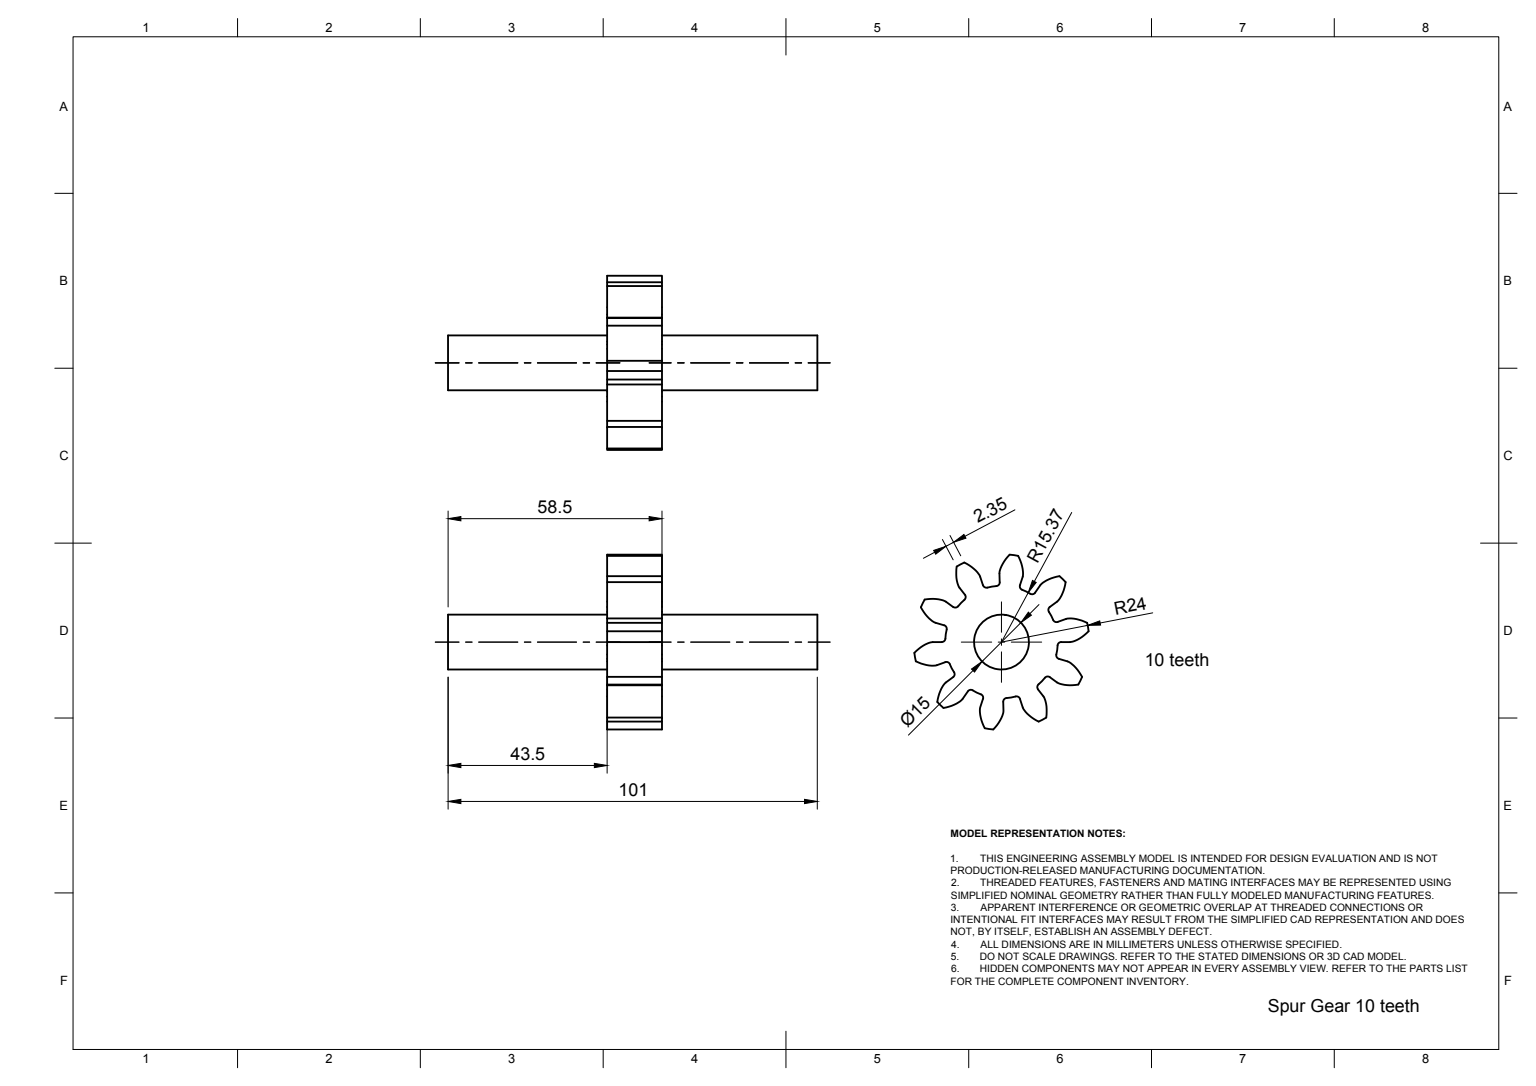
ISO-10303-21;
HEADER;
/* Generated by software containing ST-Developer
 * from STEP Tools, Inc. (www.steptools.com) 
 */

FILE_DESCRIPTION(
/* description */ (''),
/* implementation_level */ '2;1');

FILE_NAME(
/* name */ 'Spur Gear 10 teeth.step',
/* time_stamp */ '2026-10-05T21:54:13-07:00',
/* author */ (''),
/* organization */ (''),
/* preprocessor_version */ 'ST-DEVELOPER v20.2',
/* originating_system */ 'Autodesk Translation Framework v15.15.0.0',
/* authorisation */ '');

FILE_SCHEMA (('AUTOMOTIVE_DESIGN { 1 0 10303 214 3 1 1 }'));
ENDSEC;

DATA;
#10=MECHANICAL_DESIGN_GEOMETRIC_PRESENTATION_REPRESENTATION('',(#192),#43781);
#176=SHAPE_REPRESENTATION_RELATIONSHIP('SRR','None',#43814,#184);
#184=ADVANCED_BREP_SHAPE_REPRESENTATION('',(#236),#43774);
#192=STYLED_ITEM('',(#43862),#236);
#236=MANIFOLD_SOLID_BREP('Body1',#13052);
#281=FACE_BOUND('',#2275,.T.);
#282=FACE_BOUND('',#2277,.T.);
#571=B_SPLINE_CURVE_WITH_KNOTS('',5,(#32053,#32054,#32055,#32056,#32057,
#32058,#32059,#32060,#32061,#32062,#32063,#32064,#32065,#32066,#32067,#32068,
#32069,#32070,#32071,#32072,#32073,#32074,#32075,#32076,#32077,#32078,#32079,
#32080,#32081,#32082,#32083,#32084,#32085,#32086,#32087,#32088,#32089,#32090,
#32091,#32092,#32093,#32094,#32095,#32096,#32097,#32098,#32099,#32100,#32101,
#32102,#32103,#32104,#32105,#32106,#32107,#32108,#32109,#32110,#32111,#32112,
#32113,#32114,#32115,#32116,#32117,#32118,#32119,#32120,#32121,#32122,#32123,
#32124,#32125,#32126),.UNSPECIFIED.,.F.,.F.,(6,1,1,1,1,1,1,1,1,1,1,1,1,
1,1,1,1,1,1,1,1,1,1,1,1,1,1,1,1,1,1,1,1,1,1,1,1,1,1,1,1,1,1,1,1,1,1,1,1,
1,1,1,1,1,1,1,1,1,1,1,1,1,1,1,1,1,1,1,1,6),(0.,0.0142857142857143,0.0285714285714286,
0.0428571428571429,0.0571428571428571,0.0714285714285714,0.0857142857142857,
0.1,0.114285714285714,0.128571428571429,0.142857142857143,0.157142857142857,
0.171428571428571,0.185714285714286,0.2,0.214285714285714,0.228571428571429,
0.242857142857143,0.257142857142857,0.271428571428571,0.285714285714286,
0.3,0.314285714285714,0.328571428571429,0.342857142857143,0.357142857142857,
0.371428571428571,0.385714285714286,0.4,0.414285714285714,0.428571428571429,
0.442857142857143,0.457142857142857,0.471428571428572,0.485714285714286,
0.5,0.514285714285714,0.528571428571429,0.542857142857143,0.557142857142857,
0.571428571428571,0.585714285714286,0.6,0.614285714285714,0.628571428571428,
0.642857142857142,0.657142857142857,0.671428571428571,0.685714285714285,
0.699999999999999,0.714285714285714,0.728571428571428,0.742857142857142,
0.757142857142856,0.771428571428571,0.785714285714285,0.799999999999999,
0.814285714285713,0.828571428571428,0.842857142857142,0.857142857142856,
0.87142857142857,0.885714285714284,0.899999999999999,0.914285714285713,
0.928571428571427,0.942857142857141,0.957142857142856,0.97142857142857,
1.),.UNSPECIFIED.);
#572=B_SPLINE_CURVE_WITH_KNOTS('',5,(#32128,#32129,#32130,#32131,#32132,
#32133,#32134,#32135,#32136,#32137,#32138,#32139,#32140,#32141,#32142,#32143,
#32144,#32145,#32146,#32147,#32148,#32149,#32150,#32151,#32152,#32153,#32154,
#32155,#32156,#32157,#32158,#32159,#32160,#32161,#32162,#32163,#32164,#32165,
#32166,#32167,#32168,#32169,#32170,#32171,#32172,#32173,#32174,#32175,#32176,
#32177,#32178,#32179,#32180,#32181,#32182,#32183,#32184,#32185,#32186,#32187,
#32188,#32189,#32190,#32191,#32192,#32193,#32194,#32195,#32196,#32197,#32198,
#32199,#32200,#32201,#32202),.UNSPECIFIED.,.F.,.F.,(6,1,1,1,1,1,1,1,1,1,
1,1,1,1,1,1,1,1,1,1,1,1,1,1,1,1,1,1,1,1,1,1,1,1,1,1,1,1,1,1,1,1,1,1,1,1,
1,1,1,1,1,1,1,1,1,1,1,1,1,1,1,1,1,1,1,1,1,1,1,1,6),(-1.,-0.985714285714284,
-0.97142857142857,-0.957142857142856,-0.942857142857141,-0.928571428571427,
-0.914285714285713,-0.899999999999999,-0.885714285714284,-0.87142857142857,
-0.857142857142856,-0.842857142857142,-0.828571428571428,-0.814285714285713,
-0.799999999999999,-0.785714285714285,-0.771428571428571,-0.757142857142856,
-0.742857142857142,-0.728571428571428,-0.714285714285714,-0.699999999999999,
-0.685714285714285,-0.671428571428571,-0.657142857142857,-0.642857142857142,
-0.628571428571428,-0.614285714285714,-0.6,-0.585714285714286,-0.571428571428571,
-0.557142857142857,-0.542857142857143,-0.528571428571429,-0.514285714285714,
-0.5,-0.485714285714286,-0.471428571428572,-0.457142857142857,-0.442857142857143,
-0.428571428571429,-0.414285714285714,-0.4,-0.385714285714286,-0.371428571428571,
-0.357142857142857,-0.342857142857143,-0.328571428571429,-0.314285714285714,
-0.3,-0.285714285714286,-0.271428571428571,-0.257142857142857,-0.242857142857143,
-0.228571428571429,-0.214285714285714,-0.2,-0.185714285714286,-0.171428571428571,
-0.157142857142857,-0.142857142857143,-0.128571428571429,-0.114285714285714,
-0.1,-0.0857142857142857,-0.0714285714285714,-0.0571428571428571,-0.0428571428571429,
-0.0285714285714286,-0.0142857142857143,0.),.UNSPECIFIED.);
#573=B_SPLINE_CURVE_WITH_KNOTS('',5,(#32360,#32361,#32362,#32363,#32364,
#32365,#32366,#32367,#32368,#32369,#32370,#32371,#32372,#32373,#32374,#32375,
#32376,#32377,#32378,#32379,#32380,#32381,#32382,#32383,#32384,#32385,#32386,
#32387,#32388,#32389,#32390,#32391,#32392,#32393,#32394,#32395,#32396,#32397,
#32398,#32399,#32400,#32401,#32402,#32403,#32404,#32405,#32406,#32407,#32408,
#32409,#32410,#32411,#32412,#32413,#32414,#32415,#32416,#32417,#32418,#32419,
#32420,#32421,#32422,#32423,#32424,#32425,#32426,#32427,#32428,#32429,#32430,
#32431,#32432,#32433),.UNSPECIFIED.,.F.,.F.,(6,1,1,1,1,1,1,1,1,1,1,1,1,
1,1,1,1,1,1,1,1,1,1,1,1,1,1,1,1,1,1,1,1,1,1,1,1,1,1,1,1,1,1,1,1,1,1,1,1,
1,1,1,1,1,1,1,1,1,1,1,1,1,1,1,1,1,1,1,1,6),(0.,0.0142857142857143,0.0285714285714286,
0.0428571428571429,0.0571428571428571,0.0714285714285714,0.0857142857142857,
0.1,0.114285714285714,0.128571428571429,0.142857142857143,0.157142857142857,
0.171428571428571,0.185714285714286,0.2,0.214285714285714,0.228571428571429,
0.242857142857143,0.257142857142857,0.271428571428571,0.285714285714286,
0.3,0.314285714285714,0.328571428571429,0.342857142857143,0.357142857142857,
0.371428571428571,0.385714285714286,0.4,0.414285714285714,0.428571428571429,
0.442857142857143,0.457142857142857,0.471428571428572,0.485714285714286,
0.5,0.514285714285714,0.528571428571429,0.542857142857143,0.557142857142857,
0.571428571428571,0.585714285714286,0.6,0.614285714285714,0.628571428571428,
0.642857142857142,0.657142857142857,0.671428571428571,0.685714285714285,
0.699999999999999,0.714285714285714,0.728571428571428,0.742857142857142,
0.757142857142856,0.771428571428571,0.785714285714285,0.799999999999999,
0.814285714285713,0.828571428571428,0.842857142857142,0.857142857142856,
0.87142857142857,0.885714285714284,0.899999999999999,0.914285714285713,
0.928571428571427,0.942857142857141,0.957142857142856,0.97142857142857,
1.),.UNSPECIFIED.);
#574=B_SPLINE_CURVE_WITH_KNOTS('',5,(#32434,#32435,#32436,#32437,#32438,
#32439,#32440,#32441,#32442,#32443,#32444,#32445,#32446,#32447,#32448,#32449,
#32450,#32451,#32452,#32453,#32454,#32455,#32456,#32457,#32458,#32459,#32460,
#32461,#32462,#32463,#32464,#32465,#32466,#32467,#32468,#32469,#32470,#32471,
#32472,#32473,#32474,#32475,#32476,#32477,#32478,#32479,#32480,#32481,#32482,
#32483,#32484,#32485,#32486,#32487,#32488,#32489,#32490,#32491,#32492,#32493,
#32494,#32495,#32496,#32497,#32498,#32499,#32500,#32501,#32502,#32503,#32504,
#32505,#32506,#32507),.UNSPECIFIED.,.F.,.F.,(6,1,1,1,1,1,1,1,1,1,1,1,1,
1,1,1,1,1,1,1,1,1,1,1,1,1,1,1,1,1,1,1,1,1,1,1,1,1,1,1,1,1,1,1,1,1,1,1,1,
1,1,1,1,1,1,1,1,1,1,1,1,1,1,1,1,1,1,1,1,6),(0.,0.0142857142857143,0.0285714285714286,
0.0428571428571429,0.0571428571428571,0.0714285714285714,0.0857142857142857,
0.1,0.114285714285714,0.128571428571429,0.142857142857143,0.157142857142857,
0.171428571428571,0.185714285714286,0.2,0.214285714285714,0.228571428571429,
0.242857142857143,0.257142857142857,0.271428571428571,0.285714285714286,
0.3,0.314285714285714,0.328571428571429,0.342857142857143,0.357142857142857,
0.371428571428571,0.385714285714286,0.4,0.414285714285714,0.428571428571429,
0.442857142857143,0.457142857142857,0.471428571428572,0.485714285714286,
0.5,0.514285714285714,0.528571428571429,0.542857142857143,0.557142857142857,
0.571428571428571,0.585714285714286,0.6,0.614285714285714,0.628571428571428,
0.642857142857142,0.657142857142857,0.671428571428571,0.685714285714285,
0.699999999999999,0.714285714285714,0.728571428571428,0.742857142857142,
0.757142857142856,0.771428571428571,0.785714285714285,0.799999999999999,
0.814285714285713,0.828571428571428,0.842857142857142,0.857142857142856,
0.87142857142857,0.885714285714284,0.899999999999999,0.914285714285713,
0.928571428571427,0.942857142857141,0.957142857142856,0.97142857142857,
1.),.UNSPECIFIED.);
#575=B_SPLINE_CURVE_WITH_KNOTS('',5,(#32659,#32660,#32661,#32662,#32663,
#32664,#32665,#32666,#32667,#32668,#32669,#32670,#32671,#32672,#32673,#32674,
#32675,#32676,#32677,#32678,#32679,#32680,#32681,#32682,#32683,#32684,#32685,
#32686,#32687,#32688,#32689,#32690,#32691,#32692,#32693,#32694,#32695,#32696,
#32697,#32698,#32699,#32700,#32701,#32702,#32703,#32704,#32705,#32706,#32707,
#32708,#32709,#32710,#32711,#32712,#32713,#32714,#32715,#32716,#32717,#32718,
#32719,#32720,#32721,#32722,#32723,#32724,#32725,#32726,#32727,#32728,#32729,
#32730,#32731,#32732),.UNSPECIFIED.,.F.,.F.,(6,1,1,1,1,1,1,1,1,1,1,1,1,
1,1,1,1,1,1,1,1,1,1,1,1,1,1,1,1,1,1,1,1,1,1,1,1,1,1,1,1,1,1,1,1,1,1,1,1,
1,1,1,1,1,1,1,1,1,1,1,1,1,1,1,1,1,1,1,1,6),(0.,0.0142857142857143,0.0285714285714286,
0.0428571428571429,0.0571428571428571,0.0714285714285714,0.0857142857142857,
0.1,0.114285714285714,0.128571428571429,0.142857142857143,0.157142857142857,
0.171428571428571,0.185714285714286,0.2,0.214285714285714,0.228571428571429,
0.242857142857143,0.257142857142857,0.271428571428571,0.285714285714286,
0.3,0.314285714285714,0.328571428571429,0.342857142857143,0.357142857142857,
0.371428571428571,0.385714285714286,0.4,0.414285714285714,0.428571428571429,
0.442857142857143,0.457142857142857,0.471428571428572,0.485714285714286,
0.5,0.514285714285714,0.528571428571429,0.542857142857143,0.557142857142857,
0.571428571428571,0.585714285714286,0.6,0.614285714285714,0.628571428571428,
0.642857142857142,0.657142857142857,0.671428571428571,0.685714285714285,
0.699999999999999,0.714285714285714,0.728571428571428,0.742857142857142,
0.757142857142856,0.771428571428571,0.785714285714285,0.799999999999999,
0.814285714285713,0.828571428571428,0.842857142857142,0.857142857142856,
0.87142857142857,0.885714285714284,0.899999999999999,0.914285714285713,
0.928571428571427,0.942857142857141,0.957142857142856,0.97142857142857,
1.),.UNSPECIFIED.);
#576=B_SPLINE_CURVE_WITH_KNOTS('',5,(#32734,#32735,#32736,#32737,#32738,
#32739,#32740,#32741,#32742,#32743,#32744,#32745,#32746,#32747,#32748,#32749,
#32750,#32751,#32752,#32753,#32754,#32755,#32756,#32757,#32758,#32759,#32760,
#32761,#32762,#32763,#32764,#32765,#32766,#32767,#32768,#32769,#32770,#32771,
#32772,#32773,#32774,#32775,#32776,#32777,#32778,#32779,#32780,#32781,#32782,
#32783,#32784,#32785,#32786,#32787,#32788,#32789,#32790,#32791,#32792,#32793,
#32794,#32795,#32796,#32797,#32798,#32799,#32800,#32801,#32802,#32803,#32804,
#32805,#32806,#32807,#32808),.UNSPECIFIED.,.F.,.F.,(6,1,1,1,1,1,1,1,1,1,
1,1,1,1,1,1,1,1,1,1,1,1,1,1,1,1,1,1,1,1,1,1,1,1,1,1,1,1,1,1,1,1,1,1,1,1,
1,1,1,1,1,1,1,1,1,1,1,1,1,1,1,1,1,1,1,1,1,1,1,1,6),(-1.,-0.985714285714284,
-0.97142857142857,-0.957142857142856,-0.942857142857141,-0.928571428571427,
-0.914285714285713,-0.899999999999999,-0.885714285714284,-0.87142857142857,
-0.857142857142856,-0.842857142857142,-0.828571428571428,-0.814285714285713,
-0.799999999999999,-0.785714285714285,-0.771428571428571,-0.757142857142856,
-0.742857142857142,-0.728571428571428,-0.714285714285714,-0.699999999999999,
-0.685714285714285,-0.671428571428571,-0.657142857142857,-0.642857142857142,
-0.628571428571428,-0.614285714285714,-0.6,-0.585714285714286,-0.571428571428571,
-0.557142857142857,-0.542857142857143,-0.528571428571429,-0.514285714285714,
-0.5,-0.485714285714286,-0.471428571428572,-0.457142857142857,-0.442857142857143,
-0.428571428571429,-0.414285714285714,-0.4,-0.385714285714286,-0.371428571428571,
-0.357142857142857,-0.342857142857143,-0.328571428571429,-0.314285714285714,
-0.3,-0.285714285714286,-0.271428571428571,-0.257142857142857,-0.242857142857143,
-0.228571428571429,-0.214285714285714,-0.2,-0.185714285714286,-0.171428571428571,
-0.157142857142857,-0.142857142857143,-0.128571428571429,-0.114285714285714,
-0.1,-0.0857142857142857,-0.0714285714285714,-0.0571428571428571,-0.0428571428571429,
-0.0285714285714286,-0.0142857142857143,0.),.UNSPECIFIED.);
#577=B_SPLINE_CURVE_WITH_KNOTS('',5,(#32966,#32967,#32968,#32969,#32970,
#32971,#32972,#32973,#32974,#32975,#32976,#32977,#32978,#32979,#32980,#32981,
#32982,#32983,#32984,#32985,#32986,#32987,#32988,#32989,#32990,#32991,#32992,
#32993,#32994,#32995,#32996,#32997,#32998,#32999,#33000,#33001,#33002,#33003,
#33004,#33005,#33006,#33007,#33008,#33009,#33010,#33011,#33012,#33013,#33014,
#33015,#33016,#33017,#33018,#33019,#33020,#33021,#33022,#33023,#33024,#33025,
#33026,#33027,#33028,#33029,#33030,#33031,#33032,#33033,#33034,#33035,#33036,
#33037,#33038,#33039),.UNSPECIFIED.,.F.,.F.,(6,1,1,1,1,1,1,1,1,1,1,1,1,
1,1,1,1,1,1,1,1,1,1,1,1,1,1,1,1,1,1,1,1,1,1,1,1,1,1,1,1,1,1,1,1,1,1,1,1,
1,1,1,1,1,1,1,1,1,1,1,1,1,1,1,1,1,1,1,1,6),(0.,0.0142857142857143,0.0285714285714286,
0.0428571428571429,0.0571428571428571,0.0714285714285714,0.0857142857142857,
0.1,0.114285714285714,0.128571428571429,0.142857142857143,0.157142857142857,
0.171428571428571,0.185714285714286,0.2,0.214285714285714,0.228571428571429,
0.242857142857143,0.257142857142857,0.271428571428571,0.285714285714286,
0.3,0.314285714285714,0.328571428571429,0.342857142857143,0.357142857142857,
0.371428571428571,0.385714285714286,0.4,0.414285714285714,0.428571428571429,
0.442857142857143,0.457142857142857,0.471428571428572,0.485714285714286,
0.5,0.514285714285714,0.528571428571429,0.542857142857143,0.557142857142857,
0.571428571428571,0.585714285714286,0.6,0.614285714285714,0.628571428571428,
0.642857142857142,0.657142857142857,0.671428571428571,0.685714285714285,
0.699999999999999,0.714285714285714,0.728571428571428,0.742857142857142,
0.757142857142856,0.771428571428571,0.785714285714285,0.799999999999999,
0.814285714285713,0.828571428571428,0.842857142857142,0.857142857142856,
0.87142857142857,0.885714285714284,0.899999999999999,0.914285714285713,
0.928571428571427,0.942857142857141,0.957142857142856,0.97142857142857,
1.),.UNSPECIFIED.);
#578=B_SPLINE_CURVE_WITH_KNOTS('',5,(#33040,#33041,#33042,#33043,#33044,
#33045,#33046,#33047,#33048,#33049,#33050,#33051,#33052,#33053,#33054,#33055,
#33056,#33057,#33058,#33059,#33060,#33061,#33062,#33063,#33064,#33065,#33066,
#33067,#33068,#33069,#33070,#33071,#33072,#33073,#33074,#33075,#33076,#33077,
#33078,#33079,#33080,#33081,#33082,#33083,#33084,#33085,#33086,#33087,#33088,
#33089,#33090,#33091,#33092,#33093,#33094,#33095,#33096,#33097,#33098,#33099,
#33100,#33101,#33102,#33103,#33104,#33105,#33106,#33107,#33108,#33109,#33110,
#33111,#33112,#33113),.UNSPECIFIED.,.F.,.F.,(6,1,1,1,1,1,1,1,1,1,1,1,1,
1,1,1,1,1,1,1,1,1,1,1,1,1,1,1,1,1,1,1,1,1,1,1,1,1,1,1,1,1,1,1,1,1,1,1,1,
1,1,1,1,1,1,1,1,1,1,1,1,1,1,1,1,1,1,1,1,6),(0.,0.0142857142857143,0.0285714285714286,
0.0428571428571429,0.0571428571428571,0.0714285714285714,0.0857142857142857,
0.1,0.114285714285714,0.128571428571429,0.142857142857143,0.157142857142857,
0.171428571428571,0.185714285714286,0.2,0.214285714285714,0.228571428571429,
0.242857142857143,0.257142857142857,0.271428571428571,0.285714285714286,
0.3,0.314285714285714,0.328571428571429,0.342857142857143,0.357142857142857,
0.371428571428571,0.385714285714286,0.4,0.414285714285714,0.428571428571429,
0.442857142857143,0.457142857142857,0.471428571428572,0.485714285714286,
0.5,0.514285714285714,0.528571428571429,0.542857142857143,0.557142857142857,
0.571428571428571,0.585714285714286,0.6,0.614285714285714,0.628571428571428,
0.642857142857142,0.657142857142857,0.671428571428571,0.685714285714285,
0.699999999999999,0.714285714285714,0.728571428571428,0.742857142857142,
0.757142857142856,0.771428571428571,0.785714285714285,0.799999999999999,
0.814285714285713,0.828571428571428,0.842857142857142,0.857142857142856,
0.87142857142857,0.885714285714284,0.899999999999999,0.914285714285713,
0.928571428571427,0.942857142857141,0.957142857142856,0.97142857142857,
1.),.UNSPECIFIED.);
#579=B_SPLINE_CURVE_WITH_KNOTS('',5,(#33265,#33266,#33267,#33268,#33269,
#33270,#33271,#33272,#33273,#33274,#33275,#33276,#33277,#33278,#33279,#33280,
#33281,#33282,#33283,#33284,#33285,#33286,#33287,#33288,#33289,#33290,#33291,
#33292,#33293,#33294,#33295,#33296,#33297,#33298,#33299,#33300,#33301,#33302,
#33303,#33304,#33305,#33306,#33307,#33308,#33309,#33310,#33311,#33312,#33313,
#33314,#33315,#33316,#33317,#33318,#33319,#33320,#33321,#33322,#33323,#33324,
#33325,#33326,#33327,#33328,#33329,#33330,#33331,#33332,#33333,#33334,#33335,
#33336,#33337,#33338),.UNSPECIFIED.,.F.,.F.,(6,1,1,1,1,1,1,1,1,1,1,1,1,
1,1,1,1,1,1,1,1,1,1,1,1,1,1,1,1,1,1,1,1,1,1,1,1,1,1,1,1,1,1,1,1,1,1,1,1,
1,1,1,1,1,1,1,1,1,1,1,1,1,1,1,1,1,1,1,1,6),(0.,0.0142857142857143,0.0285714285714286,
0.0428571428571429,0.0571428571428571,0.0714285714285714,0.0857142857142857,
0.1,0.114285714285714,0.128571428571429,0.142857142857143,0.157142857142857,
0.171428571428571,0.185714285714286,0.2,0.214285714285714,0.228571428571429,
0.242857142857143,0.257142857142857,0.271428571428571,0.285714285714286,
0.3,0.314285714285714,0.328571428571429,0.342857142857143,0.357142857142857,
0.371428571428571,0.385714285714286,0.4,0.414285714285714,0.428571428571429,
0.442857142857143,0.457142857142857,0.471428571428572,0.485714285714286,
0.5,0.514285714285714,0.528571428571429,0.542857142857143,0.557142857142857,
0.571428571428571,0.585714285714286,0.6,0.614285714285714,0.628571428571428,
0.642857142857142,0.657142857142857,0.671428571428571,0.685714285714285,
0.699999999999999,0.714285714285714,0.728571428571428,0.742857142857142,
0.757142857142856,0.771428571428571,0.785714285714285,0.799999999999999,
0.814285714285713,0.828571428571428,0.842857142857142,0.857142857142856,
0.87142857142857,0.885714285714284,0.899999999999999,0.914285714285713,
0.928571428571427,0.942857142857141,0.957142857142856,0.97142857142857,
1.),.UNSPECIFIED.);
#580=B_SPLINE_CURVE_WITH_KNOTS('',5,(#33340,#33341,#33342,#33343,#33344,
#33345,#33346,#33347,#33348,#33349,#33350,#33351,#33352,#33353,#33354,#33355,
#33356,#33357,#33358,#33359,#33360,#33361,#33362,#33363,#33364,#33365,#33366,
#33367,#33368,#33369,#33370,#33371,#33372,#33373,#33374,#33375,#33376,#33377,
#33378,#33379,#33380,#33381,#33382,#33383,#33384,#33385,#33386,#33387,#33388,
#33389,#33390,#33391,#33392,#33393,#33394,#33395,#33396,#33397,#33398,#33399,
#33400,#33401,#33402,#33403,#33404,#33405,#33406,#33407,#33408,#33409,#33410,
#33411,#33412,#33413,#33414),.UNSPECIFIED.,.F.,.F.,(6,1,1,1,1,1,1,1,1,1,
1,1,1,1,1,1,1,1,1,1,1,1,1,1,1,1,1,1,1,1,1,1,1,1,1,1,1,1,1,1,1,1,1,1,1,1,
1,1,1,1,1,1,1,1,1,1,1,1,1,1,1,1,1,1,1,1,1,1,1,1,6),(-1.,-0.985714285714284,
-0.97142857142857,-0.957142857142856,-0.942857142857141,-0.928571428571427,
-0.914285714285713,-0.899999999999999,-0.885714285714284,-0.87142857142857,
-0.857142857142856,-0.842857142857142,-0.828571428571428,-0.814285714285713,
-0.799999999999999,-0.785714285714285,-0.771428571428571,-0.757142857142856,
-0.742857142857142,-0.728571428571428,-0.714285714285714,-0.699999999999999,
-0.685714285714285,-0.671428571428571,-0.657142857142857,-0.642857142857142,
-0.628571428571428,-0.614285714285714,-0.6,-0.585714285714286,-0.571428571428571,
-0.557142857142857,-0.542857142857143,-0.528571428571429,-0.514285714285714,
-0.5,-0.485714285714286,-0.471428571428572,-0.457142857142857,-0.442857142857143,
-0.428571428571429,-0.414285714285714,-0.4,-0.385714285714286,-0.371428571428571,
-0.357142857142857,-0.342857142857143,-0.328571428571429,-0.314285714285714,
-0.3,-0.285714285714286,-0.271428571428571,-0.257142857142857,-0.242857142857143,
-0.228571428571429,-0.214285714285714,-0.2,-0.185714285714286,-0.171428571428571,
-0.157142857142857,-0.142857142857143,-0.128571428571429,-0.114285714285714,
-0.1,-0.0857142857142857,-0.0714285714285714,-0.0571428571428571,-0.0428571428571429,
-0.0285714285714286,-0.0142857142857143,0.),.UNSPECIFIED.);
#581=B_SPLINE_CURVE_WITH_KNOTS('',5,(#33572,#33573,#33574,#33575,#33576,
#33577,#33578,#33579,#33580,#33581,#33582,#33583,#33584,#33585,#33586,#33587,
#33588,#33589,#33590,#33591,#33592,#33593,#33594,#33595,#33596,#33597,#33598,
#33599,#33600,#33601,#33602,#33603,#33604,#33605,#33606,#33607,#33608,#33609,
#33610,#33611,#33612,#33613,#33614,#33615,#33616,#33617,#33618,#33619,#33620,
#33621,#33622,#33623,#33624,#33625,#33626,#33627,#33628,#33629,#33630,#33631,
#33632,#33633,#33634,#33635,#33636,#33637,#33638,#33639,#33640,#33641,#33642,
#33643,#33644,#33645),.UNSPECIFIED.,.F.,.F.,(6,1,1,1,1,1,1,1,1,1,1,1,1,
1,1,1,1,1,1,1,1,1,1,1,1,1,1,1,1,1,1,1,1,1,1,1,1,1,1,1,1,1,1,1,1,1,1,1,1,
1,1,1,1,1,1,1,1,1,1,1,1,1,1,1,1,1,1,1,1,6),(0.,0.0142857142857143,0.0285714285714286,
0.0428571428571429,0.0571428571428571,0.0714285714285714,0.0857142857142857,
0.1,0.114285714285714,0.128571428571429,0.142857142857143,0.157142857142857,
0.171428571428571,0.185714285714286,0.2,0.214285714285714,0.228571428571429,
0.242857142857143,0.257142857142857,0.271428571428571,0.285714285714286,
0.3,0.314285714285714,0.328571428571429,0.342857142857143,0.357142857142857,
0.371428571428571,0.385714285714286,0.4,0.414285714285714,0.428571428571429,
0.442857142857143,0.457142857142857,0.471428571428572,0.485714285714286,
0.5,0.514285714285714,0.528571428571429,0.542857142857143,0.557142857142857,
0.571428571428571,0.585714285714286,0.6,0.614285714285714,0.628571428571428,
0.642857142857142,0.657142857142857,0.671428571428571,0.685714285714285,
0.699999999999999,0.714285714285714,0.728571428571428,0.742857142857142,
0.757142857142856,0.771428571428571,0.785714285714285,0.799999999999999,
0.814285714285713,0.828571428571428,0.842857142857142,0.857142857142856,
0.87142857142857,0.885714285714284,0.899999999999999,0.914285714285713,
0.928571428571427,0.942857142857141,0.957142857142856,0.97142857142857,
1.),.UNSPECIFIED.);
#582=B_SPLINE_CURVE_WITH_KNOTS('',5,(#33646,#33647,#33648,#33649,#33650,
#33651,#33652,#33653,#33654,#33655,#33656,#33657,#33658,#33659,#33660,#33661,
#33662,#33663,#33664,#33665,#33666,#33667,#33668,#33669,#33670,#33671,#33672,
#33673,#33674,#33675,#33676,#33677,#33678,#33679,#33680,#33681,#33682,#33683,
#33684,#33685,#33686,#33687,#33688,#33689,#33690,#33691,#33692,#33693,#33694,
#33695,#33696,#33697,#33698,#33699,#33700,#33701,#33702,#33703,#33704,#33705,
#33706,#33707,#33708,#33709,#33710,#33711,#33712,#33713,#33714,#33715,#33716,
#33717,#33718,#33719),.UNSPECIFIED.,.F.,.F.,(6,1,1,1,1,1,1,1,1,1,1,1,1,
1,1,1,1,1,1,1,1,1,1,1,1,1,1,1,1,1,1,1,1,1,1,1,1,1,1,1,1,1,1,1,1,1,1,1,1,
1,1,1,1,1,1,1,1,1,1,1,1,1,1,1,1,1,1,1,1,6),(0.,0.0142857142857143,0.0285714285714286,
0.0428571428571429,0.0571428571428571,0.0714285714285714,0.0857142857142857,
0.1,0.114285714285714,0.128571428571429,0.142857142857143,0.157142857142857,
0.171428571428571,0.185714285714286,0.2,0.214285714285714,0.228571428571429,
0.242857142857143,0.257142857142857,0.271428571428571,0.285714285714286,
0.3,0.314285714285714,0.328571428571429,0.342857142857143,0.357142857142857,
0.371428571428571,0.385714285714286,0.4,0.414285714285714,0.428571428571429,
0.442857142857143,0.457142857142857,0.471428571428572,0.485714285714286,
0.5,0.514285714285714,0.528571428571429,0.542857142857143,0.557142857142857,
0.571428571428571,0.585714285714286,0.6,0.614285714285714,0.628571428571428,
0.642857142857142,0.657142857142857,0.671428571428571,0.685714285714285,
0.699999999999999,0.714285714285714,0.728571428571428,0.742857142857142,
0.757142857142856,0.771428571428571,0.785714285714285,0.799999999999999,
0.814285714285713,0.828571428571428,0.842857142857142,0.857142857142856,
0.87142857142857,0.885714285714284,0.899999999999999,0.914285714285713,
0.928571428571427,0.942857142857141,0.957142857142856,0.97142857142857,
1.),.UNSPECIFIED.);
#583=B_SPLINE_CURVE_WITH_KNOTS('',5,(#33871,#33872,#33873,#33874,#33875,
#33876,#33877,#33878,#33879,#33880,#33881,#33882,#33883,#33884,#33885,#33886,
#33887,#33888,#33889,#33890,#33891,#33892,#33893,#33894,#33895,#33896,#33897,
#33898,#33899,#33900,#33901,#33902,#33903,#33904,#33905,#33906,#33907,#33908,
#33909,#33910,#33911,#33912,#33913,#33914,#33915,#33916,#33917,#33918,#33919,
#33920,#33921,#33922,#33923,#33924,#33925,#33926,#33927,#33928,#33929,#33930,
#33931,#33932,#33933,#33934,#33935,#33936,#33937,#33938,#33939,#33940,#33941,
#33942,#33943,#33944),.UNSPECIFIED.,.F.,.F.,(6,1,1,1,1,1,1,1,1,1,1,1,1,
1,1,1,1,1,1,1,1,1,1,1,1,1,1,1,1,1,1,1,1,1,1,1,1,1,1,1,1,1,1,1,1,1,1,1,1,
1,1,1,1,1,1,1,1,1,1,1,1,1,1,1,1,1,1,1,1,6),(0.,0.0142857142857143,0.0285714285714286,
0.0428571428571429,0.0571428571428571,0.0714285714285714,0.0857142857142857,
0.1,0.114285714285714,0.128571428571429,0.142857142857143,0.157142857142857,
0.171428571428571,0.185714285714286,0.2,0.214285714285714,0.228571428571429,
0.242857142857143,0.257142857142857,0.271428571428571,0.285714285714286,
0.3,0.314285714285714,0.328571428571429,0.342857142857143,0.357142857142857,
0.371428571428571,0.385714285714286,0.4,0.414285714285714,0.428571428571429,
0.442857142857143,0.457142857142857,0.471428571428572,0.485714285714286,
0.5,0.514285714285714,0.528571428571429,0.542857142857143,0.557142857142857,
0.571428571428571,0.585714285714286,0.6,0.614285714285714,0.628571428571428,
0.642857142857142,0.657142857142857,0.671428571428571,0.685714285714285,
0.699999999999999,0.714285714285714,0.728571428571428,0.742857142857142,
0.757142857142856,0.771428571428571,0.785714285714285,0.799999999999999,
0.814285714285713,0.828571428571428,0.842857142857142,0.857142857142856,
0.87142857142857,0.885714285714284,0.899999999999999,0.914285714285713,
0.928571428571427,0.942857142857141,0.957142857142856,0.97142857142857,
1.),.UNSPECIFIED.);
#584=B_SPLINE_CURVE_WITH_KNOTS('',5,(#33946,#33947,#33948,#33949,#33950,
#33951,#33952,#33953,#33954,#33955,#33956,#33957,#33958,#33959,#33960,#33961,
#33962,#33963,#33964,#33965,#33966,#33967,#33968,#33969,#33970,#33971,#33972,
#33973,#33974,#33975,#33976,#33977,#33978,#33979,#33980,#33981,#33982,#33983,
#33984,#33985,#33986,#33987,#33988,#33989,#33990,#33991,#33992,#33993,#33994,
#33995,#33996,#33997,#33998,#33999,#34000,#34001,#34002,#34003,#34004,#34005,
#34006,#34007,#34008,#34009,#34010,#34011,#34012,#34013,#34014,#34015,#34016,
#34017,#34018,#34019,#34020),.UNSPECIFIED.,.F.,.F.,(6,1,1,1,1,1,1,1,1,1,
1,1,1,1,1,1,1,1,1,1,1,1,1,1,1,1,1,1,1,1,1,1,1,1,1,1,1,1,1,1,1,1,1,1,1,1,
1,1,1,1,1,1,1,1,1,1,1,1,1,1,1,1,1,1,1,1,1,1,1,1,6),(-1.,-0.985714285714284,
-0.97142857142857,-0.957142857142856,-0.942857142857141,-0.928571428571427,
-0.914285714285713,-0.899999999999999,-0.885714285714284,-0.87142857142857,
-0.857142857142856,-0.842857142857142,-0.828571428571428,-0.814285714285713,
-0.799999999999999,-0.785714285714285,-0.771428571428571,-0.757142857142856,
-0.742857142857142,-0.728571428571428,-0.714285714285714,-0.699999999999999,
-0.685714285714285,-0.671428571428571,-0.657142857142857,-0.642857142857142,
-0.628571428571428,-0.614285714285714,-0.6,-0.585714285714286,-0.571428571428571,
-0.557142857142857,-0.542857142857143,-0.528571428571429,-0.514285714285714,
-0.5,-0.485714285714286,-0.471428571428572,-0.457142857142857,-0.442857142857143,
-0.428571428571429,-0.414285714285714,-0.4,-0.385714285714286,-0.371428571428571,
-0.357142857142857,-0.342857142857143,-0.328571428571429,-0.314285714285714,
-0.3,-0.285714285714286,-0.271428571428571,-0.257142857142857,-0.242857142857143,
-0.228571428571429,-0.214285714285714,-0.2,-0.185714285714286,-0.171428571428571,
-0.157142857142857,-0.142857142857143,-0.128571428571429,-0.114285714285714,
-0.1,-0.0857142857142857,-0.0714285714285714,-0.0571428571428571,-0.0428571428571429,
-0.0285714285714286,-0.0142857142857143,0.),.UNSPECIFIED.);
#585=B_SPLINE_CURVE_WITH_KNOTS('',5,(#34178,#34179,#34180,#34181,#34182,
#34183,#34184,#34185,#34186,#34187,#34188,#34189,#34190,#34191,#34192,#34193,
#34194,#34195,#34196,#34197,#34198,#34199,#34200,#34201,#34202,#34203,#34204,
#34205,#34206,#34207,#34208,#34209,#34210,#34211,#34212,#34213,#34214,#34215,
#34216,#34217,#34218,#34219,#34220,#34221,#34222,#34223,#34224,#34225,#34226,
#34227,#34228,#34229,#34230,#34231,#34232,#34233,#34234,#34235,#34236,#34237,
#34238,#34239,#34240,#34241,#34242,#34243,#34244,#34245,#34246,#34247,#34248,
#34249,#34250,#34251),.UNSPECIFIED.,.F.,.F.,(6,1,1,1,1,1,1,1,1,1,1,1,1,
1,1,1,1,1,1,1,1,1,1,1,1,1,1,1,1,1,1,1,1,1,1,1,1,1,1,1,1,1,1,1,1,1,1,1,1,
1,1,1,1,1,1,1,1,1,1,1,1,1,1,1,1,1,1,1,1,6),(0.,0.0142857142857143,0.0285714285714286,
0.0428571428571429,0.0571428571428571,0.0714285714285714,0.0857142857142857,
0.1,0.114285714285714,0.128571428571429,0.142857142857143,0.157142857142857,
0.171428571428571,0.185714285714286,0.2,0.214285714285714,0.228571428571429,
0.242857142857143,0.257142857142857,0.271428571428571,0.285714285714286,
0.3,0.314285714285714,0.328571428571429,0.342857142857143,0.357142857142857,
0.371428571428571,0.385714285714286,0.4,0.414285714285714,0.428571428571429,
0.442857142857143,0.457142857142857,0.471428571428572,0.485714285714286,
0.5,0.514285714285714,0.528571428571429,0.542857142857143,0.557142857142857,
0.571428571428571,0.585714285714286,0.6,0.614285714285714,0.628571428571428,
0.642857142857142,0.657142857142857,0.671428571428571,0.685714285714285,
0.699999999999999,0.714285714285714,0.728571428571428,0.742857142857142,
0.757142857142856,0.771428571428571,0.785714285714285,0.799999999999999,
0.814285714285713,0.828571428571428,0.842857142857142,0.857142857142856,
0.87142857142857,0.885714285714284,0.899999999999999,0.914285714285713,
0.928571428571427,0.942857142857141,0.957142857142856,0.97142857142857,
1.),.UNSPECIFIED.);
#586=B_SPLINE_CURVE_WITH_KNOTS('',5,(#34252,#34253,#34254,#34255,#34256,
#34257,#34258,#34259,#34260,#34261,#34262,#34263,#34264,#34265,#34266,#34267,
#34268,#34269,#34270,#34271,#34272,#34273,#34274,#34275,#34276,#34277,#34278,
#34279,#34280,#34281,#34282,#34283,#34284,#34285,#34286,#34287,#34288,#34289,
#34290,#34291,#34292,#34293,#34294,#34295,#34296,#34297,#34298,#34299,#34300,
#34301,#34302,#34303,#34304,#34305,#34306,#34307,#34308,#34309,#34310,#34311,
#34312,#34313,#34314,#34315,#34316,#34317,#34318,#34319,#34320,#34321,#34322,
#34323,#34324,#34325),.UNSPECIFIED.,.F.,.F.,(6,1,1,1,1,1,1,1,1,1,1,1,1,
1,1,1,1,1,1,1,1,1,1,1,1,1,1,1,1,1,1,1,1,1,1,1,1,1,1,1,1,1,1,1,1,1,1,1,1,
1,1,1,1,1,1,1,1,1,1,1,1,1,1,1,1,1,1,1,1,6),(0.,0.0142857142857143,0.0285714285714286,
0.0428571428571429,0.0571428571428571,0.0714285714285714,0.0857142857142857,
0.1,0.114285714285714,0.128571428571429,0.142857142857143,0.157142857142857,
0.171428571428571,0.185714285714286,0.2,0.214285714285714,0.228571428571429,
0.242857142857143,0.257142857142857,0.271428571428571,0.285714285714286,
0.3,0.314285714285714,0.328571428571429,0.342857142857143,0.357142857142857,
0.371428571428571,0.385714285714286,0.4,0.414285714285714,0.428571428571429,
0.442857142857143,0.457142857142857,0.471428571428572,0.485714285714286,
0.5,0.514285714285714,0.528571428571429,0.542857142857143,0.557142857142857,
0.571428571428571,0.585714285714286,0.6,0.614285714285714,0.628571428571428,
0.642857142857142,0.657142857142857,0.671428571428571,0.685714285714285,
0.699999999999999,0.714285714285714,0.728571428571428,0.742857142857142,
0.757142857142856,0.771428571428571,0.785714285714285,0.799999999999999,
0.814285714285713,0.828571428571428,0.842857142857142,0.857142857142856,
0.87142857142857,0.885714285714284,0.899999999999999,0.914285714285713,
0.928571428571427,0.942857142857141,0.957142857142856,0.97142857142857,
1.),.UNSPECIFIED.);
#587=B_SPLINE_CURVE_WITH_KNOTS('',5,(#34477,#34478,#34479,#34480,#34481,
#34482,#34483,#34484,#34485,#34486,#34487,#34488,#34489,#34490,#34491,#34492,
#34493,#34494,#34495,#34496,#34497,#34498,#34499,#34500,#34501,#34502,#34503,
#34504,#34505,#34506,#34507,#34508,#34509,#34510,#34511,#34512,#34513,#34514,
#34515,#34516,#34517,#34518,#34519,#34520,#34521,#34522,#34523,#34524,#34525,
#34526,#34527,#34528,#34529,#34530,#34531,#34532,#34533,#34534,#34535,#34536,
#34537,#34538,#34539,#34540,#34541,#34542,#34543,#34544,#34545,#34546,#34547,
#34548,#34549,#34550),.UNSPECIFIED.,.F.,.F.,(6,1,1,1,1,1,1,1,1,1,1,1,1,
1,1,1,1,1,1,1,1,1,1,1,1,1,1,1,1,1,1,1,1,1,1,1,1,1,1,1,1,1,1,1,1,1,1,1,1,
1,1,1,1,1,1,1,1,1,1,1,1,1,1,1,1,1,1,1,1,6),(0.,0.0142857142857143,0.0285714285714286,
0.0428571428571429,0.0571428571428571,0.0714285714285714,0.0857142857142857,
0.1,0.114285714285714,0.128571428571429,0.142857142857143,0.157142857142857,
0.171428571428571,0.185714285714286,0.2,0.214285714285714,0.228571428571429,
0.242857142857143,0.257142857142857,0.271428571428571,0.285714285714286,
0.3,0.314285714285714,0.328571428571429,0.342857142857143,0.357142857142857,
0.371428571428571,0.385714285714286,0.4,0.414285714285714,0.428571428571429,
0.442857142857143,0.457142857142857,0.471428571428572,0.485714285714286,
0.5,0.514285714285714,0.528571428571429,0.542857142857143,0.557142857142857,
0.571428571428571,0.585714285714286,0.6,0.614285714285714,0.628571428571428,
0.642857142857142,0.657142857142857,0.671428571428571,0.685714285714285,
0.699999999999999,0.714285714285714,0.728571428571428,0.742857142857142,
0.757142857142856,0.771428571428571,0.785714285714285,0.799999999999999,
0.814285714285713,0.828571428571428,0.842857142857142,0.857142857142856,
0.87142857142857,0.885714285714284,0.899999999999999,0.914285714285713,
0.928571428571427,0.942857142857141,0.957142857142856,0.97142857142857,
1.),.UNSPECIFIED.);
#588=B_SPLINE_CURVE_WITH_KNOTS('',5,(#34552,#34553,#34554,#34555,#34556,
#34557,#34558,#34559,#34560,#34561,#34562,#34563,#34564,#34565,#34566,#34567,
#34568,#34569,#34570,#34571,#34572,#34573,#34574,#34575,#34576,#34577,#34578,
#34579,#34580,#34581,#34582,#34583,#34584,#34585,#34586,#34587,#34588,#34589,
#34590,#34591,#34592,#34593,#34594,#34595,#34596,#34597,#34598,#34599,#34600,
#34601,#34602,#34603,#34604,#34605,#34606,#34607,#34608,#34609,#34610,#34611,
#34612,#34613,#34614,#34615,#34616,#34617,#34618,#34619,#34620,#34621,#34622,
#34623,#34624,#34625,#34626),.UNSPECIFIED.,.F.,.F.,(6,1,1,1,1,1,1,1,1,1,
1,1,1,1,1,1,1,1,1,1,1,1,1,1,1,1,1,1,1,1,1,1,1,1,1,1,1,1,1,1,1,1,1,1,1,1,
1,1,1,1,1,1,1,1,1,1,1,1,1,1,1,1,1,1,1,1,1,1,1,1,6),(-1.,-0.985714285714284,
-0.97142857142857,-0.957142857142856,-0.942857142857141,-0.928571428571427,
-0.914285714285713,-0.899999999999999,-0.885714285714284,-0.87142857142857,
-0.857142857142856,-0.842857142857142,-0.828571428571428,-0.814285714285713,
-0.799999999999999,-0.785714285714285,-0.771428571428571,-0.757142857142856,
-0.742857142857142,-0.728571428571428,-0.714285714285714,-0.699999999999999,
-0.685714285714285,-0.671428571428571,-0.657142857142857,-0.642857142857142,
-0.628571428571428,-0.614285714285714,-0.6,-0.585714285714286,-0.571428571428571,
-0.557142857142857,-0.542857142857143,-0.528571428571429,-0.514285714285714,
-0.5,-0.485714285714286,-0.471428571428572,-0.457142857142857,-0.442857142857143,
-0.428571428571429,-0.414285714285714,-0.4,-0.385714285714286,-0.371428571428571,
-0.357142857142857,-0.342857142857143,-0.328571428571429,-0.314285714285714,
-0.3,-0.285714285714286,-0.271428571428571,-0.257142857142857,-0.242857142857143,
-0.228571428571429,-0.214285714285714,-0.2,-0.185714285714286,-0.171428571428571,
-0.157142857142857,-0.142857142857143,-0.128571428571429,-0.114285714285714,
-0.1,-0.0857142857142857,-0.0714285714285714,-0.0571428571428571,-0.0428571428571429,
-0.0285714285714286,-0.0142857142857143,0.),.UNSPECIFIED.);
#589=B_SPLINE_CURVE_WITH_KNOTS('',5,(#34784,#34785,#34786,#34787,#34788,
#34789,#34790,#34791,#34792,#34793,#34794,#34795,#34796,#34797,#34798,#34799,
#34800,#34801,#34802,#34803,#34804,#34805,#34806,#34807,#34808,#34809,#34810,
#34811,#34812,#34813,#34814,#34815,#34816,#34817,#34818,#34819,#34820,#34821,
#34822,#34823,#34824,#34825,#34826,#34827,#34828,#34829,#34830,#34831,#34832,
#34833,#34834,#34835,#34836,#34837,#34838,#34839,#34840,#34841,#34842,#34843,
#34844,#34845,#34846,#34847,#34848,#34849,#34850,#34851,#34852,#34853,#34854,
#34855,#34856,#34857),.UNSPECIFIED.,.F.,.F.,(6,1,1,1,1,1,1,1,1,1,1,1,1,
1,1,1,1,1,1,1,1,1,1,1,1,1,1,1,1,1,1,1,1,1,1,1,1,1,1,1,1,1,1,1,1,1,1,1,1,
1,1,1,1,1,1,1,1,1,1,1,1,1,1,1,1,1,1,1,1,6),(0.,0.0142857142857143,0.0285714285714286,
0.0428571428571429,0.0571428571428571,0.0714285714285714,0.0857142857142857,
0.1,0.114285714285714,0.128571428571429,0.142857142857143,0.157142857142857,
0.171428571428571,0.185714285714286,0.2,0.214285714285714,0.228571428571429,
0.242857142857143,0.257142857142857,0.271428571428571,0.285714285714286,
0.3,0.314285714285714,0.328571428571429,0.342857142857143,0.357142857142857,
0.371428571428571,0.385714285714286,0.4,0.414285714285714,0.428571428571429,
0.442857142857143,0.457142857142857,0.471428571428572,0.485714285714286,
0.5,0.514285714285714,0.528571428571429,0.542857142857143,0.557142857142857,
0.571428571428571,0.585714285714286,0.6,0.614285714285714,0.628571428571428,
0.642857142857142,0.657142857142857,0.671428571428571,0.685714285714285,
0.699999999999999,0.714285714285714,0.728571428571428,0.742857142857142,
0.757142857142856,0.771428571428571,0.785714285714285,0.799999999999999,
0.814285714285713,0.828571428571428,0.842857142857142,0.857142857142856,
0.87142857142857,0.885714285714284,0.899999999999999,0.914285714285713,
0.928571428571427,0.942857142857141,0.957142857142856,0.97142857142857,
1.),.UNSPECIFIED.);
#590=B_SPLINE_CURVE_WITH_KNOTS('',5,(#34858,#34859,#34860,#34861,#34862,
#34863,#34864,#34865,#34866,#34867,#34868,#34869,#34870,#34871,#34872,#34873,
#34874,#34875,#34876,#34877,#34878,#34879,#34880,#34881,#34882,#34883,#34884,
#34885,#34886,#34887,#34888,#34889,#34890,#34891,#34892,#34893,#34894,#34895,
#34896,#34897,#34898,#34899,#34900,#34901,#34902,#34903,#34904,#34905,#34906,
#34907,#34908,#34909,#34910,#34911,#34912,#34913,#34914,#34915,#34916,#34917,
#34918,#34919,#34920,#34921,#34922,#34923,#34924,#34925,#34926,#34927,#34928,
#34929,#34930,#34931),.UNSPECIFIED.,.F.,.F.,(6,1,1,1,1,1,1,1,1,1,1,1,1,
1,1,1,1,1,1,1,1,1,1,1,1,1,1,1,1,1,1,1,1,1,1,1,1,1,1,1,1,1,1,1,1,1,1,1,1,
1,1,1,1,1,1,1,1,1,1,1,1,1,1,1,1,1,1,1,1,6),(0.,0.0142857142857143,0.0285714285714286,
0.0428571428571429,0.0571428571428571,0.0714285714285714,0.0857142857142857,
0.1,0.114285714285714,0.128571428571429,0.142857142857143,0.157142857142857,
0.171428571428571,0.185714285714286,0.2,0.214285714285714,0.228571428571429,
0.242857142857143,0.257142857142857,0.271428571428571,0.285714285714286,
0.3,0.314285714285714,0.328571428571429,0.342857142857143,0.357142857142857,
0.371428571428571,0.385714285714286,0.4,0.414285714285714,0.428571428571429,
0.442857142857143,0.457142857142857,0.471428571428572,0.485714285714286,
0.5,0.514285714285714,0.528571428571429,0.542857142857143,0.557142857142857,
0.571428571428571,0.585714285714286,0.6,0.614285714285714,0.628571428571428,
0.642857142857142,0.657142857142857,0.671428571428571,0.685714285714285,
0.699999999999999,0.714285714285714,0.728571428571428,0.742857142857142,
0.757142857142856,0.771428571428571,0.785714285714285,0.799999999999999,
0.814285714285713,0.828571428571428,0.842857142857142,0.857142857142856,
0.87142857142857,0.885714285714284,0.899999999999999,0.914285714285713,
0.928571428571427,0.942857142857141,0.957142857142856,0.97142857142857,
1.),.UNSPECIFIED.);
#591=B_SPLINE_CURVE_WITH_KNOTS('',5,(#35083,#35084,#35085,#35086,#35087,
#35088,#35089,#35090,#35091,#35092,#35093,#35094,#35095,#35096,#35097,#35098,
#35099,#35100,#35101,#35102,#35103,#35104,#35105,#35106,#35107,#35108,#35109,
#35110,#35111,#35112,#35113,#35114,#35115,#35116,#35117,#35118,#35119,#35120,
#35121,#35122,#35123,#35124,#35125,#35126,#35127,#35128,#35129,#35130,#35131,
#35132,#35133,#35134,#35135,#35136,#35137,#35138,#35139,#35140,#35141,#35142,
#35143,#35144,#35145,#35146,#35147,#35148,#35149,#35150,#35151,#35152,#35153,
#35154,#35155,#35156),.UNSPECIFIED.,.F.,.F.,(6,1,1,1,1,1,1,1,1,1,1,1,1,
1,1,1,1,1,1,1,1,1,1,1,1,1,1,1,1,1,1,1,1,1,1,1,1,1,1,1,1,1,1,1,1,1,1,1,1,
1,1,1,1,1,1,1,1,1,1,1,1,1,1,1,1,1,1,1,1,6),(0.,0.0142857142857143,0.0285714285714286,
0.0428571428571429,0.0571428571428571,0.0714285714285714,0.0857142857142857,
0.1,0.114285714285714,0.128571428571429,0.142857142857143,0.157142857142857,
0.171428571428571,0.185714285714286,0.2,0.214285714285714,0.228571428571429,
0.242857142857143,0.257142857142857,0.271428571428571,0.285714285714286,
0.3,0.314285714285714,0.328571428571429,0.342857142857143,0.357142857142857,
0.371428571428571,0.385714285714286,0.4,0.414285714285714,0.428571428571429,
0.442857142857143,0.457142857142857,0.471428571428572,0.485714285714286,
0.5,0.514285714285714,0.528571428571429,0.542857142857143,0.557142857142857,
0.571428571428571,0.585714285714286,0.6,0.614285714285714,0.628571428571428,
0.642857142857142,0.657142857142857,0.671428571428571,0.685714285714285,
0.699999999999999,0.714285714285714,0.728571428571428,0.742857142857142,
0.757142857142856,0.771428571428571,0.785714285714285,0.799999999999999,
0.814285714285713,0.828571428571428,0.842857142857142,0.857142857142856,
0.87142857142857,0.885714285714284,0.899999999999999,0.914285714285713,
0.928571428571427,0.942857142857141,0.957142857142856,0.97142857142857,
1.),.UNSPECIFIED.);
#592=B_SPLINE_CURVE_WITH_KNOTS('',5,(#35158,#35159,#35160,#35161,#35162,
#35163,#35164,#35165,#35166,#35167,#35168,#35169,#35170,#35171,#35172,#35173,
#35174,#35175,#35176,#35177,#35178,#35179,#35180,#35181,#35182,#35183,#35184,
#35185,#35186,#35187,#35188,#35189,#35190,#35191,#35192,#35193,#35194,#35195,
#35196,#35197,#35198,#35199,#35200,#35201,#35202,#35203,#35204,#35205,#35206,
#35207,#35208,#35209,#35210,#35211,#35212,#35213,#35214,#35215,#35216,#35217,
#35218,#35219,#35220,#35221,#35222,#35223,#35224,#35225,#35226,#35227,#35228,
#35229,#35230,#35231,#35232),.UNSPECIFIED.,.F.,.F.,(6,1,1,1,1,1,1,1,1,1,
1,1,1,1,1,1,1,1,1,1,1,1,1,1,1,1,1,1,1,1,1,1,1,1,1,1,1,1,1,1,1,1,1,1,1,1,
1,1,1,1,1,1,1,1,1,1,1,1,1,1,1,1,1,1,1,1,1,1,1,1,6),(-1.,-0.985714285714284,
-0.97142857142857,-0.957142857142856,-0.942857142857141,-0.928571428571427,
-0.914285714285713,-0.899999999999999,-0.885714285714284,-0.87142857142857,
-0.857142857142856,-0.842857142857142,-0.828571428571428,-0.814285714285713,
-0.799999999999999,-0.785714285714285,-0.771428571428571,-0.757142857142856,
-0.742857142857142,-0.728571428571428,-0.714285714285714,-0.699999999999999,
-0.685714285714285,-0.671428571428571,-0.657142857142857,-0.642857142857142,
-0.628571428571428,-0.614285714285714,-0.6,-0.585714285714286,-0.571428571428571,
-0.557142857142857,-0.542857142857143,-0.528571428571429,-0.514285714285714,
-0.5,-0.485714285714286,-0.471428571428572,-0.457142857142857,-0.442857142857143,
-0.428571428571429,-0.414285714285714,-0.4,-0.385714285714286,-0.371428571428571,
-0.357142857142857,-0.342857142857143,-0.328571428571429,-0.314285714285714,
-0.3,-0.285714285714286,-0.271428571428571,-0.257142857142857,-0.242857142857143,
-0.228571428571429,-0.214285714285714,-0.2,-0.185714285714286,-0.171428571428571,
-0.157142857142857,-0.142857142857143,-0.128571428571429,-0.114285714285714,
-0.1,-0.0857142857142857,-0.0714285714285714,-0.0571428571428571,-0.0428571428571429,
-0.0285714285714286,-0.0142857142857143,0.),.UNSPECIFIED.);
#593=B_SPLINE_CURVE_WITH_KNOTS('',5,(#35390,#35391,#35392,#35393,#35394,
#35395,#35396,#35397,#35398,#35399,#35400,#35401,#35402,#35403,#35404,#35405,
#35406,#35407,#35408,#35409,#35410,#35411,#35412,#35413,#35414,#35415,#35416,
#35417,#35418,#35419,#35420,#35421,#35422,#35423,#35424,#35425,#35426,#35427,
#35428,#35429,#35430,#35431,#35432,#35433,#35434,#35435,#35436,#35437,#35438,
#35439,#35440,#35441,#35442,#35443,#35444,#35445,#35446,#35447,#35448,#35449,
#35450,#35451,#35452,#35453,#35454,#35455,#35456,#35457,#35458,#35459,#35460,
#35461,#35462,#35463),.UNSPECIFIED.,.F.,.F.,(6,1,1,1,1,1,1,1,1,1,1,1,1,
1,1,1,1,1,1,1,1,1,1,1,1,1,1,1,1,1,1,1,1,1,1,1,1,1,1,1,1,1,1,1,1,1,1,1,1,
1,1,1,1,1,1,1,1,1,1,1,1,1,1,1,1,1,1,1,1,6),(0.,0.0142857142857143,0.0285714285714286,
0.0428571428571429,0.0571428571428571,0.0714285714285714,0.0857142857142857,
0.1,0.114285714285714,0.128571428571429,0.142857142857143,0.157142857142857,
0.171428571428571,0.185714285714286,0.2,0.214285714285714,0.228571428571429,
0.242857142857143,0.257142857142857,0.271428571428571,0.285714285714286,
0.3,0.314285714285714,0.328571428571429,0.342857142857143,0.357142857142857,
0.371428571428571,0.385714285714286,0.4,0.414285714285714,0.428571428571429,
0.442857142857143,0.457142857142857,0.471428571428572,0.485714285714286,
0.5,0.514285714285714,0.528571428571429,0.542857142857143,0.557142857142857,
0.571428571428571,0.585714285714286,0.6,0.614285714285714,0.628571428571428,
0.642857142857142,0.657142857142857,0.671428571428571,0.685714285714285,
0.699999999999999,0.714285714285714,0.728571428571428,0.742857142857142,
0.757142857142856,0.771428571428571,0.785714285714285,0.799999999999999,
0.814285714285713,0.828571428571428,0.842857142857142,0.857142857142856,
0.87142857142857,0.885714285714284,0.899999999999999,0.914285714285713,
0.928571428571427,0.942857142857141,0.957142857142856,0.97142857142857,
1.),.UNSPECIFIED.);
#594=B_SPLINE_CURVE_WITH_KNOTS('',5,(#35464,#35465,#35466,#35467,#35468,
#35469,#35470,#35471,#35472,#35473,#35474,#35475,#35476,#35477,#35478,#35479,
#35480,#35481,#35482,#35483,#35484,#35485,#35486,#35487,#35488,#35489,#35490,
#35491,#35492,#35493,#35494,#35495,#35496,#35497,#35498,#35499,#35500,#35501,
#35502,#35503,#35504,#35505,#35506,#35507,#35508,#35509,#35510,#35511,#35512,
#35513,#35514,#35515,#35516,#35517,#35518,#35519,#35520,#35521,#35522,#35523,
#35524,#35525,#35526,#35527,#35528,#35529,#35530,#35531,#35532,#35533,#35534,
#35535,#35536,#35537),.UNSPECIFIED.,.F.,.F.,(6,1,1,1,1,1,1,1,1,1,1,1,1,
1,1,1,1,1,1,1,1,1,1,1,1,1,1,1,1,1,1,1,1,1,1,1,1,1,1,1,1,1,1,1,1,1,1,1,1,
1,1,1,1,1,1,1,1,1,1,1,1,1,1,1,1,1,1,1,1,6),(0.,0.0142857142857143,0.0285714285714286,
0.0428571428571429,0.0571428571428571,0.0714285714285714,0.0857142857142857,
0.1,0.114285714285714,0.128571428571429,0.142857142857143,0.157142857142857,
0.171428571428571,0.185714285714286,0.2,0.214285714285714,0.228571428571429,
0.242857142857143,0.257142857142857,0.271428571428571,0.285714285714286,
0.3,0.314285714285714,0.328571428571429,0.342857142857143,0.357142857142857,
0.371428571428571,0.385714285714286,0.4,0.414285714285714,0.428571428571429,
0.442857142857143,0.457142857142857,0.471428571428572,0.485714285714286,
0.5,0.514285714285714,0.528571428571429,0.542857142857143,0.557142857142857,
0.571428571428571,0.585714285714286,0.6,0.614285714285714,0.628571428571428,
0.642857142857142,0.657142857142857,0.671428571428571,0.685714285714285,
0.699999999999999,0.714285714285714,0.728571428571428,0.742857142857142,
0.757142857142856,0.771428571428571,0.785714285714285,0.799999999999999,
0.814285714285713,0.828571428571428,0.842857142857142,0.857142857142856,
0.87142857142857,0.885714285714284,0.899999999999999,0.914285714285713,
0.928571428571427,0.942857142857141,0.957142857142856,0.97142857142857,
1.),.UNSPECIFIED.);
#595=B_SPLINE_CURVE_WITH_KNOTS('',5,(#35689,#35690,#35691,#35692,#35693,
#35694,#35695,#35696,#35697,#35698,#35699,#35700,#35701,#35702,#35703,#35704,
#35705,#35706,#35707,#35708,#35709,#35710,#35711,#35712,#35713,#35714,#35715,
#35716,#35717,#35718,#35719,#35720,#35721,#35722,#35723,#35724,#35725,#35726,
#35727,#35728,#35729,#35730,#35731,#35732,#35733,#35734,#35735,#35736,#35737,
#35738,#35739,#35740,#35741,#35742,#35743,#35744,#35745,#35746,#35747,#35748,
#35749,#35750,#35751,#35752,#35753,#35754,#35755,#35756,#35757,#35758,#35759,
#35760,#35761,#35762),.UNSPECIFIED.,.F.,.F.,(6,1,1,1,1,1,1,1,1,1,1,1,1,
1,1,1,1,1,1,1,1,1,1,1,1,1,1,1,1,1,1,1,1,1,1,1,1,1,1,1,1,1,1,1,1,1,1,1,1,
1,1,1,1,1,1,1,1,1,1,1,1,1,1,1,1,1,1,1,1,6),(0.,0.0142857142857143,0.0285714285714286,
0.0428571428571429,0.0571428571428571,0.0714285714285714,0.0857142857142857,
0.1,0.114285714285714,0.128571428571429,0.142857142857143,0.157142857142857,
0.171428571428571,0.185714285714286,0.2,0.214285714285714,0.228571428571429,
0.242857142857143,0.257142857142857,0.271428571428571,0.285714285714286,
0.3,0.314285714285714,0.328571428571429,0.342857142857143,0.357142857142857,
0.371428571428571,0.385714285714286,0.4,0.414285714285714,0.428571428571429,
0.442857142857143,0.457142857142857,0.471428571428572,0.485714285714286,
0.5,0.514285714285714,0.528571428571429,0.542857142857143,0.557142857142857,
0.571428571428571,0.585714285714286,0.6,0.614285714285714,0.628571428571428,
0.642857142857142,0.657142857142857,0.671428571428571,0.685714285714285,
0.699999999999999,0.714285714285714,0.728571428571428,0.742857142857142,
0.757142857142856,0.771428571428571,0.785714285714285,0.799999999999999,
0.814285714285713,0.828571428571428,0.842857142857142,0.857142857142856,
0.87142857142857,0.885714285714284,0.899999999999999,0.914285714285713,
0.928571428571427,0.942857142857141,0.957142857142856,0.97142857142857,
1.),.UNSPECIFIED.);
#596=B_SPLINE_CURVE_WITH_KNOTS('',5,(#35764,#35765,#35766,#35767,#35768,
#35769,#35770,#35771,#35772,#35773,#35774,#35775,#35776,#35777,#35778,#35779,
#35780,#35781,#35782,#35783,#35784,#35785,#35786,#35787,#35788,#35789,#35790,
#35791,#35792,#35793,#35794,#35795,#35796,#35797,#35798,#35799,#35800,#35801,
#35802,#35803,#35804,#35805,#35806,#35807,#35808,#35809,#35810,#35811,#35812,
#35813,#35814,#35815,#35816,#35817,#35818,#35819,#35820,#35821,#35822,#35823,
#35824,#35825,#35826,#35827,#35828,#35829,#35830,#35831,#35832,#35833,#35834,
#35835,#35836,#35837,#35838),.UNSPECIFIED.,.F.,.F.,(6,1,1,1,1,1,1,1,1,1,
1,1,1,1,1,1,1,1,1,1,1,1,1,1,1,1,1,1,1,1,1,1,1,1,1,1,1,1,1,1,1,1,1,1,1,1,
1,1,1,1,1,1,1,1,1,1,1,1,1,1,1,1,1,1,1,1,1,1,1,1,6),(-1.,-0.985714285714284,
-0.97142857142857,-0.957142857142856,-0.942857142857141,-0.928571428571427,
-0.914285714285713,-0.899999999999999,-0.885714285714284,-0.87142857142857,
-0.857142857142856,-0.842857142857142,-0.828571428571428,-0.814285714285713,
-0.799999999999999,-0.785714285714285,-0.771428571428571,-0.757142857142856,
-0.742857142857142,-0.728571428571428,-0.714285714285714,-0.699999999999999,
-0.685714285714285,-0.671428571428571,-0.657142857142857,-0.642857142857142,
-0.628571428571428,-0.614285714285714,-0.6,-0.585714285714286,-0.571428571428571,
-0.557142857142857,-0.542857142857143,-0.528571428571429,-0.514285714285714,
-0.5,-0.485714285714286,-0.471428571428572,-0.457142857142857,-0.442857142857143,
-0.428571428571429,-0.414285714285714,-0.4,-0.385714285714286,-0.371428571428571,
-0.357142857142857,-0.342857142857143,-0.328571428571429,-0.314285714285714,
-0.3,-0.285714285714286,-0.271428571428571,-0.257142857142857,-0.242857142857143,
-0.228571428571429,-0.214285714285714,-0.2,-0.185714285714286,-0.171428571428571,
-0.157142857142857,-0.142857142857143,-0.128571428571429,-0.114285714285714,
-0.1,-0.0857142857142857,-0.0714285714285714,-0.0571428571428571,-0.0428571428571429,
-0.0285714285714286,-0.0142857142857143,0.),.UNSPECIFIED.);
#597=B_SPLINE_CURVE_WITH_KNOTS('',5,(#35996,#35997,#35998,#35999,#36000,
#36001,#36002,#36003,#36004,#36005,#36006,#36007,#36008,#36009,#36010,#36011,
#36012,#36013,#36014,#36015,#36016,#36017,#36018,#36019,#36020,#36021,#36022,
#36023,#36024,#36025,#36026,#36027,#36028,#36029,#36030,#36031,#36032,#36033,
#36034,#36035,#36036,#36037,#36038,#36039,#36040,#36041,#36042,#36043,#36044,
#36045,#36046,#36047,#36048,#36049,#36050,#36051,#36052,#36053,#36054,#36055,
#36056,#36057,#36058,#36059,#36060,#36061,#36062,#36063,#36064,#36065,#36066,
#36067,#36068,#36069),.UNSPECIFIED.,.F.,.F.,(6,1,1,1,1,1,1,1,1,1,1,1,1,
1,1,1,1,1,1,1,1,1,1,1,1,1,1,1,1,1,1,1,1,1,1,1,1,1,1,1,1,1,1,1,1,1,1,1,1,
1,1,1,1,1,1,1,1,1,1,1,1,1,1,1,1,1,1,1,1,6),(0.,0.0142857142857143,0.0285714285714286,
0.0428571428571429,0.0571428571428571,0.0714285714285714,0.0857142857142857,
0.1,0.114285714285714,0.128571428571429,0.142857142857143,0.157142857142857,
0.171428571428571,0.185714285714286,0.2,0.214285714285714,0.228571428571429,
0.242857142857143,0.257142857142857,0.271428571428571,0.285714285714286,
0.3,0.314285714285714,0.328571428571429,0.342857142857143,0.357142857142857,
0.371428571428571,0.385714285714286,0.4,0.414285714285714,0.428571428571429,
0.442857142857143,0.457142857142857,0.471428571428572,0.485714285714286,
0.5,0.514285714285714,0.528571428571429,0.542857142857143,0.557142857142857,
0.571428571428571,0.585714285714286,0.6,0.614285714285714,0.628571428571428,
0.642857142857142,0.657142857142857,0.671428571428571,0.685714285714285,
0.699999999999999,0.714285714285714,0.728571428571428,0.742857142857142,
0.757142857142856,0.771428571428571,0.785714285714285,0.799999999999999,
0.814285714285713,0.828571428571428,0.842857142857142,0.857142857142856,
0.87142857142857,0.885714285714284,0.899999999999999,0.914285714285713,
0.928571428571427,0.942857142857141,0.957142857142856,0.97142857142857,
1.),.UNSPECIFIED.);
#598=B_SPLINE_CURVE_WITH_KNOTS('',5,(#36070,#36071,#36072,#36073,#36074,
#36075,#36076,#36077,#36078,#36079,#36080,#36081,#36082,#36083,#36084,#36085,
#36086,#36087,#36088,#36089,#36090,#36091,#36092,#36093,#36094,#36095,#36096,
#36097,#36098,#36099,#36100,#36101,#36102,#36103,#36104,#36105,#36106,#36107,
#36108,#36109,#36110,#36111,#36112,#36113,#36114,#36115,#36116,#36117,#36118,
#36119,#36120,#36121,#36122,#36123,#36124,#36125,#36126,#36127,#36128,#36129,
#36130,#36131,#36132,#36133,#36134,#36135,#36136,#36137,#36138,#36139,#36140,
#36141,#36142,#36143),.UNSPECIFIED.,.F.,.F.,(6,1,1,1,1,1,1,1,1,1,1,1,1,
1,1,1,1,1,1,1,1,1,1,1,1,1,1,1,1,1,1,1,1,1,1,1,1,1,1,1,1,1,1,1,1,1,1,1,1,
1,1,1,1,1,1,1,1,1,1,1,1,1,1,1,1,1,1,1,1,6),(0.,0.0142857142857143,0.0285714285714286,
0.0428571428571429,0.0571428571428571,0.0714285714285714,0.0857142857142857,
0.1,0.114285714285714,0.128571428571429,0.142857142857143,0.157142857142857,
0.171428571428571,0.185714285714286,0.2,0.214285714285714,0.228571428571429,
0.242857142857143,0.257142857142857,0.271428571428571,0.285714285714286,
0.3,0.314285714285714,0.328571428571429,0.342857142857143,0.357142857142857,
0.371428571428571,0.385714285714286,0.4,0.414285714285714,0.428571428571429,
0.442857142857143,0.457142857142857,0.471428571428572,0.485714285714286,
0.5,0.514285714285714,0.528571428571429,0.542857142857143,0.557142857142857,
0.571428571428571,0.585714285714286,0.6,0.614285714285714,0.628571428571428,
0.642857142857142,0.657142857142857,0.671428571428571,0.685714285714285,
0.699999999999999,0.714285714285714,0.728571428571428,0.742857142857142,
0.757142857142856,0.771428571428571,0.785714285714285,0.799999999999999,
0.814285714285713,0.828571428571428,0.842857142857142,0.857142857142856,
0.87142857142857,0.885714285714284,0.899999999999999,0.914285714285713,
0.928571428571427,0.942857142857141,0.957142857142856,0.97142857142857,
1.),.UNSPECIFIED.);
#599=B_SPLINE_CURVE_WITH_KNOTS('',5,(#36295,#36296,#36297,#36298,#36299,
#36300,#36301,#36302,#36303,#36304,#36305,#36306,#36307,#36308,#36309,#36310,
#36311,#36312,#36313,#36314,#36315,#36316,#36317,#36318,#36319,#36320,#36321,
#36322,#36323,#36324,#36325,#36326,#36327,#36328,#36329,#36330,#36331,#36332,
#36333,#36334,#36335,#36336,#36337,#36338,#36339,#36340,#36341,#36342,#36343,
#36344,#36345,#36346,#36347,#36348,#36349,#36350,#36351,#36352,#36353,#36354,
#36355,#36356,#36357,#36358,#36359,#36360,#36361,#36362,#36363,#36364,#36365,
#36366,#36367,#36368),.UNSPECIFIED.,.F.,.F.,(6,1,1,1,1,1,1,1,1,1,1,1,1,
1,1,1,1,1,1,1,1,1,1,1,1,1,1,1,1,1,1,1,1,1,1,1,1,1,1,1,1,1,1,1,1,1,1,1,1,
1,1,1,1,1,1,1,1,1,1,1,1,1,1,1,1,1,1,1,1,6),(0.,0.0142857142857143,0.0285714285714286,
0.0428571428571429,0.0571428571428571,0.0714285714285714,0.0857142857142857,
0.1,0.114285714285714,0.128571428571429,0.142857142857143,0.157142857142857,
0.171428571428571,0.185714285714286,0.2,0.214285714285714,0.228571428571429,
0.242857142857143,0.257142857142857,0.271428571428571,0.285714285714286,
0.3,0.314285714285714,0.328571428571429,0.342857142857143,0.357142857142857,
0.371428571428571,0.385714285714286,0.4,0.414285714285714,0.428571428571429,
0.442857142857143,0.457142857142857,0.471428571428572,0.485714285714286,
0.5,0.514285714285714,0.528571428571429,0.542857142857143,0.557142857142857,
0.571428571428571,0.585714285714286,0.6,0.614285714285714,0.628571428571428,
0.642857142857142,0.657142857142857,0.671428571428571,0.685714285714285,
0.699999999999999,0.714285714285714,0.728571428571428,0.742857142857142,
0.757142857142856,0.771428571428571,0.785714285714285,0.799999999999999,
0.814285714285713,0.828571428571428,0.842857142857142,0.857142857142856,
0.87142857142857,0.885714285714284,0.899999999999999,0.914285714285713,
0.928571428571427,0.942857142857141,0.957142857142856,0.97142857142857,
1.),.UNSPECIFIED.);
#600=B_SPLINE_CURVE_WITH_KNOTS('',5,(#36370,#36371,#36372,#36373,#36374,
#36375,#36376,#36377,#36378,#36379,#36380,#36381,#36382,#36383,#36384,#36385,
#36386,#36387,#36388,#36389,#36390,#36391,#36392,#36393,#36394,#36395,#36396,
#36397,#36398,#36399,#36400,#36401,#36402,#36403,#36404,#36405,#36406,#36407,
#36408,#36409,#36410,#36411,#36412,#36413,#36414,#36415,#36416,#36417,#36418,
#36419,#36420,#36421,#36422,#36423,#36424,#36425,#36426,#36427,#36428,#36429,
#36430,#36431,#36432,#36433,#36434,#36435,#36436,#36437,#36438,#36439,#36440,
#36441,#36442,#36443,#36444),.UNSPECIFIED.,.F.,.F.,(6,1,1,1,1,1,1,1,1,1,
1,1,1,1,1,1,1,1,1,1,1,1,1,1,1,1,1,1,1,1,1,1,1,1,1,1,1,1,1,1,1,1,1,1,1,1,
1,1,1,1,1,1,1,1,1,1,1,1,1,1,1,1,1,1,1,1,1,1,1,1,6),(-1.,-0.985714285714284,
-0.97142857142857,-0.957142857142856,-0.942857142857141,-0.928571428571427,
-0.914285714285713,-0.899999999999999,-0.885714285714284,-0.87142857142857,
-0.857142857142856,-0.842857142857142,-0.828571428571428,-0.814285714285713,
-0.799999999999999,-0.785714285714285,-0.771428571428571,-0.757142857142856,
-0.742857142857142,-0.728571428571428,-0.714285714285714,-0.699999999999999,
-0.685714285714285,-0.671428571428571,-0.657142857142857,-0.642857142857142,
-0.628571428571428,-0.614285714285714,-0.6,-0.585714285714286,-0.571428571428571,
-0.557142857142857,-0.542857142857143,-0.528571428571429,-0.514285714285714,
-0.5,-0.485714285714286,-0.471428571428572,-0.457142857142857,-0.442857142857143,
-0.428571428571429,-0.414285714285714,-0.4,-0.385714285714286,-0.371428571428571,
-0.357142857142857,-0.342857142857143,-0.328571428571429,-0.314285714285714,
-0.3,-0.285714285714286,-0.271428571428571,-0.257142857142857,-0.242857142857143,
-0.228571428571429,-0.214285714285714,-0.2,-0.185714285714286,-0.171428571428571,
-0.157142857142857,-0.142857142857143,-0.128571428571429,-0.114285714285714,
-0.1,-0.0857142857142857,-0.0714285714285714,-0.0571428571428571,-0.0428571428571429,
-0.0285714285714286,-0.0142857142857143,0.),.UNSPECIFIED.);
#601=B_SPLINE_CURVE_WITH_KNOTS('',5,(#36602,#36603,#36604,#36605,#36606,
#36607,#36608,#36609,#36610,#36611,#36612,#36613,#36614,#36615,#36616,#36617,
#36618,#36619,#36620,#36621,#36622,#36623,#36624,#36625,#36626,#36627,#36628,
#36629,#36630,#36631,#36632,#36633,#36634,#36635,#36636,#36637,#36638,#36639,
#36640,#36641,#36642,#36643,#36644,#36645,#36646,#36647,#36648,#36649,#36650,
#36651,#36652,#36653,#36654,#36655,#36656,#36657,#36658,#36659,#36660,#36661,
#36662,#36663,#36664,#36665,#36666,#36667,#36668,#36669,#36670,#36671,#36672,
#36673,#36674,#36675),.UNSPECIFIED.,.F.,.F.,(6,1,1,1,1,1,1,1,1,1,1,1,1,
1,1,1,1,1,1,1,1,1,1,1,1,1,1,1,1,1,1,1,1,1,1,1,1,1,1,1,1,1,1,1,1,1,1,1,1,
1,1,1,1,1,1,1,1,1,1,1,1,1,1,1,1,1,1,1,1,6),(0.,0.0142857142857143,0.0285714285714286,
0.0428571428571429,0.0571428571428571,0.0714285714285714,0.0857142857142857,
0.1,0.114285714285714,0.128571428571429,0.142857142857143,0.157142857142857,
0.171428571428571,0.185714285714286,0.2,0.214285714285714,0.228571428571429,
0.242857142857143,0.257142857142857,0.271428571428571,0.285714285714286,
0.3,0.314285714285714,0.328571428571429,0.342857142857143,0.357142857142857,
0.371428571428571,0.385714285714286,0.4,0.414285714285714,0.428571428571429,
0.442857142857143,0.457142857142857,0.471428571428572,0.485714285714286,
0.5,0.514285714285714,0.528571428571429,0.542857142857143,0.557142857142857,
0.571428571428571,0.585714285714286,0.6,0.614285714285714,0.628571428571428,
0.642857142857142,0.657142857142857,0.671428571428571,0.685714285714285,
0.699999999999999,0.714285714285714,0.728571428571428,0.742857142857142,
0.757142857142856,0.771428571428571,0.785714285714285,0.799999999999999,
0.814285714285713,0.828571428571428,0.842857142857142,0.857142857142856,
0.87142857142857,0.885714285714284,0.899999999999999,0.914285714285713,
0.928571428571427,0.942857142857141,0.957142857142856,0.97142857142857,
1.),.UNSPECIFIED.);
#602=B_SPLINE_CURVE_WITH_KNOTS('',5,(#36676,#36677,#36678,#36679,#36680,
#36681,#36682,#36683,#36684,#36685,#36686,#36687,#36688,#36689,#36690,#36691,
#36692,#36693,#36694,#36695,#36696,#36697,#36698,#36699,#36700,#36701,#36702,
#36703,#36704,#36705,#36706,#36707,#36708,#36709,#36710,#36711,#36712,#36713,
#36714,#36715,#36716,#36717,#36718,#36719,#36720,#36721,#36722,#36723,#36724,
#36725,#36726,#36727,#36728,#36729,#36730,#36731,#36732,#36733,#36734,#36735,
#36736,#36737,#36738,#36739,#36740,#36741,#36742,#36743,#36744,#36745,#36746,
#36747,#36748,#36749),.UNSPECIFIED.,.F.,.F.,(6,1,1,1,1,1,1,1,1,1,1,1,1,
1,1,1,1,1,1,1,1,1,1,1,1,1,1,1,1,1,1,1,1,1,1,1,1,1,1,1,1,1,1,1,1,1,1,1,1,
1,1,1,1,1,1,1,1,1,1,1,1,1,1,1,1,1,1,1,1,6),(0.,0.0142857142857143,0.0285714285714286,
0.0428571428571429,0.0571428571428571,0.0714285714285714,0.0857142857142857,
0.1,0.114285714285714,0.128571428571429,0.142857142857143,0.157142857142857,
0.171428571428571,0.185714285714286,0.2,0.214285714285714,0.228571428571429,
0.242857142857143,0.257142857142857,0.271428571428571,0.285714285714286,
0.3,0.314285714285714,0.328571428571429,0.342857142857143,0.357142857142857,
0.371428571428571,0.385714285714286,0.4,0.414285714285714,0.428571428571429,
0.442857142857143,0.457142857142857,0.471428571428572,0.485714285714286,
0.5,0.514285714285714,0.528571428571429,0.542857142857143,0.557142857142857,
0.571428571428571,0.585714285714286,0.6,0.614285714285714,0.628571428571428,
0.642857142857142,0.657142857142857,0.671428571428571,0.685714285714285,
0.699999999999999,0.714285714285714,0.728571428571428,0.742857142857142,
0.757142857142856,0.771428571428571,0.785714285714285,0.799999999999999,
0.814285714285713,0.828571428571428,0.842857142857142,0.857142857142856,
0.87142857142857,0.885714285714284,0.899999999999999,0.914285714285713,
0.928571428571427,0.942857142857141,0.957142857142856,0.97142857142857,
1.),.UNSPECIFIED.);
#603=B_SPLINE_CURVE_WITH_KNOTS('',5,(#36901,#36902,#36903,#36904,#36905,
#36906,#36907,#36908,#36909,#36910,#36911,#36912,#36913,#36914,#36915,#36916,
#36917,#36918,#36919,#36920,#36921,#36922,#36923,#36924,#36925,#36926,#36927,
#36928,#36929,#36930,#36931,#36932,#36933,#36934,#36935,#36936,#36937,#36938,
#36939,#36940,#36941,#36942,#36943,#36944,#36945,#36946,#36947,#36948,#36949,
#36950,#36951,#36952,#36953,#36954,#36955,#36956,#36957,#36958,#36959,#36960,
#36961,#36962,#36963,#36964,#36965,#36966,#36967,#36968,#36969,#36970,#36971,
#36972,#36973,#36974),.UNSPECIFIED.,.F.,.F.,(6,1,1,1,1,1,1,1,1,1,1,1,1,
1,1,1,1,1,1,1,1,1,1,1,1,1,1,1,1,1,1,1,1,1,1,1,1,1,1,1,1,1,1,1,1,1,1,1,1,
1,1,1,1,1,1,1,1,1,1,1,1,1,1,1,1,1,1,1,1,6),(0.,0.0142857142857143,0.0285714285714286,
0.0428571428571429,0.0571428571428571,0.0714285714285714,0.0857142857142857,
0.1,0.114285714285714,0.128571428571429,0.142857142857143,0.157142857142857,
0.171428571428571,0.185714285714286,0.2,0.214285714285714,0.228571428571429,
0.242857142857143,0.257142857142857,0.271428571428571,0.285714285714286,
0.3,0.314285714285714,0.328571428571429,0.342857142857143,0.357142857142857,
0.371428571428571,0.385714285714286,0.4,0.414285714285714,0.428571428571429,
0.442857142857143,0.457142857142857,0.471428571428572,0.485714285714286,
0.5,0.514285714285714,0.528571428571429,0.542857142857143,0.557142857142857,
0.571428571428571,0.585714285714286,0.6,0.614285714285714,0.628571428571428,
0.642857142857142,0.657142857142857,0.671428571428571,0.685714285714285,
0.699999999999999,0.714285714285714,0.728571428571428,0.742857142857142,
0.757142857142856,0.771428571428571,0.785714285714285,0.799999999999999,
0.814285714285713,0.828571428571428,0.842857142857142,0.857142857142856,
0.87142857142857,0.885714285714284,0.899999999999999,0.914285714285713,
0.928571428571427,0.942857142857141,0.957142857142856,0.97142857142857,
1.),.UNSPECIFIED.);
#604=B_SPLINE_CURVE_WITH_KNOTS('',5,(#36976,#36977,#36978,#36979,#36980,
#36981,#36982,#36983,#36984,#36985,#36986,#36987,#36988,#36989,#36990,#36991,
#36992,#36993,#36994,#36995,#36996,#36997,#36998,#36999,#37000,#37001,#37002,
#37003,#37004,#37005,#37006,#37007,#37008,#37009,#37010,#37011,#37012,#37013,
#37014,#37015,#37016,#37017,#37018,#37019,#37020,#37021,#37022,#37023,#37024,
#37025,#37026,#37027,#37028,#37029,#37030,#37031,#37032,#37033,#37034,#37035,
#37036,#37037,#37038,#37039,#37040,#37041,#37042,#37043,#37044,#37045,#37046,
#37047,#37048,#37049,#37050),.UNSPECIFIED.,.F.,.F.,(6,1,1,1,1,1,1,1,1,1,
1,1,1,1,1,1,1,1,1,1,1,1,1,1,1,1,1,1,1,1,1,1,1,1,1,1,1,1,1,1,1,1,1,1,1,1,
1,1,1,1,1,1,1,1,1,1,1,1,1,1,1,1,1,1,1,1,1,1,1,1,6),(-1.,-0.985714285714284,
-0.97142857142857,-0.957142857142856,-0.942857142857141,-0.928571428571427,
-0.914285714285713,-0.899999999999999,-0.885714285714284,-0.87142857142857,
-0.857142857142856,-0.842857142857142,-0.828571428571428,-0.814285714285713,
-0.799999999999999,-0.785714285714285,-0.771428571428571,-0.757142857142856,
-0.742857142857142,-0.728571428571428,-0.714285714285714,-0.699999999999999,
-0.685714285714285,-0.671428571428571,-0.657142857142857,-0.642857142857142,
-0.628571428571428,-0.614285714285714,-0.6,-0.585714285714286,-0.571428571428571,
-0.557142857142857,-0.542857142857143,-0.528571428571429,-0.514285714285714,
-0.5,-0.485714285714286,-0.471428571428572,-0.457142857142857,-0.442857142857143,
-0.428571428571429,-0.414285714285714,-0.4,-0.385714285714286,-0.371428571428571,
-0.357142857142857,-0.342857142857143,-0.328571428571429,-0.314285714285714,
-0.3,-0.285714285714286,-0.271428571428571,-0.257142857142857,-0.242857142857143,
-0.228571428571429,-0.214285714285714,-0.2,-0.185714285714286,-0.171428571428571,
-0.157142857142857,-0.142857142857143,-0.128571428571429,-0.114285714285714,
-0.1,-0.0857142857142857,-0.0714285714285714,-0.0571428571428571,-0.0428571428571429,
-0.0285714285714286,-0.0142857142857143,0.),.UNSPECIFIED.);
#605=B_SPLINE_CURVE_WITH_KNOTS('',5,(#37208,#37209,#37210,#37211,#37212,
#37213,#37214,#37215,#37216,#37217,#37218,#37219,#37220,#37221,#37222,#37223,
#37224,#37225,#37226,#37227,#37228,#37229,#37230,#37231,#37232,#37233,#37234,
#37235,#37236,#37237,#37238,#37239,#37240,#37241,#37242,#37243,#37244,#37245,
#37246,#37247,#37248,#37249,#37250,#37251,#37252,#37253,#37254,#37255,#37256,
#37257,#37258,#37259,#37260,#37261,#37262,#37263,#37264,#37265,#37266,#37267,
#37268,#37269,#37270,#37271,#37272,#37273,#37274,#37275,#37276,#37277,#37278,
#37279,#37280,#37281),.UNSPECIFIED.,.F.,.F.,(6,1,1,1,1,1,1,1,1,1,1,1,1,
1,1,1,1,1,1,1,1,1,1,1,1,1,1,1,1,1,1,1,1,1,1,1,1,1,1,1,1,1,1,1,1,1,1,1,1,
1,1,1,1,1,1,1,1,1,1,1,1,1,1,1,1,1,1,1,1,6),(0.,0.0142857142857143,0.0285714285714286,
0.0428571428571429,0.0571428571428571,0.0714285714285714,0.0857142857142857,
0.1,0.114285714285714,0.128571428571429,0.142857142857143,0.157142857142857,
0.171428571428571,0.185714285714286,0.2,0.214285714285714,0.228571428571429,
0.242857142857143,0.257142857142857,0.271428571428571,0.285714285714286,
0.3,0.314285714285714,0.328571428571429,0.342857142857143,0.357142857142857,
0.371428571428571,0.385714285714286,0.4,0.414285714285714,0.428571428571429,
0.442857142857143,0.457142857142857,0.471428571428572,0.485714285714286,
0.5,0.514285714285714,0.528571428571429,0.542857142857143,0.557142857142857,
0.571428571428571,0.585714285714286,0.6,0.614285714285714,0.628571428571428,
0.642857142857142,0.657142857142857,0.671428571428571,0.685714285714285,
0.699999999999999,0.714285714285714,0.728571428571428,0.742857142857142,
0.757142857142856,0.771428571428571,0.785714285714285,0.799999999999999,
0.814285714285713,0.828571428571428,0.842857142857142,0.857142857142856,
0.87142857142857,0.885714285714284,0.899999999999999,0.914285714285713,
0.928571428571427,0.942857142857141,0.957142857142856,0.97142857142857,
1.),.UNSPECIFIED.);
#606=B_SPLINE_CURVE_WITH_KNOTS('',5,(#37282,#37283,#37284,#37285,#37286,
#37287,#37288,#37289,#37290,#37291,#37292,#37293,#37294,#37295,#37296,#37297,
#37298,#37299,#37300,#37301,#37302,#37303,#37304,#37305,#37306,#37307,#37308,
#37309,#37310,#37311,#37312,#37313,#37314,#37315,#37316,#37317,#37318,#37319,
#37320,#37321,#37322,#37323,#37324,#37325,#37326,#37327,#37328,#37329,#37330,
#37331,#37332,#37333,#37334,#37335,#37336,#37337,#37338,#37339,#37340,#37341,
#37342,#37343,#37344,#37345,#37346,#37347,#37348,#37349,#37350,#37351,#37352,
#37353,#37354,#37355),.UNSPECIFIED.,.F.,.F.,(6,1,1,1,1,1,1,1,1,1,1,1,1,
1,1,1,1,1,1,1,1,1,1,1,1,1,1,1,1,1,1,1,1,1,1,1,1,1,1,1,1,1,1,1,1,1,1,1,1,
1,1,1,1,1,1,1,1,1,1,1,1,1,1,1,1,1,1,1,1,6),(0.,0.0142857142857143,0.0285714285714286,
0.0428571428571429,0.0571428571428571,0.0714285714285714,0.0857142857142857,
0.1,0.114285714285714,0.128571428571429,0.142857142857143,0.157142857142857,
0.171428571428571,0.185714285714286,0.2,0.214285714285714,0.228571428571429,
0.242857142857143,0.257142857142857,0.271428571428571,0.285714285714286,
0.3,0.314285714285714,0.328571428571429,0.342857142857143,0.357142857142857,
0.371428571428571,0.385714285714286,0.4,0.414285714285714,0.428571428571429,
0.442857142857143,0.457142857142857,0.471428571428572,0.485714285714286,
0.5,0.514285714285714,0.528571428571429,0.542857142857143,0.557142857142857,
0.571428571428571,0.585714285714286,0.6,0.614285714285714,0.628571428571428,
0.642857142857142,0.657142857142857,0.671428571428571,0.685714285714285,
0.699999999999999,0.714285714285714,0.728571428571428,0.742857142857142,
0.757142857142856,0.771428571428571,0.785714285714285,0.799999999999999,
0.814285714285713,0.828571428571428,0.842857142857142,0.857142857142856,
0.87142857142857,0.885714285714284,0.899999999999999,0.914285714285713,
0.928571428571427,0.942857142857141,0.957142857142856,0.97142857142857,
1.),.UNSPECIFIED.);
#607=B_SPLINE_CURVE_WITH_KNOTS('',5,(#37371,#37372,#37373,#37374,#37375,
#37376,#37377,#37378,#37379,#37380,#37381,#37382,#37383,#37384,#37385,#37386,
#37387,#37388,#37389,#37390,#37391,#37392,#37393,#37394,#37395,#37396,#37397,
#37398,#37399,#37400,#37401,#37402,#37403,#37404,#37405,#37406,#37407,#37408,
#37409,#37410,#37411,#37412,#37413,#37414,#37415,#37416,#37417,#37418,#37419,
#37420,#37421,#37422,#37423,#37424,#37425,#37426,#37427,#37428,#37429,#37430,
#37431,#37432,#37433,#37434,#37435,#37436,#37437,#37438,#37439,#37440,#37441,
#37442,#37443,#37444),.UNSPECIFIED.,.F.,.F.,(6,1,1,1,1,1,1,1,1,1,1,1,1,
1,1,1,1,1,1,1,1,1,1,1,1,1,1,1,1,1,1,1,1,1,1,1,1,1,1,1,1,1,1,1,1,1,1,1,1,
1,1,1,1,1,1,1,1,1,1,1,1,1,1,1,1,1,1,1,1,6),(0.,0.0142857142857143,0.0285714285714286,
0.0428571428571429,0.0571428571428571,0.0714285714285714,0.0857142857142857,
0.1,0.114285714285714,0.128571428571429,0.142857142857143,0.157142857142857,
0.171428571428571,0.185714285714286,0.2,0.214285714285714,0.228571428571429,
0.242857142857143,0.257142857142857,0.271428571428571,0.285714285714286,
0.3,0.314285714285714,0.328571428571429,0.342857142857143,0.357142857142857,
0.371428571428571,0.385714285714286,0.4,0.414285714285714,0.428571428571429,
0.442857142857143,0.457142857142857,0.471428571428572,0.485714285714286,
0.5,0.514285714285714,0.528571428571429,0.542857142857143,0.557142857142857,
0.571428571428571,0.585714285714286,0.6,0.614285714285714,0.628571428571428,
0.642857142857142,0.657142857142857,0.671428571428571,0.685714285714285,
0.699999999999999,0.714285714285714,0.728571428571428,0.742857142857142,
0.757142857142856,0.771428571428571,0.785714285714285,0.799999999999999,
0.814285714285713,0.828571428571428,0.842857142857142,0.857142857142856,
0.87142857142857,0.885714285714284,0.899999999999999,0.914285714285713,
0.928571428571427,0.942857142857141,0.957142857142856,0.97142857142857,
1.),.UNSPECIFIED.);
#608=B_SPLINE_CURVE_WITH_KNOTS('',5,(#37448,#37449,#37450,#37451,#37452,
#37453,#37454,#37455,#37456,#37457,#37458,#37459,#37460,#37461,#37462,#37463,
#37464,#37465,#37466,#37467,#37468,#37469,#37470,#37471,#37472,#37473,#37474,
#37475,#37476,#37477,#37478,#37479,#37480,#37481,#37482,#37483,#37484,#37485,
#37486,#37487,#37488,#37489,#37490,#37491,#37492,#37493,#37494,#37495,#37496,
#37497,#37498,#37499,#37500,#37501,#37502,#37503,#37504,#37505,#37506,#37507,
#37508,#37509,#37510,#37511,#37512,#37513,#37514,#37515,#37516,#37517,#37518,
#37519,#37520,#37521),.UNSPECIFIED.,.F.,.F.,(6,1,1,1,1,1,1,1,1,1,1,1,1,
1,1,1,1,1,1,1,1,1,1,1,1,1,1,1,1,1,1,1,1,1,1,1,1,1,1,1,1,1,1,1,1,1,1,1,1,
1,1,1,1,1,1,1,1,1,1,1,1,1,1,1,1,1,1,1,1,6),(0.,0.0142857142857143,0.0285714285714286,
0.0428571428571429,0.0571428571428571,0.0714285714285714,0.0857142857142857,
0.1,0.114285714285714,0.128571428571429,0.142857142857143,0.157142857142857,
0.171428571428571,0.185714285714286,0.2,0.214285714285714,0.228571428571429,
0.242857142857143,0.257142857142857,0.271428571428571,0.285714285714286,
0.3,0.314285714285714,0.328571428571429,0.342857142857143,0.357142857142857,
0.371428571428571,0.385714285714286,0.4,0.414285714285714,0.428571428571429,
0.442857142857143,0.457142857142857,0.471428571428572,0.485714285714286,
0.5,0.514285714285714,0.528571428571429,0.542857142857143,0.557142857142857,
0.571428571428571,0.585714285714286,0.6,0.614285714285714,0.628571428571428,
0.642857142857142,0.657142857142857,0.671428571428571,0.685714285714285,
0.699999999999999,0.714285714285714,0.728571428571428,0.742857142857142,
0.757142857142856,0.771428571428571,0.785714285714285,0.799999999999999,
0.814285714285713,0.828571428571428,0.842857142857142,0.857142857142856,
0.87142857142857,0.885714285714284,0.899999999999999,0.914285714285713,
0.928571428571427,0.942857142857141,0.957142857142856,0.97142857142857,
1.),.UNSPECIFIED.);
#609=B_SPLINE_CURVE_WITH_KNOTS('',5,(#37536,#37537,#37538,#37539,#37540,
#37541,#37542,#37543,#37544,#37545,#37546,#37547,#37548,#37549,#37550,#37551,
#37552,#37553,#37554,#37555,#37556,#37557,#37558,#37559,#37560,#37561,#37562,
#37563,#37564,#37565,#37566,#37567,#37568,#37569,#37570,#37571,#37572,#37573,
#37574,#37575,#37576,#37577,#37578,#37579,#37580,#37581,#37582,#37583,#37584,
#37585,#37586,#37587,#37588,#37589,#37590,#37591,#37592,#37593,#37594,#37595,
#37596,#37597,#37598,#37599,#37600,#37601,#37602,#37603,#37604,#37605,#37606,
#37607,#37608,#37609),.UNSPECIFIED.,.F.,.F.,(6,1,1,1,1,1,1,1,1,1,1,1,1,
1,1,1,1,1,1,1,1,1,1,1,1,1,1,1,1,1,1,1,1,1,1,1,1,1,1,1,1,1,1,1,1,1,1,1,1,
1,1,1,1,1,1,1,1,1,1,1,1,1,1,1,1,1,1,1,1,6),(0.,0.0142857142857143,0.0285714285714286,
0.0428571428571429,0.0571428571428571,0.0714285714285714,0.0857142857142857,
0.1,0.114285714285714,0.128571428571429,0.142857142857143,0.157142857142857,
0.171428571428571,0.185714285714286,0.2,0.214285714285714,0.228571428571429,
0.242857142857143,0.257142857142857,0.271428571428571,0.285714285714286,
0.3,0.314285714285714,0.328571428571429,0.342857142857143,0.357142857142857,
0.371428571428571,0.385714285714286,0.4,0.414285714285714,0.428571428571429,
0.442857142857143,0.457142857142857,0.471428571428572,0.485714285714286,
0.5,0.514285714285714,0.528571428571429,0.542857142857143,0.557142857142857,
0.571428571428571,0.585714285714286,0.6,0.614285714285714,0.628571428571428,
0.642857142857142,0.657142857142857,0.671428571428571,0.685714285714285,
0.699999999999999,0.714285714285714,0.728571428571428,0.742857142857142,
0.757142857142856,0.771428571428571,0.785714285714285,0.799999999999999,
0.814285714285713,0.828571428571428,0.842857142857142,0.857142857142856,
0.87142857142857,0.885714285714284,0.899999999999999,0.914285714285713,
0.928571428571427,0.942857142857141,0.957142857142856,0.97142857142857,
1.),.UNSPECIFIED.);
#610=B_SPLINE_CURVE_WITH_KNOTS('',5,(#37613,#37614,#37615,#37616,#37617,
#37618,#37619,#37620,#37621,#37622,#37623,#37624,#37625,#37626,#37627,#37628,
#37629,#37630,#37631,#37632,#37633,#37634,#37635,#37636,#37637,#37638,#37639,
#37640,#37641,#37642,#37643,#37644,#37645,#37646,#37647,#37648,#37649,#37650,
#37651,#37652,#37653,#37654,#37655,#37656,#37657,#37658,#37659,#37660,#37661,
#37662,#37663,#37664,#37665,#37666,#37667,#37668,#37669,#37670,#37671,#37672,
#37673,#37674,#37675,#37676,#37677,#37678,#37679,#37680,#37681,#37682,#37683,
#37684,#37685,#37686,#37687),.UNSPECIFIED.,.F.,.F.,(6,1,1,1,1,1,1,1,1,1,
1,1,1,1,1,1,1,1,1,1,1,1,1,1,1,1,1,1,1,1,1,1,1,1,1,1,1,1,1,1,1,1,1,1,1,1,
1,1,1,1,1,1,1,1,1,1,1,1,1,1,1,1,1,1,1,1,1,1,1,1,6),(-1.,-0.985714285714284,
-0.97142857142857,-0.957142857142856,-0.942857142857141,-0.928571428571427,
-0.914285714285713,-0.899999999999999,-0.885714285714284,-0.87142857142857,
-0.857142857142856,-0.842857142857142,-0.828571428571428,-0.814285714285713,
-0.799999999999999,-0.785714285714285,-0.771428571428571,-0.757142857142856,
-0.742857142857142,-0.728571428571428,-0.714285714285714,-0.699999999999999,
-0.685714285714285,-0.671428571428571,-0.657142857142857,-0.642857142857142,
-0.628571428571428,-0.614285714285714,-0.6,-0.585714285714286,-0.571428571428571,
-0.557142857142857,-0.542857142857143,-0.528571428571429,-0.514285714285714,
-0.5,-0.485714285714286,-0.471428571428572,-0.457142857142857,-0.442857142857143,
-0.428571428571429,-0.414285714285714,-0.4,-0.385714285714286,-0.371428571428571,
-0.357142857142857,-0.342857142857143,-0.328571428571429,-0.314285714285714,
-0.3,-0.285714285714286,-0.271428571428571,-0.257142857142857,-0.242857142857143,
-0.228571428571429,-0.214285714285714,-0.2,-0.185714285714286,-0.171428571428571,
-0.157142857142857,-0.142857142857143,-0.128571428571429,-0.114285714285714,
-0.1,-0.0857142857142857,-0.0714285714285714,-0.0571428571428571,-0.0428571428571429,
-0.0285714285714286,-0.0142857142857143,0.),.UNSPECIFIED.);
#987=B_SPLINE_SURFACE_WITH_KNOTS('',5,1,((#31902,#31903),(#31904,#31905),
(#31906,#31907),(#31908,#31909),(#31910,#31911),(#31912,#31913),(#31914,
#31915),(#31916,#31917),(#31918,#31919),(#31920,#31921),(#31922,#31923),
(#31924,#31925),(#31926,#31927),(#31928,#31929),(#31930,#31931),(#31932,
#31933),(#31934,#31935),(#31936,#31937),(#31938,#31939),(#31940,#31941),
(#31942,#31943),(#31944,#31945),(#31946,#31947),(#31948,#31949),(#31950,
#31951),(#31952,#31953),(#31954,#31955),(#31956,#31957),(#31958,#31959),
(#31960,#31961),(#31962,#31963),(#31964,#31965),(#31966,#31967),(#31968,
#31969),(#31970,#31971),(#31972,#31973),(#31974,#31975),(#31976,#31977),
(#31978,#31979),(#31980,#31981),(#31982,#31983),(#31984,#31985),(#31986,
#31987),(#31988,#31989),(#31990,#31991),(#31992,#31993),(#31994,#31995),
(#31996,#31997),(#31998,#31999),(#32000,#32001),(#32002,#32003),(#32004,
#32005),(#32006,#32007),(#32008,#32009),(#32010,#32011),(#32012,#32013),
(#32014,#32015),(#32016,#32017),(#32018,#32019),(#32020,#32021),(#32022,
#32023),(#32024,#32025),(#32026,#32027),(#32028,#32029),(#32030,#32031),
(#32032,#32033),(#32034,#32035),(#32036,#32037),(#32038,#32039),(#32040,
#32041),(#32042,#32043),(#32044,#32045),(#32046,#32047),(#32048,#32049),
(#32050,#32051)),.UNSPECIFIED.,.F.,.F.,.F.,(6,1,1,1,1,1,1,1,1,1,1,1,1,1,
1,1,1,1,1,1,1,1,1,1,1,1,1,1,1,1,1,1,1,1,1,1,1,1,1,1,1,1,1,1,1,1,1,1,1,1,
1,1,1,1,1,1,1,1,1,1,1,1,1,1,1,1,1,1,1,1,6),(2,2),(-1.,-0.985714285714284,
-0.97142857142857,-0.957142857142856,-0.942857142857141,-0.928571428571427,
-0.914285714285713,-0.899999999999999,-0.885714285714284,-0.87142857142857,
-0.857142857142856,-0.842857142857142,-0.828571428571428,-0.814285714285713,
-0.799999999999999,-0.785714285714285,-0.771428571428571,-0.757142857142856,
-0.742857142857142,-0.728571428571428,-0.714285714285714,-0.699999999999999,
-0.685714285714285,-0.671428571428571,-0.657142857142857,-0.642857142857142,
-0.628571428571428,-0.614285714285714,-0.6,-0.585714285714286,-0.571428571428571,
-0.557142857142857,-0.542857142857143,-0.528571428571429,-0.514285714285714,
-0.5,-0.485714285714286,-0.471428571428572,-0.457142857142857,-0.442857142857143,
-0.428571428571429,-0.414285714285714,-0.4,-0.385714285714286,-0.371428571428571,
-0.357142857142857,-0.342857142857143,-0.328571428571429,-0.314285714285714,
-0.3,-0.285714285714286,-0.271428571428571,-0.257142857142857,-0.242857142857143,
-0.228571428571429,-0.214285714285714,-0.2,-0.185714285714286,-0.171428571428571,
-0.157142857142857,-0.142857142857143,-0.128571428571429,-0.114285714285714,
-0.1,-0.0857142857142857,-0.0714285714285714,-0.0571428571428571,-0.0428571428571429,
-0.0285714285714286,-0.0142857142857143,0.),(0.,1.8),.UNSPECIFIED.);
#988=B_SPLINE_SURFACE_WITH_KNOTS('',5,1,((#32210,#32211),(#32212,#32213),
(#32214,#32215),(#32216,#32217),(#32218,#32219),(#32220,#32221),(#32222,
#32223),(#32224,#32225),(#32226,#32227),(#32228,#32229),(#32230,#32231),
(#32232,#32233),(#32234,#32235),(#32236,#32237),(#32238,#32239),(#32240,
#32241),(#32242,#32243),(#32244,#32245),(#32246,#32247),(#32248,#32249),
(#32250,#32251),(#32252,#32253),(#32254,#32255),(#32256,#32257),(#32258,
#32259),(#32260,#32261),(#32262,#32263),(#32264,#32265),(#32266,#32267),
(#32268,#32269),(#32270,#32271),(#32272,#32273),(#32274,#32275),(#32276,
#32277),(#32278,#32279),(#32280,#32281),(#32282,#32283),(#32284,#32285),
(#32286,#32287),(#32288,#32289),(#32290,#32291),(#32292,#32293),(#32294,
#32295),(#32296,#32297),(#32298,#32299),(#32300,#32301),(#32302,#32303),
(#32304,#32305),(#32306,#32307),(#32308,#32309),(#32310,#32311),(#32312,
#32313),(#32314,#32315),(#32316,#32317),(#32318,#32319),(#32320,#32321),
(#32322,#32323),(#32324,#32325),(#32326,#32327),(#32328,#32329),(#32330,
#32331),(#32332,#32333),(#32334,#32335),(#32336,#32337),(#32338,#32339),
(#32340,#32341),(#32342,#32343),(#32344,#32345),(#32346,#32347),(#32348,
#32349),(#32350,#32351),(#32352,#32353),(#32354,#32355),(#32356,#32357),
(#32358,#32359)),.UNSPECIFIED.,.F.,.F.,.F.,(6,1,1,1,1,1,1,1,1,1,1,1,1,1,
1,1,1,1,1,1,1,1,1,1,1,1,1,1,1,1,1,1,1,1,1,1,1,1,1,1,1,1,1,1,1,1,1,1,1,1,
1,1,1,1,1,1,1,1,1,1,1,1,1,1,1,1,1,1,1,1,6),(2,2),(0.,0.0142857142857143,
0.0285714285714286,0.0428571428571429,0.0571428571428571,0.0714285714285714,
0.0857142857142857,0.1,0.114285714285714,0.128571428571429,0.142857142857143,
0.157142857142857,0.171428571428571,0.185714285714286,0.2,0.214285714285714,
0.228571428571429,0.242857142857143,0.257142857142857,0.271428571428571,
0.285714285714286,0.3,0.314285714285714,0.328571428571429,0.342857142857143,
0.357142857142857,0.371428571428571,0.385714285714286,0.4,0.414285714285714,
0.428571428571429,0.442857142857143,0.457142857142857,0.471428571428572,
0.485714285714286,0.5,0.514285714285714,0.528571428571429,0.542857142857143,
0.557142857142857,0.571428571428571,0.585714285714286,0.6,0.614285714285714,
0.628571428571428,0.642857142857142,0.657142857142857,0.671428571428571,
0.685714285714285,0.699999999999999,0.714285714285714,0.728571428571428,
0.742857142857142,0.757142857142856,0.771428571428571,0.785714285714285,
0.799999999999999,0.814285714285713,0.828571428571428,0.842857142857142,
0.857142857142856,0.87142857142857,0.885714285714284,0.899999999999999,
0.914285714285713,0.928571428571427,0.942857142857141,0.957142857142856,
0.97142857142857,0.985714285714284,1.),(0.,1.8),.UNSPECIFIED.);
#989=B_SPLINE_SURFACE_WITH_KNOTS('',5,1,((#32508,#32509),(#32510,#32511),
(#32512,#32513),(#32514,#32515),(#32516,#32517),(#32518,#32519),(#32520,
#32521),(#32522,#32523),(#32524,#32525),(#32526,#32527),(#32528,#32529),
(#32530,#32531),(#32532,#32533),(#32534,#32535),(#32536,#32537),(#32538,
#32539),(#32540,#32541),(#32542,#32543),(#32544,#32545),(#32546,#32547),
(#32548,#32549),(#32550,#32551),(#32552,#32553),(#32554,#32555),(#32556,
#32557),(#32558,#32559),(#32560,#32561),(#32562,#32563),(#32564,#32565),
(#32566,#32567),(#32568,#32569),(#32570,#32571),(#32572,#32573),(#32574,
#32575),(#32576,#32577),(#32578,#32579),(#32580,#32581),(#32582,#32583),
(#32584,#32585),(#32586,#32587),(#32588,#32589),(#32590,#32591),(#32592,
#32593),(#32594,#32595),(#32596,#32597),(#32598,#32599),(#32600,#32601),
(#32602,#32603),(#32604,#32605),(#32606,#32607),(#32608,#32609),(#32610,
#32611),(#32612,#32613),(#32614,#32615),(#32616,#32617),(#32618,#32619),
(#32620,#32621),(#32622,#32623),(#32624,#32625),(#32626,#32627),(#32628,
#32629),(#32630,#32631),(#32632,#32633),(#32634,#32635),(#32636,#32637),
(#32638,#32639),(#32640,#32641),(#32642,#32643),(#32644,#32645),(#32646,
#32647),(#32648,#32649),(#32650,#32651),(#32652,#32653),(#32654,#32655),
(#32656,#32657)),.UNSPECIFIED.,.F.,.F.,.F.,(6,1,1,1,1,1,1,1,1,1,1,1,1,1,
1,1,1,1,1,1,1,1,1,1,1,1,1,1,1,1,1,1,1,1,1,1,1,1,1,1,1,1,1,1,1,1,1,1,1,1,
1,1,1,1,1,1,1,1,1,1,1,1,1,1,1,1,1,1,1,1,6),(2,2),(-1.,-0.985714285714284,
-0.97142857142857,-0.957142857142856,-0.942857142857141,-0.928571428571427,
-0.914285714285713,-0.899999999999999,-0.885714285714284,-0.87142857142857,
-0.857142857142856,-0.842857142857142,-0.828571428571428,-0.814285714285713,
-0.799999999999999,-0.785714285714285,-0.771428571428571,-0.757142857142856,
-0.742857142857142,-0.728571428571428,-0.714285714285714,-0.699999999999999,
-0.685714285714285,-0.671428571428571,-0.657142857142857,-0.642857142857142,
-0.628571428571428,-0.614285714285714,-0.6,-0.585714285714286,-0.571428571428571,
-0.557142857142857,-0.542857142857143,-0.528571428571429,-0.514285714285714,
-0.5,-0.485714285714286,-0.471428571428572,-0.457142857142857,-0.442857142857143,
-0.428571428571429,-0.414285714285714,-0.4,-0.385714285714286,-0.371428571428571,
-0.357142857142857,-0.342857142857143,-0.328571428571429,-0.314285714285714,
-0.3,-0.285714285714286,-0.271428571428571,-0.257142857142857,-0.242857142857143,
-0.228571428571429,-0.214285714285714,-0.2,-0.185714285714286,-0.171428571428571,
-0.157142857142857,-0.142857142857143,-0.128571428571429,-0.114285714285714,
-0.1,-0.0857142857142857,-0.0714285714285714,-0.0571428571428571,-0.0428571428571429,
-0.0285714285714286,-0.0142857142857143,0.),(0.,1.8),.UNSPECIFIED.);
#990=B_SPLINE_SURFACE_WITH_KNOTS('',5,1,((#32816,#32817),(#32818,#32819),
(#32820,#32821),(#32822,#32823),(#32824,#32825),(#32826,#32827),(#32828,
#32829),(#32830,#32831),(#32832,#32833),(#32834,#32835),(#32836,#32837),
(#32838,#32839),(#32840,#32841),(#32842,#32843),(#32844,#32845),(#32846,
#32847),(#32848,#32849),(#32850,#32851),(#32852,#32853),(#32854,#32855),
(#32856,#32857),(#32858,#32859),(#32860,#32861),(#32862,#32863),(#32864,
#32865),(#32866,#32867),(#32868,#32869),(#32870,#32871),(#32872,#32873),
(#32874,#32875),(#32876,#32877),(#32878,#32879),(#32880,#32881),(#32882,
#32883),(#32884,#32885),(#32886,#32887),(#32888,#32889),(#32890,#32891),
(#32892,#32893),(#32894,#32895),(#32896,#32897),(#32898,#32899),(#32900,
#32901),(#32902,#32903),(#32904,#32905),(#32906,#32907),(#32908,#32909),
(#32910,#32911),(#32912,#32913),(#32914,#32915),(#32916,#32917),(#32918,
#32919),(#32920,#32921),(#32922,#32923),(#32924,#32925),(#32926,#32927),
(#32928,#32929),(#32930,#32931),(#32932,#32933),(#32934,#32935),(#32936,
#32937),(#32938,#32939),(#32940,#32941),(#32942,#32943),(#32944,#32945),
(#32946,#32947),(#32948,#32949),(#32950,#32951),(#32952,#32953),(#32954,
#32955),(#32956,#32957),(#32958,#32959),(#32960,#32961),(#32962,#32963),
(#32964,#32965)),.UNSPECIFIED.,.F.,.F.,.F.,(6,1,1,1,1,1,1,1,1,1,1,1,1,1,
1,1,1,1,1,1,1,1,1,1,1,1,1,1,1,1,1,1,1,1,1,1,1,1,1,1,1,1,1,1,1,1,1,1,1,1,
1,1,1,1,1,1,1,1,1,1,1,1,1,1,1,1,1,1,1,1,6),(2,2),(0.,0.0142857142857143,
0.0285714285714286,0.0428571428571429,0.0571428571428571,0.0714285714285714,
0.0857142857142857,0.1,0.114285714285714,0.128571428571429,0.142857142857143,
0.157142857142857,0.171428571428571,0.185714285714286,0.2,0.214285714285714,
0.228571428571429,0.242857142857143,0.257142857142857,0.271428571428571,
0.285714285714286,0.3,0.314285714285714,0.328571428571429,0.342857142857143,
0.357142857142857,0.371428571428571,0.385714285714286,0.4,0.414285714285714,
0.428571428571429,0.442857142857143,0.457142857142857,0.471428571428572,
0.485714285714286,0.5,0.514285714285714,0.528571428571429,0.542857142857143,
0.557142857142857,0.571428571428571,0.585714285714286,0.6,0.614285714285714,
0.628571428571428,0.642857142857142,0.657142857142857,0.671428571428571,
0.685714285714285,0.699999999999999,0.714285714285714,0.728571428571428,
0.742857142857142,0.757142857142856,0.771428571428571,0.785714285714285,
0.799999999999999,0.814285714285713,0.828571428571428,0.842857142857142,
0.857142857142856,0.87142857142857,0.885714285714284,0.899999999999999,
0.914285714285713,0.928571428571427,0.942857142857141,0.957142857142856,
0.97142857142857,0.985714285714284,1.),(0.,1.8),.UNSPECIFIED.);
#991=B_SPLINE_SURFACE_WITH_KNOTS('',5,1,((#33114,#33115),(#33116,#33117),
(#33118,#33119),(#33120,#33121),(#33122,#33123),(#33124,#33125),(#33126,
#33127),(#33128,#33129),(#33130,#33131),(#33132,#33133),(#33134,#33135),
(#33136,#33137),(#33138,#33139),(#33140,#33141),(#33142,#33143),(#33144,
#33145),(#33146,#33147),(#33148,#33149),(#33150,#33151),(#33152,#33153),
(#33154,#33155),(#33156,#33157),(#33158,#33159),(#33160,#33161),(#33162,
#33163),(#33164,#33165),(#33166,#33167),(#33168,#33169),(#33170,#33171),
(#33172,#33173),(#33174,#33175),(#33176,#33177),(#33178,#33179),(#33180,
#33181),(#33182,#33183),(#33184,#33185),(#33186,#33187),(#33188,#33189),
(#33190,#33191),(#33192,#33193),(#33194,#33195),(#33196,#33197),(#33198,
#33199),(#33200,#33201),(#33202,#33203),(#33204,#33205),(#33206,#33207),
(#33208,#33209),(#33210,#33211),(#33212,#33213),(#33214,#33215),(#33216,
#33217),(#33218,#33219),(#33220,#33221),(#33222,#33223),(#33224,#33225),
(#33226,#33227),(#33228,#33229),(#33230,#33231),(#33232,#33233),(#33234,
#33235),(#33236,#33237),(#33238,#33239),(#33240,#33241),(#33242,#33243),
(#33244,#33245),(#33246,#33247),(#33248,#33249),(#33250,#33251),(#33252,
#33253),(#33254,#33255),(#33256,#33257),(#33258,#33259),(#33260,#33261),
(#33262,#33263)),.UNSPECIFIED.,.F.,.F.,.F.,(6,1,1,1,1,1,1,1,1,1,1,1,1,1,
1,1,1,1,1,1,1,1,1,1,1,1,1,1,1,1,1,1,1,1,1,1,1,1,1,1,1,1,1,1,1,1,1,1,1,1,
1,1,1,1,1,1,1,1,1,1,1,1,1,1,1,1,1,1,1,1,6),(2,2),(-1.,-0.985714285714284,
-0.97142857142857,-0.957142857142856,-0.942857142857141,-0.928571428571427,
-0.914285714285713,-0.899999999999999,-0.885714285714284,-0.87142857142857,
-0.857142857142856,-0.842857142857142,-0.828571428571428,-0.814285714285713,
-0.799999999999999,-0.785714285714285,-0.771428571428571,-0.757142857142856,
-0.742857142857142,-0.728571428571428,-0.714285714285714,-0.699999999999999,
-0.685714285714285,-0.671428571428571,-0.657142857142857,-0.642857142857142,
-0.628571428571428,-0.614285714285714,-0.6,-0.585714285714286,-0.571428571428571,
-0.557142857142857,-0.542857142857143,-0.528571428571429,-0.514285714285714,
-0.5,-0.485714285714286,-0.471428571428572,-0.457142857142857,-0.442857142857143,
-0.428571428571429,-0.414285714285714,-0.4,-0.385714285714286,-0.371428571428571,
-0.357142857142857,-0.342857142857143,-0.328571428571429,-0.314285714285714,
-0.3,-0.285714285714286,-0.271428571428571,-0.257142857142857,-0.242857142857143,
-0.228571428571429,-0.214285714285714,-0.2,-0.185714285714286,-0.171428571428571,
-0.157142857142857,-0.142857142857143,-0.128571428571429,-0.114285714285714,
-0.1,-0.0857142857142857,-0.0714285714285714,-0.0571428571428571,-0.0428571428571429,
-0.0285714285714286,-0.0142857142857143,0.),(0.,1.8),.UNSPECIFIED.);
#992=B_SPLINE_SURFACE_WITH_KNOTS('',5,1,((#33422,#33423),(#33424,#33425),
(#33426,#33427),(#33428,#33429),(#33430,#33431),(#33432,#33433),(#33434,
#33435),(#33436,#33437),(#33438,#33439),(#33440,#33441),(#33442,#33443),
(#33444,#33445),(#33446,#33447),(#33448,#33449),(#33450,#33451),(#33452,
#33453),(#33454,#33455),(#33456,#33457),(#33458,#33459),(#33460,#33461),
(#33462,#33463),(#33464,#33465),(#33466,#33467),(#33468,#33469),(#33470,
#33471),(#33472,#33473),(#33474,#33475),(#33476,#33477),(#33478,#33479),
(#33480,#33481),(#33482,#33483),(#33484,#33485),(#33486,#33487),(#33488,
#33489),(#33490,#33491),(#33492,#33493),(#33494,#33495),(#33496,#33497),
(#33498,#33499),(#33500,#33501),(#33502,#33503),(#33504,#33505),(#33506,
#33507),(#33508,#33509),(#33510,#33511),(#33512,#33513),(#33514,#33515),
(#33516,#33517),(#33518,#33519),(#33520,#33521),(#33522,#33523),(#33524,
#33525),(#33526,#33527),(#33528,#33529),(#33530,#33531),(#33532,#33533),
(#33534,#33535),(#33536,#33537),(#33538,#33539),(#33540,#33541),(#33542,
#33543),(#33544,#33545),(#33546,#33547),(#33548,#33549),(#33550,#33551),
(#33552,#33553),(#33554,#33555),(#33556,#33557),(#33558,#33559),(#33560,
#33561),(#33562,#33563),(#33564,#33565),(#33566,#33567),(#33568,#33569),
(#33570,#33571)),.UNSPECIFIED.,.F.,.F.,.F.,(6,1,1,1,1,1,1,1,1,1,1,1,1,1,
1,1,1,1,1,1,1,1,1,1,1,1,1,1,1,1,1,1,1,1,1,1,1,1,1,1,1,1,1,1,1,1,1,1,1,1,
1,1,1,1,1,1,1,1,1,1,1,1,1,1,1,1,1,1,1,1,6),(2,2),(0.,0.0142857142857143,
0.0285714285714286,0.0428571428571429,0.0571428571428571,0.0714285714285714,
0.0857142857142857,0.1,0.114285714285714,0.128571428571429,0.142857142857143,
0.157142857142857,0.171428571428571,0.185714285714286,0.2,0.214285714285714,
0.228571428571429,0.242857142857143,0.257142857142857,0.271428571428571,
0.285714285714286,0.3,0.314285714285714,0.328571428571429,0.342857142857143,
0.357142857142857,0.371428571428571,0.385714285714286,0.4,0.414285714285714,
0.428571428571429,0.442857142857143,0.457142857142857,0.471428571428572,
0.485714285714286,0.5,0.514285714285714,0.528571428571429,0.542857142857143,
0.557142857142857,0.571428571428571,0.585714285714286,0.6,0.614285714285714,
0.628571428571428,0.642857142857142,0.657142857142857,0.671428571428571,
0.685714285714285,0.699999999999999,0.714285714285714,0.728571428571428,
0.742857142857142,0.757142857142856,0.771428571428571,0.785714285714285,
0.799999999999999,0.814285714285713,0.828571428571428,0.842857142857142,
0.857142857142856,0.87142857142857,0.885714285714284,0.899999999999999,
0.914285714285713,0.928571428571427,0.942857142857141,0.957142857142856,
0.97142857142857,0.985714285714284,1.),(0.,1.8),.UNSPECIFIED.);
#993=B_SPLINE_SURFACE_WITH_KNOTS('',5,1,((#33720,#33721),(#33722,#33723),
(#33724,#33725),(#33726,#33727),(#33728,#33729),(#33730,#33731),(#33732,
#33733),(#33734,#33735),(#33736,#33737),(#33738,#33739),(#33740,#33741),
(#33742,#33743),(#33744,#33745),(#33746,#33747),(#33748,#33749),(#33750,
#33751),(#33752,#33753),(#33754,#33755),(#33756,#33757),(#33758,#33759),
(#33760,#33761),(#33762,#33763),(#33764,#33765),(#33766,#33767),(#33768,
#33769),(#33770,#33771),(#33772,#33773),(#33774,#33775),(#33776,#33777),
(#33778,#33779),(#33780,#33781),(#33782,#33783),(#33784,#33785),(#33786,
#33787),(#33788,#33789),(#33790,#33791),(#33792,#33793),(#33794,#33795),
(#33796,#33797),(#33798,#33799),(#33800,#33801),(#33802,#33803),(#33804,
#33805),(#33806,#33807),(#33808,#33809),(#33810,#33811),(#33812,#33813),
(#33814,#33815),(#33816,#33817),(#33818,#33819),(#33820,#33821),(#33822,
#33823),(#33824,#33825),(#33826,#33827),(#33828,#33829),(#33830,#33831),
(#33832,#33833),(#33834,#33835),(#33836,#33837),(#33838,#33839),(#33840,
#33841),(#33842,#33843),(#33844,#33845),(#33846,#33847),(#33848,#33849),
(#33850,#33851),(#33852,#33853),(#33854,#33855),(#33856,#33857),(#33858,
#33859),(#33860,#33861),(#33862,#33863),(#33864,#33865),(#33866,#33867),
(#33868,#33869)),.UNSPECIFIED.,.F.,.F.,.F.,(6,1,1,1,1,1,1,1,1,1,1,1,1,1,
1,1,1,1,1,1,1,1,1,1,1,1,1,1,1,1,1,1,1,1,1,1,1,1,1,1,1,1,1,1,1,1,1,1,1,1,
1,1,1,1,1,1,1,1,1,1,1,1,1,1,1,1,1,1,1,1,6),(2,2),(-1.,-0.985714285714284,
-0.97142857142857,-0.957142857142856,-0.942857142857141,-0.928571428571427,
-0.914285714285713,-0.899999999999999,-0.885714285714284,-0.87142857142857,
-0.857142857142856,-0.842857142857142,-0.828571428571428,-0.814285714285713,
-0.799999999999999,-0.785714285714285,-0.771428571428571,-0.757142857142856,
-0.742857142857142,-0.728571428571428,-0.714285714285714,-0.699999999999999,
-0.685714285714285,-0.671428571428571,-0.657142857142857,-0.642857142857142,
-0.628571428571428,-0.614285714285714,-0.6,-0.585714285714286,-0.571428571428571,
-0.557142857142857,-0.542857142857143,-0.528571428571429,-0.514285714285714,
-0.5,-0.485714285714286,-0.471428571428572,-0.457142857142857,-0.442857142857143,
-0.428571428571429,-0.414285714285714,-0.4,-0.385714285714286,-0.371428571428571,
-0.357142857142857,-0.342857142857143,-0.328571428571429,-0.314285714285714,
-0.3,-0.285714285714286,-0.271428571428571,-0.257142857142857,-0.242857142857143,
-0.228571428571429,-0.214285714285714,-0.2,-0.185714285714286,-0.171428571428571,
-0.157142857142857,-0.142857142857143,-0.128571428571429,-0.114285714285714,
-0.1,-0.0857142857142857,-0.0714285714285714,-0.0571428571428571,-0.0428571428571429,
-0.0285714285714286,-0.0142857142857143,0.),(0.,1.8),.UNSPECIFIED.);
#994=B_SPLINE_SURFACE_WITH_KNOTS('',5,1,((#34028,#34029),(#34030,#34031),
(#34032,#34033),(#34034,#34035),(#34036,#34037),(#34038,#34039),(#34040,
#34041),(#34042,#34043),(#34044,#34045),(#34046,#34047),(#34048,#34049),
(#34050,#34051),(#34052,#34053),(#34054,#34055),(#34056,#34057),(#34058,
#34059),(#34060,#34061),(#34062,#34063),(#34064,#34065),(#34066,#34067),
(#34068,#34069),(#34070,#34071),(#34072,#34073),(#34074,#34075),(#34076,
#34077),(#34078,#34079),(#34080,#34081),(#34082,#34083),(#34084,#34085),
(#34086,#34087),(#34088,#34089),(#34090,#34091),(#34092,#34093),(#34094,
#34095),(#34096,#34097),(#34098,#34099),(#34100,#34101),(#34102,#34103),
(#34104,#34105),(#34106,#34107),(#34108,#34109),(#34110,#34111),(#34112,
#34113),(#34114,#34115),(#34116,#34117),(#34118,#34119),(#34120,#34121),
(#34122,#34123),(#34124,#34125),(#34126,#34127),(#34128,#34129),(#34130,
#34131),(#34132,#34133),(#34134,#34135),(#34136,#34137),(#34138,#34139),
(#34140,#34141),(#34142,#34143),(#34144,#34145),(#34146,#34147),(#34148,
#34149),(#34150,#34151),(#34152,#34153),(#34154,#34155),(#34156,#34157),
(#34158,#34159),(#34160,#34161),(#34162,#34163),(#34164,#34165),(#34166,
#34167),(#34168,#34169),(#34170,#34171),(#34172,#34173),(#34174,#34175),
(#34176,#34177)),.UNSPECIFIED.,.F.,.F.,.F.,(6,1,1,1,1,1,1,1,1,1,1,1,1,1,
1,1,1,1,1,1,1,1,1,1,1,1,1,1,1,1,1,1,1,1,1,1,1,1,1,1,1,1,1,1,1,1,1,1,1,1,
1,1,1,1,1,1,1,1,1,1,1,1,1,1,1,1,1,1,1,1,6),(2,2),(0.,0.0142857142857143,
0.0285714285714286,0.0428571428571429,0.0571428571428571,0.0714285714285714,
0.0857142857142857,0.1,0.114285714285714,0.128571428571429,0.142857142857143,
0.157142857142857,0.171428571428571,0.185714285714286,0.2,0.214285714285714,
0.228571428571429,0.242857142857143,0.257142857142857,0.271428571428571,
0.285714285714286,0.3,0.314285714285714,0.328571428571429,0.342857142857143,
0.357142857142857,0.371428571428571,0.385714285714286,0.4,0.414285714285714,
0.428571428571429,0.442857142857143,0.457142857142857,0.471428571428572,
0.485714285714286,0.5,0.514285714285714,0.528571428571429,0.542857142857143,
0.557142857142857,0.571428571428571,0.585714285714286,0.6,0.614285714285714,
0.628571428571428,0.642857142857142,0.657142857142857,0.671428571428571,
0.685714285714285,0.699999999999999,0.714285714285714,0.728571428571428,
0.742857142857142,0.757142857142856,0.771428571428571,0.785714285714285,
0.799999999999999,0.814285714285713,0.828571428571428,0.842857142857142,
0.857142857142856,0.87142857142857,0.885714285714284,0.899999999999999,
0.914285714285713,0.928571428571427,0.942857142857141,0.957142857142856,
0.97142857142857,0.985714285714284,1.),(0.,1.8),.UNSPECIFIED.);
#995=B_SPLINE_SURFACE_WITH_KNOTS('',5,1,((#34326,#34327),(#34328,#34329),
(#34330,#34331),(#34332,#34333),(#34334,#34335),(#34336,#34337),(#34338,
#34339),(#34340,#34341),(#34342,#34343),(#34344,#34345),(#34346,#34347),
(#34348,#34349),(#34350,#34351),(#34352,#34353),(#34354,#34355),(#34356,
#34357),(#34358,#34359),(#34360,#34361),(#34362,#34363),(#34364,#34365),
(#34366,#34367),(#34368,#34369),(#34370,#34371),(#34372,#34373),(#34374,
#34375),(#34376,#34377),(#34378,#34379),(#34380,#34381),(#34382,#34383),
(#34384,#34385),(#34386,#34387),(#34388,#34389),(#34390,#34391),(#34392,
#34393),(#34394,#34395),(#34396,#34397),(#34398,#34399),(#34400,#34401),
(#34402,#34403),(#34404,#34405),(#34406,#34407),(#34408,#34409),(#34410,
#34411),(#34412,#34413),(#34414,#34415),(#34416,#34417),(#34418,#34419),
(#34420,#34421),(#34422,#34423),(#34424,#34425),(#34426,#34427),(#34428,
#34429),(#34430,#34431),(#34432,#34433),(#34434,#34435),(#34436,#34437),
(#34438,#34439),(#34440,#34441),(#34442,#34443),(#34444,#34445),(#34446,
#34447),(#34448,#34449),(#34450,#34451),(#34452,#34453),(#34454,#34455),
(#34456,#34457),(#34458,#34459),(#34460,#34461),(#34462,#34463),(#34464,
#34465),(#34466,#34467),(#34468,#34469),(#34470,#34471),(#34472,#34473),
(#34474,#34475)),.UNSPECIFIED.,.F.,.F.,.F.,(6,1,1,1,1,1,1,1,1,1,1,1,1,1,
1,1,1,1,1,1,1,1,1,1,1,1,1,1,1,1,1,1,1,1,1,1,1,1,1,1,1,1,1,1,1,1,1,1,1,1,
1,1,1,1,1,1,1,1,1,1,1,1,1,1,1,1,1,1,1,1,6),(2,2),(-1.,-0.985714285714284,
-0.97142857142857,-0.957142857142856,-0.942857142857141,-0.928571428571427,
-0.914285714285713,-0.899999999999999,-0.885714285714284,-0.87142857142857,
-0.857142857142856,-0.842857142857142,-0.828571428571428,-0.814285714285713,
-0.799999999999999,-0.785714285714285,-0.771428571428571,-0.757142857142856,
-0.742857142857142,-0.728571428571428,-0.714285714285714,-0.699999999999999,
-0.685714285714285,-0.671428571428571,-0.657142857142857,-0.642857142857142,
-0.628571428571428,-0.614285714285714,-0.6,-0.585714285714286,-0.571428571428571,
-0.557142857142857,-0.542857142857143,-0.528571428571429,-0.514285714285714,
-0.5,-0.485714285714286,-0.471428571428572,-0.457142857142857,-0.442857142857143,
-0.428571428571429,-0.414285714285714,-0.4,-0.385714285714286,-0.371428571428571,
-0.357142857142857,-0.342857142857143,-0.328571428571429,-0.314285714285714,
-0.3,-0.285714285714286,-0.271428571428571,-0.257142857142857,-0.242857142857143,
-0.228571428571429,-0.214285714285714,-0.2,-0.185714285714286,-0.171428571428571,
-0.157142857142857,-0.142857142857143,-0.128571428571429,-0.114285714285714,
-0.1,-0.0857142857142857,-0.0714285714285714,-0.0571428571428571,-0.0428571428571429,
-0.0285714285714286,-0.0142857142857143,0.),(0.,1.8),.UNSPECIFIED.);
#996=B_SPLINE_SURFACE_WITH_KNOTS('',5,1,((#34634,#34635),(#34636,#34637),
(#34638,#34639),(#34640,#34641),(#34642,#34643),(#34644,#34645),(#34646,
#34647),(#34648,#34649),(#34650,#34651),(#34652,#34653),(#34654,#34655),
(#34656,#34657),(#34658,#34659),(#34660,#34661),(#34662,#34663),(#34664,
#34665),(#34666,#34667),(#34668,#34669),(#34670,#34671),(#34672,#34673),
(#34674,#34675),(#34676,#34677),(#34678,#34679),(#34680,#34681),(#34682,
#34683),(#34684,#34685),(#34686,#34687),(#34688,#34689),(#34690,#34691),
(#34692,#34693),(#34694,#34695),(#34696,#34697),(#34698,#34699),(#34700,
#34701),(#34702,#34703),(#34704,#34705),(#34706,#34707),(#34708,#34709),
(#34710,#34711),(#34712,#34713),(#34714,#34715),(#34716,#34717),(#34718,
#34719),(#34720,#34721),(#34722,#34723),(#34724,#34725),(#34726,#34727),
(#34728,#34729),(#34730,#34731),(#34732,#34733),(#34734,#34735),(#34736,
#34737),(#34738,#34739),(#34740,#34741),(#34742,#34743),(#34744,#34745),
(#34746,#34747),(#34748,#34749),(#34750,#34751),(#34752,#34753),(#34754,
#34755),(#34756,#34757),(#34758,#34759),(#34760,#34761),(#34762,#34763),
(#34764,#34765),(#34766,#34767),(#34768,#34769),(#34770,#34771),(#34772,
#34773),(#34774,#34775),(#34776,#34777),(#34778,#34779),(#34780,#34781),
(#34782,#34783)),.UNSPECIFIED.,.F.,.F.,.F.,(6,1,1,1,1,1,1,1,1,1,1,1,1,1,
1,1,1,1,1,1,1,1,1,1,1,1,1,1,1,1,1,1,1,1,1,1,1,1,1,1,1,1,1,1,1,1,1,1,1,1,
1,1,1,1,1,1,1,1,1,1,1,1,1,1,1,1,1,1,1,1,6),(2,2),(0.,0.0142857142857143,
0.0285714285714286,0.0428571428571429,0.0571428571428571,0.0714285714285714,
0.0857142857142857,0.1,0.114285714285714,0.128571428571429,0.142857142857143,
0.157142857142857,0.171428571428571,0.185714285714286,0.2,0.214285714285714,
0.228571428571429,0.242857142857143,0.257142857142857,0.271428571428571,
0.285714285714286,0.3,0.314285714285714,0.328571428571429,0.342857142857143,
0.357142857142857,0.371428571428571,0.385714285714286,0.4,0.414285714285714,
0.428571428571429,0.442857142857143,0.457142857142857,0.471428571428572,
0.485714285714286,0.5,0.514285714285714,0.528571428571429,0.542857142857143,
0.557142857142857,0.571428571428571,0.585714285714286,0.6,0.614285714285714,
0.628571428571428,0.642857142857142,0.657142857142857,0.671428571428571,
0.685714285714285,0.699999999999999,0.714285714285714,0.728571428571428,
0.742857142857142,0.757142857142856,0.771428571428571,0.785714285714285,
0.799999999999999,0.814285714285713,0.828571428571428,0.842857142857142,
0.857142857142856,0.87142857142857,0.885714285714284,0.899999999999999,
0.914285714285713,0.928571428571427,0.942857142857141,0.957142857142856,
0.97142857142857,0.985714285714284,1.),(0.,1.8),.UNSPECIFIED.);
#997=B_SPLINE_SURFACE_WITH_KNOTS('',5,1,((#34932,#34933),(#34934,#34935),
(#34936,#34937),(#34938,#34939),(#34940,#34941),(#34942,#34943),(#34944,
#34945),(#34946,#34947),(#34948,#34949),(#34950,#34951),(#34952,#34953),
(#34954,#34955),(#34956,#34957),(#34958,#34959),(#34960,#34961),(#34962,
#34963),(#34964,#34965),(#34966,#34967),(#34968,#34969),(#34970,#34971),
(#34972,#34973),(#34974,#34975),(#34976,#34977),(#34978,#34979),(#34980,
#34981),(#34982,#34983),(#34984,#34985),(#34986,#34987),(#34988,#34989),
(#34990,#34991),(#34992,#34993),(#34994,#34995),(#34996,#34997),(#34998,
#34999),(#35000,#35001),(#35002,#35003),(#35004,#35005),(#35006,#35007),
(#35008,#35009),(#35010,#35011),(#35012,#35013),(#35014,#35015),(#35016,
#35017),(#35018,#35019),(#35020,#35021),(#35022,#35023),(#35024,#35025),
(#35026,#35027),(#35028,#35029),(#35030,#35031),(#35032,#35033),(#35034,
#35035),(#35036,#35037),(#35038,#35039),(#35040,#35041),(#35042,#35043),
(#35044,#35045),(#35046,#35047),(#35048,#35049),(#35050,#35051),(#35052,
#35053),(#35054,#35055),(#35056,#35057),(#35058,#35059),(#35060,#35061),
(#35062,#35063),(#35064,#35065),(#35066,#35067),(#35068,#35069),(#35070,
#35071),(#35072,#35073),(#35074,#35075),(#35076,#35077),(#35078,#35079),
(#35080,#35081)),.UNSPECIFIED.,.F.,.F.,.F.,(6,1,1,1,1,1,1,1,1,1,1,1,1,1,
1,1,1,1,1,1,1,1,1,1,1,1,1,1,1,1,1,1,1,1,1,1,1,1,1,1,1,1,1,1,1,1,1,1,1,1,
1,1,1,1,1,1,1,1,1,1,1,1,1,1,1,1,1,1,1,1,6),(2,2),(-1.,-0.985714285714284,
-0.97142857142857,-0.957142857142856,-0.942857142857141,-0.928571428571427,
-0.914285714285713,-0.899999999999999,-0.885714285714284,-0.87142857142857,
-0.857142857142856,-0.842857142857142,-0.828571428571428,-0.814285714285713,
-0.799999999999999,-0.785714285714285,-0.771428571428571,-0.757142857142856,
-0.742857142857142,-0.728571428571428,-0.714285714285714,-0.699999999999999,
-0.685714285714285,-0.671428571428571,-0.657142857142857,-0.642857142857142,
-0.628571428571428,-0.614285714285714,-0.6,-0.585714285714286,-0.571428571428571,
-0.557142857142857,-0.542857142857143,-0.528571428571429,-0.514285714285714,
-0.5,-0.485714285714286,-0.471428571428572,-0.457142857142857,-0.442857142857143,
-0.428571428571429,-0.414285714285714,-0.4,-0.385714285714286,-0.371428571428571,
-0.357142857142857,-0.342857142857143,-0.328571428571429,-0.314285714285714,
-0.3,-0.285714285714286,-0.271428571428571,-0.257142857142857,-0.242857142857143,
-0.228571428571429,-0.214285714285714,-0.2,-0.185714285714286,-0.171428571428571,
-0.157142857142857,-0.142857142857143,-0.128571428571429,-0.114285714285714,
-0.1,-0.0857142857142857,-0.0714285714285714,-0.0571428571428571,-0.0428571428571429,
-0.0285714285714286,-0.0142857142857143,0.),(0.,1.8),.UNSPECIFIED.);
#998=B_SPLINE_SURFACE_WITH_KNOTS('',5,1,((#35240,#35241),(#35242,#35243),
(#35244,#35245),(#35246,#35247),(#35248,#35249),(#35250,#35251),(#35252,
#35253),(#35254,#35255),(#35256,#35257),(#35258,#35259),(#35260,#35261),
(#35262,#35263),(#35264,#35265),(#35266,#35267),(#35268,#35269),(#35270,
#35271),(#35272,#35273),(#35274,#35275),(#35276,#35277),(#35278,#35279),
(#35280,#35281),(#35282,#35283),(#35284,#35285),(#35286,#35287),(#35288,
#35289),(#35290,#35291),(#35292,#35293),(#35294,#35295),(#35296,#35297),
(#35298,#35299),(#35300,#35301),(#35302,#35303),(#35304,#35305),(#35306,
#35307),(#35308,#35309),(#35310,#35311),(#35312,#35313),(#35314,#35315),
(#35316,#35317),(#35318,#35319),(#35320,#35321),(#35322,#35323),(#35324,
#35325),(#35326,#35327),(#35328,#35329),(#35330,#35331),(#35332,#35333),
(#35334,#35335),(#35336,#35337),(#35338,#35339),(#35340,#35341),(#35342,
#35343),(#35344,#35345),(#35346,#35347),(#35348,#35349),(#35350,#35351),
(#35352,#35353),(#35354,#35355),(#35356,#35357),(#35358,#35359),(#35360,
#35361),(#35362,#35363),(#35364,#35365),(#35366,#35367),(#35368,#35369),
(#35370,#35371),(#35372,#35373),(#35374,#35375),(#35376,#35377),(#35378,
#35379),(#35380,#35381),(#35382,#35383),(#35384,#35385),(#35386,#35387),
(#35388,#35389)),.UNSPECIFIED.,.F.,.F.,.F.,(6,1,1,1,1,1,1,1,1,1,1,1,1,1,
1,1,1,1,1,1,1,1,1,1,1,1,1,1,1,1,1,1,1,1,1,1,1,1,1,1,1,1,1,1,1,1,1,1,1,1,
1,1,1,1,1,1,1,1,1,1,1,1,1,1,1,1,1,1,1,1,6),(2,2),(0.,0.0142857142857143,
0.0285714285714286,0.0428571428571429,0.0571428571428571,0.0714285714285714,
0.0857142857142857,0.1,0.114285714285714,0.128571428571429,0.142857142857143,
0.157142857142857,0.171428571428571,0.185714285714286,0.2,0.214285714285714,
0.228571428571429,0.242857142857143,0.257142857142857,0.271428571428571,
0.285714285714286,0.3,0.314285714285714,0.328571428571429,0.342857142857143,
0.357142857142857,0.371428571428571,0.385714285714286,0.4,0.414285714285714,
0.428571428571429,0.442857142857143,0.457142857142857,0.471428571428572,
0.485714285714286,0.5,0.514285714285714,0.528571428571429,0.542857142857143,
0.557142857142857,0.571428571428571,0.585714285714286,0.6,0.614285714285714,
0.628571428571428,0.642857142857142,0.657142857142857,0.671428571428571,
0.685714285714285,0.699999999999999,0.714285714285714,0.728571428571428,
0.742857142857142,0.757142857142856,0.771428571428571,0.785714285714285,
0.799999999999999,0.814285714285713,0.828571428571428,0.842857142857142,
0.857142857142856,0.87142857142857,0.885714285714284,0.899999999999999,
0.914285714285713,0.928571428571427,0.942857142857141,0.957142857142856,
0.97142857142857,0.985714285714284,1.),(0.,1.8),.UNSPECIFIED.);
#999=B_SPLINE_SURFACE_WITH_KNOTS('',5,1,((#35538,#35539),(#35540,#35541),
(#35542,#35543),(#35544,#35545),(#35546,#35547),(#35548,#35549),(#35550,
#35551),(#35552,#35553),(#35554,#35555),(#35556,#35557),(#35558,#35559),
(#35560,#35561),(#35562,#35563),(#35564,#35565),(#35566,#35567),(#35568,
#35569),(#35570,#35571),(#35572,#35573),(#35574,#35575),(#35576,#35577),
(#35578,#35579),(#35580,#35581),(#35582,#35583),(#35584,#35585),(#35586,
#35587),(#35588,#35589),(#35590,#35591),(#35592,#35593),(#35594,#35595),
(#35596,#35597),(#35598,#35599),(#35600,#35601),(#35602,#35603),(#35604,
#35605),(#35606,#35607),(#35608,#35609),(#35610,#35611),(#35612,#35613),
(#35614,#35615),(#35616,#35617),(#35618,#35619),(#35620,#35621),(#35622,
#35623),(#35624,#35625),(#35626,#35627),(#35628,#35629),(#35630,#35631),
(#35632,#35633),(#35634,#35635),(#35636,#35637),(#35638,#35639),(#35640,
#35641),(#35642,#35643),(#35644,#35645),(#35646,#35647),(#35648,#35649),
(#35650,#35651),(#35652,#35653),(#35654,#35655),(#35656,#35657),(#35658,
#35659),(#35660,#35661),(#35662,#35663),(#35664,#35665),(#35666,#35667),
(#35668,#35669),(#35670,#35671),(#35672,#35673),(#35674,#35675),(#35676,
#35677),(#35678,#35679),(#35680,#35681),(#35682,#35683),(#35684,#35685),
(#35686,#35687)),.UNSPECIFIED.,.F.,.F.,.F.,(6,1,1,1,1,1,1,1,1,1,1,1,1,1,
1,1,1,1,1,1,1,1,1,1,1,1,1,1,1,1,1,1,1,1,1,1,1,1,1,1,1,1,1,1,1,1,1,1,1,1,
1,1,1,1,1,1,1,1,1,1,1,1,1,1,1,1,1,1,1,1,6),(2,2),(-1.,-0.985714285714284,
-0.97142857142857,-0.957142857142856,-0.942857142857141,-0.928571428571427,
-0.914285714285713,-0.899999999999999,-0.885714285714284,-0.87142857142857,
-0.857142857142856,-0.842857142857142,-0.828571428571428,-0.814285714285713,
-0.799999999999999,-0.785714285714285,-0.771428571428571,-0.757142857142856,
-0.742857142857142,-0.728571428571428,-0.714285714285714,-0.699999999999999,
-0.685714285714285,-0.671428571428571,-0.657142857142857,-0.642857142857142,
-0.628571428571428,-0.614285714285714,-0.6,-0.585714285714286,-0.571428571428571,
-0.557142857142857,-0.542857142857143,-0.528571428571429,-0.514285714285714,
-0.5,-0.485714285714286,-0.471428571428572,-0.457142857142857,-0.442857142857143,
-0.428571428571429,-0.414285714285714,-0.4,-0.385714285714286,-0.371428571428571,
-0.357142857142857,-0.342857142857143,-0.328571428571429,-0.314285714285714,
-0.3,-0.285714285714286,-0.271428571428571,-0.257142857142857,-0.242857142857143,
-0.228571428571429,-0.214285714285714,-0.2,-0.185714285714286,-0.171428571428571,
-0.157142857142857,-0.142857142857143,-0.128571428571429,-0.114285714285714,
-0.1,-0.0857142857142857,-0.0714285714285714,-0.0571428571428571,-0.0428571428571429,
-0.0285714285714286,-0.0142857142857143,0.),(0.,1.8),.UNSPECIFIED.);
#1000=B_SPLINE_SURFACE_WITH_KNOTS('',5,1,((#35846,#35847),(#35848,#35849),
(#35850,#35851),(#35852,#35853),(#35854,#35855),(#35856,#35857),(#35858,
#35859),(#35860,#35861),(#35862,#35863),(#35864,#35865),(#35866,#35867),
(#35868,#35869),(#35870,#35871),(#35872,#35873),(#35874,#35875),(#35876,
#35877),(#35878,#35879),(#35880,#35881),(#35882,#35883),(#35884,#35885),
(#35886,#35887),(#35888,#35889),(#35890,#35891),(#35892,#35893),(#35894,
#35895),(#35896,#35897),(#35898,#35899),(#35900,#35901),(#35902,#35903),
(#35904,#35905),(#35906,#35907),(#35908,#35909),(#35910,#35911),(#35912,
#35913),(#35914,#35915),(#35916,#35917),(#35918,#35919),(#35920,#35921),
(#35922,#35923),(#35924,#35925),(#35926,#35927),(#35928,#35929),(#35930,
#35931),(#35932,#35933),(#35934,#35935),(#35936,#35937),(#35938,#35939),
(#35940,#35941),(#35942,#35943),(#35944,#35945),(#35946,#35947),(#35948,
#35949),(#35950,#35951),(#35952,#35953),(#35954,#35955),(#35956,#35957),
(#35958,#35959),(#35960,#35961),(#35962,#35963),(#35964,#35965),(#35966,
#35967),(#35968,#35969),(#35970,#35971),(#35972,#35973),(#35974,#35975),
(#35976,#35977),(#35978,#35979),(#35980,#35981),(#35982,#35983),(#35984,
#35985),(#35986,#35987),(#35988,#35989),(#35990,#35991),(#35992,#35993),
(#35994,#35995)),.UNSPECIFIED.,.F.,.F.,.F.,(6,1,1,1,1,1,1,1,1,1,1,1,1,1,
1,1,1,1,1,1,1,1,1,1,1,1,1,1,1,1,1,1,1,1,1,1,1,1,1,1,1,1,1,1,1,1,1,1,1,1,
1,1,1,1,1,1,1,1,1,1,1,1,1,1,1,1,1,1,1,1,6),(2,2),(0.,0.0142857142857143,
0.0285714285714286,0.0428571428571429,0.0571428571428571,0.0714285714285714,
0.0857142857142857,0.1,0.114285714285714,0.128571428571429,0.142857142857143,
0.157142857142857,0.171428571428571,0.185714285714286,0.2,0.214285714285714,
0.228571428571429,0.242857142857143,0.257142857142857,0.271428571428571,
0.285714285714286,0.3,0.314285714285714,0.328571428571429,0.342857142857143,
0.357142857142857,0.371428571428571,0.385714285714286,0.4,0.414285714285714,
0.428571428571429,0.442857142857143,0.457142857142857,0.471428571428572,
0.485714285714286,0.5,0.514285714285714,0.528571428571429,0.542857142857143,
0.557142857142857,0.571428571428571,0.585714285714286,0.6,0.614285714285714,
0.628571428571428,0.642857142857142,0.657142857142857,0.671428571428571,
0.685714285714285,0.699999999999999,0.714285714285714,0.728571428571428,
0.742857142857142,0.757142857142856,0.771428571428571,0.785714285714285,
0.799999999999999,0.814285714285713,0.828571428571428,0.842857142857142,
0.857142857142856,0.87142857142857,0.885714285714284,0.899999999999999,
0.914285714285713,0.928571428571427,0.942857142857141,0.957142857142856,
0.97142857142857,0.985714285714284,1.),(0.,1.8),.UNSPECIFIED.);
#1001=B_SPLINE_SURFACE_WITH_KNOTS('',5,1,((#36144,#36145),(#36146,#36147),
(#36148,#36149),(#36150,#36151),(#36152,#36153),(#36154,#36155),(#36156,
#36157),(#36158,#36159),(#36160,#36161),(#36162,#36163),(#36164,#36165),
(#36166,#36167),(#36168,#36169),(#36170,#36171),(#36172,#36173),(#36174,
#36175),(#36176,#36177),(#36178,#36179),(#36180,#36181),(#36182,#36183),
(#36184,#36185),(#36186,#36187),(#36188,#36189),(#36190,#36191),(#36192,
#36193),(#36194,#36195),(#36196,#36197),(#36198,#36199),(#36200,#36201),
(#36202,#36203),(#36204,#36205),(#36206,#36207),(#36208,#36209),(#36210,
#36211),(#36212,#36213),(#36214,#36215),(#36216,#36217),(#36218,#36219),
(#36220,#36221),(#36222,#36223),(#36224,#36225),(#36226,#36227),(#36228,
#36229),(#36230,#36231),(#36232,#36233),(#36234,#36235),(#36236,#36237),
(#36238,#36239),(#36240,#36241),(#36242,#36243),(#36244,#36245),(#36246,
#36247),(#36248,#36249),(#36250,#36251),(#36252,#36253),(#36254,#36255),
(#36256,#36257),(#36258,#36259),(#36260,#36261),(#36262,#36263),(#36264,
#36265),(#36266,#36267),(#36268,#36269),(#36270,#36271),(#36272,#36273),
(#36274,#36275),(#36276,#36277),(#36278,#36279),(#36280,#36281),(#36282,
#36283),(#36284,#36285),(#36286,#36287),(#36288,#36289),(#36290,#36291),
(#36292,#36293)),.UNSPECIFIED.,.F.,.F.,.F.,(6,1,1,1,1,1,1,1,1,1,1,1,1,1,
1,1,1,1,1,1,1,1,1,1,1,1,1,1,1,1,1,1,1,1,1,1,1,1,1,1,1,1,1,1,1,1,1,1,1,1,
1,1,1,1,1,1,1,1,1,1,1,1,1,1,1,1,1,1,1,1,6),(2,2),(-1.,-0.985714285714284,
-0.97142857142857,-0.957142857142856,-0.942857142857141,-0.928571428571427,
-0.914285714285713,-0.899999999999999,-0.885714285714284,-0.87142857142857,
-0.857142857142856,-0.842857142857142,-0.828571428571428,-0.814285714285713,
-0.799999999999999,-0.785714285714285,-0.771428571428571,-0.757142857142856,
-0.742857142857142,-0.728571428571428,-0.714285714285714,-0.699999999999999,
-0.685714285714285,-0.671428571428571,-0.657142857142857,-0.642857142857142,
-0.628571428571428,-0.614285714285714,-0.6,-0.585714285714286,-0.571428571428571,
-0.557142857142857,-0.542857142857143,-0.528571428571429,-0.514285714285714,
-0.5,-0.485714285714286,-0.471428571428572,-0.457142857142857,-0.442857142857143,
-0.428571428571429,-0.414285714285714,-0.4,-0.385714285714286,-0.371428571428571,
-0.357142857142857,-0.342857142857143,-0.328571428571429,-0.314285714285714,
-0.3,-0.285714285714286,-0.271428571428571,-0.257142857142857,-0.242857142857143,
-0.228571428571429,-0.214285714285714,-0.2,-0.185714285714286,-0.171428571428571,
-0.157142857142857,-0.142857142857143,-0.128571428571429,-0.114285714285714,
-0.1,-0.0857142857142857,-0.0714285714285714,-0.0571428571428571,-0.0428571428571429,
-0.0285714285714286,-0.0142857142857143,0.),(0.,1.8),.UNSPECIFIED.);
#1002=B_SPLINE_SURFACE_WITH_KNOTS('',5,1,((#36452,#36453),(#36454,#36455),
(#36456,#36457),(#36458,#36459),(#36460,#36461),(#36462,#36463),(#36464,
#36465),(#36466,#36467),(#36468,#36469),(#36470,#36471),(#36472,#36473),
(#36474,#36475),(#36476,#36477),(#36478,#36479),(#36480,#36481),(#36482,
#36483),(#36484,#36485),(#36486,#36487),(#36488,#36489),(#36490,#36491),
(#36492,#36493),(#36494,#36495),(#36496,#36497),(#36498,#36499),(#36500,
#36501),(#36502,#36503),(#36504,#36505),(#36506,#36507),(#36508,#36509),
(#36510,#36511),(#36512,#36513),(#36514,#36515),(#36516,#36517),(#36518,
#36519),(#36520,#36521),(#36522,#36523),(#36524,#36525),(#36526,#36527),
(#36528,#36529),(#36530,#36531),(#36532,#36533),(#36534,#36535),(#36536,
#36537),(#36538,#36539),(#36540,#36541),(#36542,#36543),(#36544,#36545),
(#36546,#36547),(#36548,#36549),(#36550,#36551),(#36552,#36553),(#36554,
#36555),(#36556,#36557),(#36558,#36559),(#36560,#36561),(#36562,#36563),
(#36564,#36565),(#36566,#36567),(#36568,#36569),(#36570,#36571),(#36572,
#36573),(#36574,#36575),(#36576,#36577),(#36578,#36579),(#36580,#36581),
(#36582,#36583),(#36584,#36585),(#36586,#36587),(#36588,#36589),(#36590,
#36591),(#36592,#36593),(#36594,#36595),(#36596,#36597),(#36598,#36599),
(#36600,#36601)),.UNSPECIFIED.,.F.,.F.,.F.,(6,1,1,1,1,1,1,1,1,1,1,1,1,1,
1,1,1,1,1,1,1,1,1,1,1,1,1,1,1,1,1,1,1,1,1,1,1,1,1,1,1,1,1,1,1,1,1,1,1,1,
1,1,1,1,1,1,1,1,1,1,1,1,1,1,1,1,1,1,1,1,6),(2,2),(0.,0.0142857142857143,
0.0285714285714286,0.0428571428571429,0.0571428571428571,0.0714285714285714,
0.0857142857142857,0.1,0.114285714285714,0.128571428571429,0.142857142857143,
0.157142857142857,0.171428571428571,0.185714285714286,0.2,0.214285714285714,
0.228571428571429,0.242857142857143,0.257142857142857,0.271428571428571,
0.285714285714286,0.3,0.314285714285714,0.328571428571429,0.342857142857143,
0.357142857142857,0.371428571428571,0.385714285714286,0.4,0.414285714285714,
0.428571428571429,0.442857142857143,0.457142857142857,0.471428571428572,
0.485714285714286,0.5,0.514285714285714,0.528571428571429,0.542857142857143,
0.557142857142857,0.571428571428571,0.585714285714286,0.6,0.614285714285714,
0.628571428571428,0.642857142857142,0.657142857142857,0.671428571428571,
0.685714285714285,0.699999999999999,0.714285714285714,0.728571428571428,
0.742857142857142,0.757142857142856,0.771428571428571,0.785714285714285,
0.799999999999999,0.814285714285713,0.828571428571428,0.842857142857142,
0.857142857142856,0.87142857142857,0.885714285714284,0.899999999999999,
0.914285714285713,0.928571428571427,0.942857142857141,0.957142857142856,
0.97142857142857,0.985714285714284,1.),(0.,1.8),.UNSPECIFIED.);
#1003=B_SPLINE_SURFACE_WITH_KNOTS('',5,1,((#36750,#36751),(#36752,#36753),
(#36754,#36755),(#36756,#36757),(#36758,#36759),(#36760,#36761),(#36762,
#36763),(#36764,#36765),(#36766,#36767),(#36768,#36769),(#36770,#36771),
(#36772,#36773),(#36774,#36775),(#36776,#36777),(#36778,#36779),(#36780,
#36781),(#36782,#36783),(#36784,#36785),(#36786,#36787),(#36788,#36789),
(#36790,#36791),(#36792,#36793),(#36794,#36795),(#36796,#36797),(#36798,
#36799),(#36800,#36801),(#36802,#36803),(#36804,#36805),(#36806,#36807),
(#36808,#36809),(#36810,#36811),(#36812,#36813),(#36814,#36815),(#36816,
#36817),(#36818,#36819),(#36820,#36821),(#36822,#36823),(#36824,#36825),
(#36826,#36827),(#36828,#36829),(#36830,#36831),(#36832,#36833),(#36834,
#36835),(#36836,#36837),(#36838,#36839),(#36840,#36841),(#36842,#36843),
(#36844,#36845),(#36846,#36847),(#36848,#36849),(#36850,#36851),(#36852,
#36853),(#36854,#36855),(#36856,#36857),(#36858,#36859),(#36860,#36861),
(#36862,#36863),(#36864,#36865),(#36866,#36867),(#36868,#36869),(#36870,
#36871),(#36872,#36873),(#36874,#36875),(#36876,#36877),(#36878,#36879),
(#36880,#36881),(#36882,#36883),(#36884,#36885),(#36886,#36887),(#36888,
#36889),(#36890,#36891),(#36892,#36893),(#36894,#36895),(#36896,#36897),
(#36898,#36899)),.UNSPECIFIED.,.F.,.F.,.F.,(6,1,1,1,1,1,1,1,1,1,1,1,1,1,
1,1,1,1,1,1,1,1,1,1,1,1,1,1,1,1,1,1,1,1,1,1,1,1,1,1,1,1,1,1,1,1,1,1,1,1,
1,1,1,1,1,1,1,1,1,1,1,1,1,1,1,1,1,1,1,1,6),(2,2),(-1.,-0.985714285714284,
-0.97142857142857,-0.957142857142856,-0.942857142857141,-0.928571428571427,
-0.914285714285713,-0.899999999999999,-0.885714285714284,-0.87142857142857,
-0.857142857142856,-0.842857142857142,-0.828571428571428,-0.814285714285713,
-0.799999999999999,-0.785714285714285,-0.771428571428571,-0.757142857142856,
-0.742857142857142,-0.728571428571428,-0.714285714285714,-0.699999999999999,
-0.685714285714285,-0.671428571428571,-0.657142857142857,-0.642857142857142,
-0.628571428571428,-0.614285714285714,-0.6,-0.585714285714286,-0.571428571428571,
-0.557142857142857,-0.542857142857143,-0.528571428571429,-0.514285714285714,
-0.5,-0.485714285714286,-0.471428571428572,-0.457142857142857,-0.442857142857143,
-0.428571428571429,-0.414285714285714,-0.4,-0.385714285714286,-0.371428571428571,
-0.357142857142857,-0.342857142857143,-0.328571428571429,-0.314285714285714,
-0.3,-0.285714285714286,-0.271428571428571,-0.257142857142857,-0.242857142857143,
-0.228571428571429,-0.214285714285714,-0.2,-0.185714285714286,-0.171428571428571,
-0.157142857142857,-0.142857142857143,-0.128571428571429,-0.114285714285714,
-0.1,-0.0857142857142857,-0.0714285714285714,-0.0571428571428571,-0.0428571428571429,
-0.0285714285714286,-0.0142857142857143,0.),(0.,1.8),.UNSPECIFIED.);
#1004=B_SPLINE_SURFACE_WITH_KNOTS('',5,1,((#37058,#37059),(#37060,#37061),
(#37062,#37063),(#37064,#37065),(#37066,#37067),(#37068,#37069),(#37070,
#37071),(#37072,#37073),(#37074,#37075),(#37076,#37077),(#37078,#37079),
(#37080,#37081),(#37082,#37083),(#37084,#37085),(#37086,#37087),(#37088,
#37089),(#37090,#37091),(#37092,#37093),(#37094,#37095),(#37096,#37097),
(#37098,#37099),(#37100,#37101),(#37102,#37103),(#37104,#37105),(#37106,
#37107),(#37108,#37109),(#37110,#37111),(#37112,#37113),(#37114,#37115),
(#37116,#37117),(#37118,#37119),(#37120,#37121),(#37122,#37123),(#37124,
#37125),(#37126,#37127),(#37128,#37129),(#37130,#37131),(#37132,#37133),
(#37134,#37135),(#37136,#37137),(#37138,#37139),(#37140,#37141),(#37142,
#37143),(#37144,#37145),(#37146,#37147),(#37148,#37149),(#37150,#37151),
(#37152,#37153),(#37154,#37155),(#37156,#37157),(#37158,#37159),(#37160,
#37161),(#37162,#37163),(#37164,#37165),(#37166,#37167),(#37168,#37169),
(#37170,#37171),(#37172,#37173),(#37174,#37175),(#37176,#37177),(#37178,
#37179),(#37180,#37181),(#37182,#37183),(#37184,#37185),(#37186,#37187),
(#37188,#37189),(#37190,#37191),(#37192,#37193),(#37194,#37195),(#37196,
#37197),(#37198,#37199),(#37200,#37201),(#37202,#37203),(#37204,#37205),
(#37206,#37207)),.UNSPECIFIED.,.F.,.F.,.F.,(6,1,1,1,1,1,1,1,1,1,1,1,1,1,
1,1,1,1,1,1,1,1,1,1,1,1,1,1,1,1,1,1,1,1,1,1,1,1,1,1,1,1,1,1,1,1,1,1,1,1,
1,1,1,1,1,1,1,1,1,1,1,1,1,1,1,1,1,1,1,1,6),(2,2),(0.,0.0142857142857143,
0.0285714285714286,0.0428571428571429,0.0571428571428571,0.0714285714285714,
0.0857142857142857,0.1,0.114285714285714,0.128571428571429,0.142857142857143,
0.157142857142857,0.171428571428571,0.185714285714286,0.2,0.214285714285714,
0.228571428571429,0.242857142857143,0.257142857142857,0.271428571428571,
0.285714285714286,0.3,0.314285714285714,0.328571428571429,0.342857142857143,
0.357142857142857,0.371428571428571,0.385714285714286,0.4,0.414285714285714,
0.428571428571429,0.442857142857143,0.457142857142857,0.471428571428572,
0.485714285714286,0.5,0.514285714285714,0.528571428571429,0.542857142857143,
0.557142857142857,0.571428571428571,0.585714285714286,0.6,0.614285714285714,
0.628571428571428,0.642857142857142,0.657142857142857,0.671428571428571,
0.685714285714285,0.699999999999999,0.714285714285714,0.728571428571428,
0.742857142857142,0.757142857142856,0.771428571428571,0.785714285714285,
0.799999999999999,0.814285714285713,0.828571428571428,0.842857142857142,
0.857142857142856,0.87142857142857,0.885714285714284,0.899999999999999,
0.914285714285713,0.928571428571427,0.942857142857141,0.957142857142856,
0.97142857142857,0.985714285714284,1.),(0.,1.8),.UNSPECIFIED.);
#1005=B_SPLINE_SURFACE_WITH_KNOTS('',5,1,((#37720,#37721),(#37722,#37723),
(#37724,#37725),(#37726,#37727),(#37728,#37729),(#37730,#37731),(#37732,
#37733),(#37734,#37735),(#37736,#37737),(#37738,#37739),(#37740,#37741),
(#37742,#37743),(#37744,#37745),(#37746,#37747),(#37748,#37749),(#37750,
#37751),(#37752,#37753),(#37754,#37755),(#37756,#37757),(#37758,#37759),
(#37760,#37761),(#37762,#37763),(#37764,#37765),(#37766,#37767),(#37768,
#37769),(#37770,#37771),(#37772,#37773),(#37774,#37775),(#37776,#37777),
(#37778,#37779),(#37780,#37781),(#37782,#37783),(#37784,#37785),(#37786,
#37787),(#37788,#37789),(#37790,#37791),(#37792,#37793),(#37794,#37795),
(#37796,#37797),(#37798,#37799),(#37800,#37801),(#37802,#37803),(#37804,
#37805),(#37806,#37807),(#37808,#37809),(#37810,#37811),(#37812,#37813),
(#37814,#37815),(#37816,#37817),(#37818,#37819),(#37820,#37821),(#37822,
#37823),(#37824,#37825),(#37826,#37827),(#37828,#37829),(#37830,#37831),
(#37832,#37833),(#37834,#37835),(#37836,#37837),(#37838,#37839),(#37840,
#37841),(#37842,#37843),(#37844,#37845),(#37846,#37847),(#37848,#37849),
(#37850,#37851),(#37852,#37853),(#37854,#37855),(#37856,#37857),(#37858,
#37859),(#37860,#37861),(#37862,#37863),(#37864,#37865),(#37866,#37867),
(#37868,#37869)),.UNSPECIFIED.,.F.,.F.,.F.,(6,1,1,1,1,1,1,1,1,1,1,1,1,1,
1,1,1,1,1,1,1,1,1,1,1,1,1,1,1,1,1,1,1,1,1,1,1,1,1,1,1,1,1,1,1,1,1,1,1,1,
1,1,1,1,1,1,1,1,1,1,1,1,1,1,1,1,1,1,1,1,6),(2,2),(-1.,-0.985714285714284,
-0.97142857142857,-0.957142857142856,-0.942857142857141,-0.928571428571427,
-0.914285714285713,-0.899999999999999,-0.885714285714284,-0.87142857142857,
-0.857142857142856,-0.842857142857142,-0.828571428571428,-0.814285714285713,
-0.799999999999999,-0.785714285714285,-0.771428571428571,-0.757142857142856,
-0.742857142857142,-0.728571428571428,-0.714285714285714,-0.699999999999999,
-0.685714285714285,-0.671428571428571,-0.657142857142857,-0.642857142857142,
-0.628571428571428,-0.614285714285714,-0.6,-0.585714285714286,-0.571428571428571,
-0.557142857142857,-0.542857142857143,-0.528571428571429,-0.514285714285714,
-0.5,-0.485714285714286,-0.471428571428572,-0.457142857142857,-0.442857142857143,
-0.428571428571429,-0.414285714285714,-0.4,-0.385714285714286,-0.371428571428571,
-0.357142857142857,-0.342857142857143,-0.328571428571429,-0.314285714285714,
-0.3,-0.285714285714286,-0.271428571428571,-0.257142857142857,-0.242857142857143,
-0.228571428571429,-0.214285714285714,-0.2,-0.185714285714286,-0.171428571428571,
-0.157142857142857,-0.142857142857143,-0.128571428571429,-0.114285714285714,
-0.1,-0.0857142857142857,-0.0714285714285714,-0.0571428571428571,-0.0428571428571429,
-0.0285714285714286,-0.0142857142857143,0.),(0.,1.8),.UNSPECIFIED.);
#1006=B_SPLINE_SURFACE_WITH_KNOTS('',5,1,((#37873,#37874),(#37875,#37876),
(#37877,#37878),(#37879,#37880),(#37881,#37882),(#37883,#37884),(#37885,
#37886),(#37887,#37888),(#37889,#37890),(#37891,#37892),(#37893,#37894),
(#37895,#37896),(#37897,#37898),(#37899,#37900),(#37901,#37902),(#37903,
#37904),(#37905,#37906),(#37907,#37908),(#37909,#37910),(#37911,#37912),
(#37913,#37914),(#37915,#37916),(#37917,#37918),(#37919,#37920),(#37921,
#37922),(#37923,#37924),(#37925,#37926),(#37927,#37928),(#37929,#37930),
(#37931,#37932),(#37933,#37934),(#37935,#37936),(#37937,#37938),(#37939,
#37940),(#37941,#37942),(#37943,#37944),(#37945,#37946),(#37947,#37948),
(#37949,#37950),(#37951,#37952),(#37953,#37954),(#37955,#37956),(#37957,
#37958),(#37959,#37960),(#37961,#37962),(#37963,#37964),(#37965,#37966),
(#37967,#37968),(#37969,#37970),(#37971,#37972),(#37973,#37974),(#37975,
#37976),(#37977,#37978),(#37979,#37980),(#37981,#37982),(#37983,#37984),
(#37985,#37986),(#37987,#37988),(#37989,#37990),(#37991,#37992),(#37993,
#37994),(#37995,#37996),(#37997,#37998),(#37999,#38000),(#38001,#38002),
(#38003,#38004),(#38005,#38006),(#38007,#38008),(#38009,#38010),(#38011,
#38012),(#38013,#38014),(#38015,#38016),(#38017,#38018),(#38019,#38020),
(#38021,#38022)),.UNSPECIFIED.,.F.,.F.,.F.,(6,1,1,1,1,1,1,1,1,1,1,1,1,1,
1,1,1,1,1,1,1,1,1,1,1,1,1,1,1,1,1,1,1,1,1,1,1,1,1,1,1,1,1,1,1,1,1,1,1,1,
1,1,1,1,1,1,1,1,1,1,1,1,1,1,1,1,1,1,1,1,6),(2,2),(0.,0.0142857142857143,
0.0285714285714286,0.0428571428571429,0.0571428571428571,0.0714285714285714,
0.0857142857142857,0.1,0.114285714285714,0.128571428571429,0.142857142857143,
0.157142857142857,0.171428571428571,0.185714285714286,0.2,0.214285714285714,
0.228571428571429,0.242857142857143,0.257142857142857,0.271428571428571,
0.285714285714286,0.3,0.314285714285714,0.328571428571429,0.342857142857143,
0.357142857142857,0.371428571428571,0.385714285714286,0.4,0.414285714285714,
0.428571428571429,0.442857142857143,0.457142857142857,0.471428571428572,
0.485714285714286,0.5,0.514285714285714,0.528571428571429,0.542857142857143,
0.557142857142857,0.571428571428571,0.585714285714286,0.6,0.614285714285714,
0.628571428571428,0.642857142857142,0.657142857142857,0.671428571428571,
0.685714285714285,0.699999999999999,0.714285714285714,0.728571428571428,
0.742857142857142,0.757142857142856,0.771428571428571,0.785714285714285,
0.799999999999999,0.814285714285713,0.828571428571428,0.842857142857142,
0.857142857142856,0.87142857142857,0.885714285714284,0.899999999999999,
0.914285714285713,0.928571428571427,0.942857142857141,0.957142857142856,
0.97142857142857,0.985714285714284,1.),(0.,1.8),.UNSPECIFIED.);
#1051=PLANE('',#13483);
#1052=PLANE('',#13484);
#1053=PLANE('',#13488);
#1054=PLANE('',#13492);
#1055=PLANE('',#13496);
#1056=PLANE('',#13500);
#1057=PLANE('',#13504);
#1058=PLANE('',#13508);
#1059=PLANE('',#13512);
#1060=PLANE('',#13516);
#1061=PLANE('',#13520);
#1062=PLANE('',#13524);
#1063=PLANE('',#13528);
#1064=PLANE('',#13532);
#1065=PLANE('',#13536);
#1066=PLANE('',#13540);
#1067=PLANE('',#13544);
#1068=PLANE('',#13548);
#1069=PLANE('',#13552);
#1070=PLANE('',#13556);
#1071=PLANE('',#13584);
#1072=PLANE('',#13598);
#1073=PLANE('',#13622);
#1074=PLANE('',#13624);
#1453=FACE_OUTER_BOUND('',#2207,.T.);
#1454=FACE_OUTER_BOUND('',#2208,.T.);
#1455=FACE_OUTER_BOUND('',#2209,.T.);
#1456=FACE_OUTER_BOUND('',#2210,.T.);
#1457=FACE_OUTER_BOUND('',#2211,.T.);
#1458=FACE_OUTER_BOUND('',#2212,.T.);
#1459=FACE_OUTER_BOUND('',#2213,.T.);
#1460=FACE_OUTER_BOUND('',#2214,.T.);
#1461=FACE_OUTER_BOUND('',#2215,.T.);
#1462=FACE_OUTER_BOUND('',#2216,.T.);
#1463=FACE_OUTER_BOUND('',#2217,.T.);
#1464=FACE_OUTER_BOUND('',#2218,.T.);
#1465=FACE_OUTER_BOUND('',#2219,.T.);
#1466=FACE_OUTER_BOUND('',#2220,.T.);
#1467=FACE_OUTER_BOUND('',#2221,.T.);
#1468=FACE_OUTER_BOUND('',#2222,.T.);
#1469=FACE_OUTER_BOUND('',#2223,.T.);
#1470=FACE_OUTER_BOUND('',#2224,.T.);
#1471=FACE_OUTER_BOUND('',#2225,.T.);
#1472=FACE_OUTER_BOUND('',#2226,.T.);
#1473=FACE_OUTER_BOUND('',#2227,.T.);
#1474=FACE_OUTER_BOUND('',#2228,.T.);
#1475=FACE_OUTER_BOUND('',#2229,.T.);
#1476=FACE_OUTER_BOUND('',#2230,.T.);
#1477=FACE_OUTER_BOUND('',#2231,.T.);
#1478=FACE_OUTER_BOUND('',#2232,.T.);
#1479=FACE_OUTER_BOUND('',#2233,.T.);
#1480=FACE_OUTER_BOUND('',#2234,.T.);
#1481=FACE_OUTER_BOUND('',#2235,.T.);
#1482=FACE_OUTER_BOUND('',#2236,.T.);
#1483=FACE_OUTER_BOUND('',#2237,.T.);
#1484=FACE_OUTER_BOUND('',#2238,.T.);
#1485=FACE_OUTER_BOUND('',#2239,.T.);
#1486=FACE_OUTER_BOUND('',#2240,.T.);
#1487=FACE_OUTER_BOUND('',#2241,.T.);
#1488=FACE_OUTER_BOUND('',#2242,.T.);
#1489=FACE_OUTER_BOUND('',#2243,.T.);
#1490=FACE_OUTER_BOUND('',#2244,.T.);
#1491=FACE_OUTER_BOUND('',#2245,.T.);
#1492=FACE_OUTER_BOUND('',#2246,.T.);
#1493=FACE_OUTER_BOUND('',#2247,.T.);
#1494=FACE_OUTER_BOUND('',#2248,.T.);
#1495=FACE_OUTER_BOUND('',#2249,.T.);
#1496=FACE_OUTER_BOUND('',#2250,.T.);
#1497=FACE_OUTER_BOUND('',#2251,.T.);
#1498=FACE_OUTER_BOUND('',#2252,.T.);
#1499=FACE_OUTER_BOUND('',#2253,.T.);
#1500=FACE_OUTER_BOUND('',#2254,.T.);
#1501=FACE_OUTER_BOUND('',#2255,.T.);
#1502=FACE_OUTER_BOUND('',#2256,.T.);
#1503=FACE_OUTER_BOUND('',#2257,.T.);
#1504=FACE_OUTER_BOUND('',#2258,.T.);
#1505=FACE_OUTER_BOUND('',#2259,.T.);
#1506=FACE_OUTER_BOUND('',#2260,.T.);
#1507=FACE_OUTER_BOUND('',#2261,.T.);
#1508=FACE_OUTER_BOUND('',#2262,.T.);
#1509=FACE_OUTER_BOUND('',#2263,.T.);
#1510=FACE_OUTER_BOUND('',#2264,.T.);
#1511=FACE_OUTER_BOUND('',#2265,.T.);
#1512=FACE_OUTER_BOUND('',#2266,.T.);
#1513=FACE_OUTER_BOUND('',#2267,.T.);
#1514=FACE_OUTER_BOUND('',#2268,.T.);
#1515=FACE_OUTER_BOUND('',#2269,.T.);
#1516=FACE_OUTER_BOUND('',#2270,.T.);
#1517=FACE_OUTER_BOUND('',#2271,.T.);
#1518=FACE_OUTER_BOUND('',#2272,.T.);
#1519=FACE_OUTER_BOUND('',#2273,.T.);
#1520=FACE_OUTER_BOUND('',#2274,.T.);
#1521=FACE_OUTER_BOUND('',#2276,.T.);
#1522=FACE_OUTER_BOUND('',#2278,.T.);
#1523=FACE_OUTER_BOUND('',#2279,.T.);
#1524=FACE_OUTER_BOUND('',#2280,.T.);
#1525=FACE_OUTER_BOUND('',#2281,.T.);
#1526=FACE_OUTER_BOUND('',#2282,.T.);
#1527=FACE_OUTER_BOUND('',#2283,.T.);
#1528=FACE_OUTER_BOUND('',#2284,.T.);
#1529=FACE_OUTER_BOUND('',#2285,.T.);
#1530=FACE_OUTER_BOUND('',#2286,.T.);
#1531=FACE_OUTER_BOUND('',#2287,.T.);
#1532=FACE_OUTER_BOUND('',#2288,.T.);
#1533=FACE_OUTER_BOUND('',#2289,.T.);
#1534=FACE_OUTER_BOUND('',#2290,.T.);
#1535=FACE_OUTER_BOUND('',#2291,.T.);
#1536=FACE_OUTER_BOUND('',#2292,.T.);
#1537=FACE_OUTER_BOUND('',#2293,.T.);
#1538=FACE_OUTER_BOUND('',#2294,.T.);
#2207=EDGE_LOOP('',(#9143,#9144,#9145,#9146));
#2208=EDGE_LOOP('',(#9147,#9148,#9149,#9150));
#2209=EDGE_LOOP('',(#9151));
#2210=EDGE_LOOP('',(#9152));
#2211=EDGE_LOOP('',(#9153,#9154,#9155,#9156));
#2212=EDGE_LOOP('',(#9157,#9158,#9159,#9160));
#2213=EDGE_LOOP('',(#9161,#9162,#9163,#9164));
#2214=EDGE_LOOP('',(#9165,#9166,#9167,#9168));
#2215=EDGE_LOOP('',(#9169,#9170,#9171,#9172));
#2216=EDGE_LOOP('',(#9173,#9174,#9175,#9176));
#2217=EDGE_LOOP('',(#9177,#9178,#9179,#9180));
#2218=EDGE_LOOP('',(#9181,#9182,#9183,#9184));
#2219=EDGE_LOOP('',(#9185,#9186,#9187,#9188));
#2220=EDGE_LOOP('',(#9189,#9190,#9191,#9192));
#2221=EDGE_LOOP('',(#9193,#9194,#9195,#9196));
#2222=EDGE_LOOP('',(#9197,#9198,#9199,#9200));
#2223=EDGE_LOOP('',(#9201,#9202,#9203,#9204));
#2224=EDGE_LOOP('',(#9205,#9206,#9207,#9208));
#2225=EDGE_LOOP('',(#9209,#9210,#9211,#9212));
#2226=EDGE_LOOP('',(#9213,#9214,#9215,#9216));
#2227=EDGE_LOOP('',(#9217,#9218,#9219,#9220));
#2228=EDGE_LOOP('',(#9221,#9222,#9223,#9224));
#2229=EDGE_LOOP('',(#9225,#9226,#9227,#9228));
#2230=EDGE_LOOP('',(#9229,#9230,#9231,#9232));
#2231=EDGE_LOOP('',(#9233,#9234,#9235,#9236));
#2232=EDGE_LOOP('',(#9237,#9238,#9239,#9240));
#2233=EDGE_LOOP('',(#9241,#9242,#9243,#9244));
#2234=EDGE_LOOP('',(#9245,#9246,#9247,#9248));
#2235=EDGE_LOOP('',(#9249,#9250,#9251,#9252));
#2236=EDGE_LOOP('',(#9253,#9254,#9255,#9256));
#2237=EDGE_LOOP('',(#9257,#9258,#9259,#9260));
#2238=EDGE_LOOP('',(#9261,#9262,#9263,#9264));
#2239=EDGE_LOOP('',(#9265,#9266,#9267,#9268));
#2240=EDGE_LOOP('',(#9269,#9270,#9271,#9272));
#2241=EDGE_LOOP('',(#9273,#9274,#9275,#9276));
#2242=EDGE_LOOP('',(#9277,#9278,#9279,#9280));
#2243=EDGE_LOOP('',(#9281,#9282,#9283,#9284));
#2244=EDGE_LOOP('',(#9285,#9286,#9287,#9288));
#2245=EDGE_LOOP('',(#9289,#9290,#9291,#9292));
#2246=EDGE_LOOP('',(#9293,#9294,#9295,#9296));
#2247=EDGE_LOOP('',(#9297,#9298,#9299,#9300));
#2248=EDGE_LOOP('',(#9301,#9302,#9303,#9304));
#2249=EDGE_LOOP('',(#9305,#9306,#9307,#9308));
#2250=EDGE_LOOP('',(#9309,#9310,#9311,#9312));
#2251=EDGE_LOOP('',(#9313,#9314,#9315,#9316));
#2252=EDGE_LOOP('',(#9317,#9318,#9319,#9320));
#2253=EDGE_LOOP('',(#9321,#9322,#9323,#9324));
#2254=EDGE_LOOP('',(#9325,#9326,#9327,#9328));
#2255=EDGE_LOOP('',(#9329,#9330,#9331,#9332));
#2256=EDGE_LOOP('',(#9333,#9334,#9335,#9336));
#2257=EDGE_LOOP('',(#9337,#9338,#9339,#9340));
#2258=EDGE_LOOP('',(#9341,#9342,#9343,#9344));
#2259=EDGE_LOOP('',(#9345,#9346,#9347,#9348));
#2260=EDGE_LOOP('',(#9349,#9350,#9351,#9352));
#2261=EDGE_LOOP('',(#9353,#9354,#9355,#9356));
#2262=EDGE_LOOP('',(#9357,#9358,#9359,#9360));
#2263=EDGE_LOOP('',(#9361,#9362,#9363,#9364));
#2264=EDGE_LOOP('',(#9365,#9366,#9367,#9368));
#2265=EDGE_LOOP('',(#9369,#9370,#9371,#9372));
#2266=EDGE_LOOP('',(#9373,#9374,#9375,#9376));
#2267=EDGE_LOOP('',(#9377,#9378,#9379,#9380));
#2268=EDGE_LOOP('',(#9381,#9382,#9383,#9384));
#2269=EDGE_LOOP('',(#9385,#9386,#9387,#9388));
#2270=EDGE_LOOP('',(#9389,#9390,#9391,#9392));
#2271=EDGE_LOOP('',(#9393,#9394,#9395,#9396));
#2272=EDGE_LOOP('',(#9397,#9398,#9399,#9400));
#2273=EDGE_LOOP('',(#9401,#9402,#9403,#9404));
#2274=EDGE_LOOP('',(#9405,#9406,#9407,#9408,#9409,#9410,#9411,#9412,#9413,
#9414,#9415,#9416,#9417,#9418,#9419,#9420,#9421,#9422,#9423,#9424,#9425,
#9426,#9427,#9428,#9429,#9430,#9431,#9432,#9433,#9434,#9435,#9436,#9437,
#9438,#9439,#9440,#9441,#9442,#9443,#9444,#9445,#9446,#9447,#9448,#9449,
#9450,#9451,#9452,#9453,#9454,#9455,#9456,#9457,#9458,#9459,#9460,#9461,
#9462,#9463,#9464,#9465,#9466,#9467,#9468,#9469,#9470,#9471,#9472,#9473,
#9474,#9475,#9476,#9477,#9478,#9479,#9480,#9481,#9482,#9483,#9484));
#2275=EDGE_LOOP('',(#9485));
#2276=EDGE_LOOP('',(#9486,#9487,#9488,#9489,#9490,#9491,#9492,#9493,#9494,
#9495,#9496,#9497,#9498,#9499,#9500,#9501,#9502,#9503,#9504,#9505,#9506,
#9507,#9508,#9509,#9510,#9511,#9512,#9513,#9514,#9515,#9516,#9517,#9518,
#9519,#9520,#9521,#9522,#9523,#9524,#9525,#9526,#9527,#9528,#9529,#9530,
#9531,#9532,#9533,#9534,#9535,#9536,#9537,#9538,#9539,#9540,#9541,#9542,
#9543,#9544,#9545,#9546,#9547,#9548,#9549,#9550,#9551,#9552,#9553,#9554,
#9555,#9556,#9557,#9558,#9559,#9560,#9561,#9562,#9563,#9564,#9565));
#2277=EDGE_LOOP('',(#9566));
#2278=EDGE_LOOP('',(#9567,#9568,#9569,#9570));
#2279=EDGE_LOOP('',(#9571,#9572,#9573,#9574));
#2280=EDGE_LOOP('',(#9575,#9576,#9577,#9578));
#2281=EDGE_LOOP('',(#9579,#9580,#9581,#9582));
#2282=EDGE_LOOP('',(#9583,#9584,#9585,#9586));
#2283=EDGE_LOOP('',(#9587,#9588,#9589,#9590));
#2284=EDGE_LOOP('',(#9591,#9592,#9593,#9594));
#2285=EDGE_LOOP('',(#9595,#9596,#9597,#9598));
#2286=EDGE_LOOP('',(#9599,#9600,#9601,#9602));
#2287=EDGE_LOOP('',(#9603,#9604,#9605,#9606));
#2288=EDGE_LOOP('',(#9607,#9608,#9609,#9610));
#2289=EDGE_LOOP('',(#9611,#9612,#9613,#9614));
#2290=EDGE_LOOP('',(#9615,#9616,#9617,#9618));
#2291=EDGE_LOOP('',(#9619,#9620,#9621,#9622));
#2292=EDGE_LOOP('',(#9623,#9624,#9625,#9626));
#2293=EDGE_LOOP('',(#9627,#9628,#9629,#9630));
#2294=EDGE_LOOP('',(#9631,#9632,#9633,#9634));
#3245=LINE('',#31622,#3693);
#3246=LINE('',#31628,#3694);
#3247=LINE('',#31637,#3695);
#3248=LINE('',#31640,#3696);
#3249=LINE('',#31643,#3697);
#3250=LINE('',#31645,#3698);
#3251=LINE('',#31646,#3699);
#3252=LINE('',#31652,#3700);
#3253=LINE('',#31655,#3701);
#3254=LINE('',#31658,#3702);
#3255=LINE('',#31660,#3703);
#3256=LINE('',#31661,#3704);
#3257=LINE('',#31667,#3705);
#3258=LINE('',#31670,#3706);
#3259=LINE('',#31673,#3707);
#3260=LINE('',#31675,#3708);
#3261=LINE('',#31676,#3709);
#3262=LINE('',#31682,#3710);
#3263=LINE('',#31685,#3711);
#3264=LINE('',#31688,#3712);
#3265=LINE('',#31690,#3713);
#3266=LINE('',#31691,#3714);
#3267=LINE('',#31697,#3715);
#3268=LINE('',#31700,#3716);
#3269=LINE('',#31703,#3717);
#3270=LINE('',#31705,#3718);
#3271=LINE('',#31706,#3719);
#3272=LINE('',#31712,#3720);
#3273=LINE('',#31715,#3721);
#3274=LINE('',#31718,#3722);
#3275=LINE('',#31720,#3723);
#3276=LINE('',#31721,#3724);
#3277=LINE('',#31727,#3725);
#3278=LINE('',#31730,#3726);
#3279=LINE('',#31733,#3727);
#3280=LINE('',#31735,#3728);
#3281=LINE('',#31736,#3729);
#3282=LINE('',#31742,#3730);
#3283=LINE('',#31745,#3731);
#3284=LINE('',#31748,#3732);
#3285=LINE('',#31750,#3733);
#3286=LINE('',#31751,#3734);
#3287=LINE('',#31757,#3735);
#3288=LINE('',#31760,#3736);
#3289=LINE('',#31763,#3737);
#3290=LINE('',#31765,#3738);
#3291=LINE('',#31766,#3739);
#3292=LINE('',#31772,#3740);
#3293=LINE('',#31775,#3741);
#3294=LINE('',#31778,#3742);
#3295=LINE('',#31780,#3743);
#3296=LINE('',#31781,#3744);
#3297=LINE('',#31787,#3745);
#3298=LINE('',#31790,#3746);
#3299=LINE('',#31793,#3747);
#3300=LINE('',#31795,#3748);
#3301=LINE('',#31796,#3749);
#3302=LINE('',#31802,#3750);
#3303=LINE('',#31805,#3751);
#3304=LINE('',#31808,#3752);
#3305=LINE('',#31810,#3753);
#3306=LINE('',#31811,#3754);
#3307=LINE('',#31817,#3755);
#3308=LINE('',#31820,#3756);
#3309=LINE('',#31823,#3757);
#3310=LINE('',#31825,#3758);
#3311=LINE('',#31826,#3759);
#3312=LINE('',#31832,#3760);
#3313=LINE('',#31835,#3761);
#3314=LINE('',#31838,#3762);
#3315=LINE('',#31840,#3763);
#3316=LINE('',#31841,#3764);
#3317=LINE('',#31847,#3765);
#3318=LINE('',#31850,#3766);
#3319=LINE('',#31853,#3767);
#3320=LINE('',#31855,#3768);
#3321=LINE('',#31856,#3769);
#3322=LINE('',#31862,#3770);
#3323=LINE('',#31865,#3771);
#3324=LINE('',#31868,#3772);
#3325=LINE('',#31870,#3773);
#3326=LINE('',#31871,#3774);
#3327=LINE('',#31877,#3775);
#3328=LINE('',#31880,#3776);
#3329=LINE('',#31883,#3777);
#3330=LINE('',#31885,#3778);
#3331=LINE('',#31886,#3779);
#3332=LINE('',#31892,#3780);
#3333=LINE('',#31895,#3781);
#3334=LINE('',#31898,#3782);
#3335=LINE('',#31900,#3783);
#3336=LINE('',#31901,#3784);
#3337=LINE('',#32203,#3785);
#3338=LINE('',#32209,#3786);
#3339=LINE('',#32809,#3787);
#3340=LINE('',#32815,#3788);
#3341=LINE('',#33415,#3789);
#3342=LINE('',#33421,#3790);
#3343=LINE('',#34021,#3791);
#3344=LINE('',#34027,#3792);
#3345=LINE('',#34627,#3793);
#3346=LINE('',#34633,#3794);
#3347=LINE('',#35233,#3795);
#3348=LINE('',#35239,#3796);
#3349=LINE('',#35839,#3797);
#3350=LINE('',#35845,#3798);
#3351=LINE('',#36445,#3799);
#3352=LINE('',#36451,#3800);
#3353=LINE('',#37051,#3801);
#3354=LINE('',#37057,#3802);
#3355=LINE('',#37369,#3803);
#3356=LINE('',#37523,#3804);
#3357=LINE('',#37534,#3805);
#3358=LINE('',#37689,#3806);
#3359=LINE('',#37702,#3807);
#3360=LINE('',#37712,#3808);
#3361=LINE('',#37714,#3809);
#3362=LINE('',#37716,#3810);
#3363=LINE('',#37717,#3811);
#3364=LINE('',#37719,#3812);
#3365=LINE('',#37870,#3813);
#3366=LINE('',#37872,#3814);
#3693=VECTOR('',#15745,7.50000000000001);
#3694=VECTOR('',#15752,7.50000000000001);
#3695=VECTOR('',#15763,10.);
#3696=VECTOR('',#15766,10.);
#3697=VECTOR('',#15769,10.);
#3698=VECTOR('',#15770,10.);
#3699=VECTOR('',#15771,10.);
#3700=VECTOR('',#15776,10.);
#3701=VECTOR('',#15779,10.);
#3702=VECTOR('',#15782,10.);
#3703=VECTOR('',#15783,10.);
#3704=VECTOR('',#15784,10.);
#3705=VECTOR('',#15789,10.);
#3706=VECTOR('',#15792,10.);
#3707=VECTOR('',#15795,10.);
#3708=VECTOR('',#15796,10.);
#3709=VECTOR('',#15797,10.);
#3710=VECTOR('',#15802,10.);
#3711=VECTOR('',#15805,10.);
#3712=VECTOR('',#15808,10.);
#3713=VECTOR('',#15809,10.);
#3714=VECTOR('',#15810,10.);
#3715=VECTOR('',#15815,10.);
#3716=VECTOR('',#15818,10.);
#3717=VECTOR('',#15821,10.);
#3718=VECTOR('',#15822,10.);
#3719=VECTOR('',#15823,10.);
#3720=VECTOR('',#15828,10.);
#3721=VECTOR('',#15831,10.);
#3722=VECTOR('',#15834,10.);
#3723=VECTOR('',#15835,10.);
#3724=VECTOR('',#15836,10.);
#3725=VECTOR('',#15841,10.);
#3726=VECTOR('',#15844,10.);
#3727=VECTOR('',#15847,10.);
#3728=VECTOR('',#15848,10.);
#3729=VECTOR('',#15849,10.);
#3730=VECTOR('',#15854,10.);
#3731=VECTOR('',#15857,10.);
#3732=VECTOR('',#15860,10.);
#3733=VECTOR('',#15861,10.);
#3734=VECTOR('',#15862,10.);
#3735=VECTOR('',#15867,10.);
#3736=VECTOR('',#15870,10.);
#3737=VECTOR('',#15873,10.);
#3738=VECTOR('',#15874,10.);
#3739=VECTOR('',#15875,10.);
#3740=VECTOR('',#15880,10.);
#3741=VECTOR('',#15883,10.);
#3742=VECTOR('',#15886,10.);
#3743=VECTOR('',#15887,10.);
#3744=VECTOR('',#15888,10.);
#3745=VECTOR('',#15893,10.);
#3746=VECTOR('',#15896,10.);
#3747=VECTOR('',#15899,10.);
#3748=VECTOR('',#15900,10.);
#3749=VECTOR('',#15901,10.);
#3750=VECTOR('',#15906,10.);
#3751=VECTOR('',#15909,10.);
#3752=VECTOR('',#15912,10.);
#3753=VECTOR('',#15913,10.);
#3754=VECTOR('',#15914,10.);
#3755=VECTOR('',#15919,10.);
#3756=VECTOR('',#15922,10.);
#3757=VECTOR('',#15925,10.);
#3758=VECTOR('',#15926,10.);
#3759=VECTOR('',#15927,10.);
#3760=VECTOR('',#15932,10.);
#3761=VECTOR('',#15935,10.);
#3762=VECTOR('',#15938,10.);
#3763=VECTOR('',#15939,10.);
#3764=VECTOR('',#15940,10.);
#3765=VECTOR('',#15945,10.);
#3766=VECTOR('',#15948,10.);
#3767=VECTOR('',#15951,10.);
#3768=VECTOR('',#15952,10.);
#3769=VECTOR('',#15953,10.);
#3770=VECTOR('',#15958,10.);
#3771=VECTOR('',#15961,10.);
#3772=VECTOR('',#15964,10.);
#3773=VECTOR('',#15965,10.);
#3774=VECTOR('',#15966,10.);
#3775=VECTOR('',#15971,10.);
#3776=VECTOR('',#15974,10.);
#3777=VECTOR('',#15977,10.);
#3778=VECTOR('',#15978,10.);
#3779=VECTOR('',#15979,10.);
#3780=VECTOR('',#15984,10.);
#3781=VECTOR('',#15987,10.);
#3782=VECTOR('',#15990,10.);
#3783=VECTOR('',#15991,10.);
#3784=VECTOR('',#15992,10.);
#3785=VECTOR('',#15993,10.);
#3786=VECTOR('',#16000,10.);
#3787=VECTOR('',#16001,10.);
#3788=VECTOR('',#16008,10.);
#3789=VECTOR('',#16009,10.);
#3790=VECTOR('',#16016,10.);
#3791=VECTOR('',#16017,10.);
#3792=VECTOR('',#16024,10.);
#3793=VECTOR('',#16025,10.);
#3794=VECTOR('',#16032,10.);
#3795=VECTOR('',#16033,10.);
#3796=VECTOR('',#16040,10.);
#3797=VECTOR('',#16041,10.);
#3798=VECTOR('',#16048,10.);
#3799=VECTOR('',#16049,10.);
#3800=VECTOR('',#16056,10.);
#3801=VECTOR('',#16057,10.);
#3802=VECTOR('',#16064,10.);
#3803=VECTOR('',#16085,10.);
#3804=VECTOR('',#16088,10.);
#3805=VECTOR('',#16101,10.);
#3806=VECTOR('',#16104,10.);
#3807=VECTOR('',#16127,10.);
#3808=VECTOR('',#16146,10.);
#3809=VECTOR('',#16149,10.);
#3810=VECTOR('',#16152,10.);
#3811=VECTOR('',#16153,10.);
#3812=VECTOR('',#16156,10.);
#3813=VECTOR('',#16157,10.);
#3814=VECTOR('',#16160,10.);
#4063=CIRCLE('',#13478,7.5);
#4064=CIRCLE('',#13479,7.50000000000001);
#4065=CIRCLE('',#13481,7.50000000000001);
#4066=CIRCLE('',#13482,7.5);
#4067=CIRCLE('',#13486,1.);
#4068=CIRCLE('',#13487,1.);
#4069=CIRCLE('',#13490,1.);
#4070=CIRCLE('',#13491,1.);
#4071=CIRCLE('',#13494,1.);
#4072=CIRCLE('',#13495,1.);
#4073=CIRCLE('',#13498,1.);
#4074=CIRCLE('',#13499,1.);
#4075=CIRCLE('',#13502,1.);
#4076=CIRCLE('',#13503,1.);
#4077=CIRCLE('',#13506,1.);
#4078=CIRCLE('',#13507,1.);
#4079=CIRCLE('',#13510,1.);
#4080=CIRCLE('',#13511,1.);
#4081=CIRCLE('',#13514,1.);
#4082=CIRCLE('',#13515,1.);
#4083=CIRCLE('',#13518,1.);
#4084=CIRCLE('',#13519,1.);
#4085=CIRCLE('',#13522,1.);
#4086=CIRCLE('',#13523,1.);
#4087=CIRCLE('',#13526,1.);
#4088=CIRCLE('',#13527,1.);
#4089=CIRCLE('',#13530,1.);
#4090=CIRCLE('',#13531,1.);
#4091=CIRCLE('',#13534,1.);
#4092=CIRCLE('',#13535,1.);
#4093=CIRCLE('',#13538,1.);
#4094=CIRCLE('',#13539,1.);
#4095=CIRCLE('',#13542,1.);
#4096=CIRCLE('',#13543,1.);
#4097=CIRCLE('',#13546,1.);
#4098=CIRCLE('',#13547,1.);
#4099=CIRCLE('',#13550,1.);
#4100=CIRCLE('',#13551,1.);
#4101=CIRCLE('',#13554,1.);
#4102=CIRCLE('',#13555,1.);
#4103=CIRCLE('',#13558,23.9999999999999);
#4104=CIRCLE('',#13559,23.9999999999999);
#4105=CIRCLE('',#13561,23.9999999999999);
#4106=CIRCLE('',#13562,23.9999999999999);
#4107=CIRCLE('',#13564,23.9999999999999);
#4108=CIRCLE('',#13565,23.9999999999999);
#4109=CIRCLE('',#13567,23.9999999999999);
#4110=CIRCLE('',#13568,23.9999999999999);
#4111=CIRCLE('',#13570,23.9999999999999);
#4112=CIRCLE('',#13571,23.9999999999999);
#4113=CIRCLE('',#13573,23.9999999999999);
#4114=CIRCLE('',#13574,23.9999999999999);
#4115=CIRCLE('',#13576,23.9999999999999);
#4116=CIRCLE('',#13577,23.9999999999999);
#4117=CIRCLE('',#13579,23.9999999999999);
#4118=CIRCLE('',#13580,23.9999999999999);
#4119=CIRCLE('',#13582,23.9999999999999);
#4120=CIRCLE('',#13583,23.9999999999999);
#4121=CIRCLE('',#13585,15.372);
#4122=CIRCLE('',#13586,15.372);
#4123=CIRCLE('',#13587,15.372);
#4124=CIRCLE('',#13588,15.372);
#4125=CIRCLE('',#13589,15.372);
#4126=CIRCLE('',#13590,15.372);
#4127=CIRCLE('',#13591,15.372);
#4128=CIRCLE('',#13592,15.372);
#4129=CIRCLE('',#13593,1.);
#4130=CIRCLE('',#13594,23.9999999999999);
#4131=CIRCLE('',#13595,1.);
#4132=CIRCLE('',#13596,15.372);
#4133=CIRCLE('',#13597,15.372);
#4134=CIRCLE('',#13599,15.372);
#4135=CIRCLE('',#13600,1.);
#4136=CIRCLE('',#13601,23.9999999999999);
#4137=CIRCLE('',#13602,1.);
#4138=CIRCLE('',#13603,15.372);
#4139=CIRCLE('',#13604,15.372);
#4140=CIRCLE('',#13605,15.372);
#4141=CIRCLE('',#13606,15.372);
#4142=CIRCLE('',#13607,15.372);
#4143=CIRCLE('',#13608,15.372);
#4144=CIRCLE('',#13609,15.372);
#4145=CIRCLE('',#13610,15.372);
#4146=CIRCLE('',#13611,15.372);
#5243=VERTEX_POINT('',#31619);
#5244=VERTEX_POINT('',#31621);
#5245=VERTEX_POINT('',#31625);
#5246=VERTEX_POINT('',#31627);
#5247=VERTEX_POINT('',#31633);
#5248=VERTEX_POINT('',#31634);
#5249=VERTEX_POINT('',#31636);
#5250=VERTEX_POINT('',#31638);
#5251=VERTEX_POINT('',#31642);
#5252=VERTEX_POINT('',#31644);
#5253=VERTEX_POINT('',#31648);
#5254=VERTEX_POINT('',#31649);
#5255=VERTEX_POINT('',#31651);
#5256=VERTEX_POINT('',#31653);
#5257=VERTEX_POINT('',#31657);
#5258=VERTEX_POINT('',#31659);
#5259=VERTEX_POINT('',#31663);
#5260=VERTEX_POINT('',#31664);
#5261=VERTEX_POINT('',#31666);
#5262=VERTEX_POINT('',#31668);
#5263=VERTEX_POINT('',#31672);
#5264=VERTEX_POINT('',#31674);
#5265=VERTEX_POINT('',#31678);
#5266=VERTEX_POINT('',#31679);
#5267=VERTEX_POINT('',#31681);
#5268=VERTEX_POINT('',#31683);
#5269=VERTEX_POINT('',#31687);
#5270=VERTEX_POINT('',#31689);
#5271=VERTEX_POINT('',#31693);
#5272=VERTEX_POINT('',#31694);
#5273=VERTEX_POINT('',#31696);
#5274=VERTEX_POINT('',#31698);
#5275=VERTEX_POINT('',#31702);
#5276=VERTEX_POINT('',#31704);
#5277=VERTEX_POINT('',#31708);
#5278=VERTEX_POINT('',#31709);
#5279=VERTEX_POINT('',#31711);
#5280=VERTEX_POINT('',#31713);
#5281=VERTEX_POINT('',#31717);
#5282=VERTEX_POINT('',#31719);
#5283=VERTEX_POINT('',#31723);
#5284=VERTEX_POINT('',#31724);
#5285=VERTEX_POINT('',#31726);
#5286=VERTEX_POINT('',#31728);
#5287=VERTEX_POINT('',#31732);
#5288=VERTEX_POINT('',#31734);
#5289=VERTEX_POINT('',#31738);
#5290=VERTEX_POINT('',#31739);
#5291=VERTEX_POINT('',#31741);
#5292=VERTEX_POINT('',#31743);
#5293=VERTEX_POINT('',#31747);
#5294=VERTEX_POINT('',#31749);
#5295=VERTEX_POINT('',#31753);
#5296=VERTEX_POINT('',#31754);
#5297=VERTEX_POINT('',#31756);
#5298=VERTEX_POINT('',#31758);
#5299=VERTEX_POINT('',#31762);
#5300=VERTEX_POINT('',#31764);
#5301=VERTEX_POINT('',#31768);
#5302=VERTEX_POINT('',#31769);
#5303=VERTEX_POINT('',#31771);
#5304=VERTEX_POINT('',#31773);
#5305=VERTEX_POINT('',#31777);
#5306=VERTEX_POINT('',#31779);
#5307=VERTEX_POINT('',#31783);
#5308=VERTEX_POINT('',#31784);
#5309=VERTEX_POINT('',#31786);
#5310=VERTEX_POINT('',#31788);
#5311=VERTEX_POINT('',#31792);
#5312=VERTEX_POINT('',#31794);
#5313=VERTEX_POINT('',#31798);
#5314=VERTEX_POINT('',#31799);
#5315=VERTEX_POINT('',#31801);
#5316=VERTEX_POINT('',#31803);
#5317=VERTEX_POINT('',#31807);
#5318=VERTEX_POINT('',#31809);
#5319=VERTEX_POINT('',#31813);
#5320=VERTEX_POINT('',#31814);
#5321=VERTEX_POINT('',#31816);
#5322=VERTEX_POINT('',#31818);
#5323=VERTEX_POINT('',#31822);
#5324=VERTEX_POINT('',#31824);
#5325=VERTEX_POINT('',#31828);
#5326=VERTEX_POINT('',#31829);
#5327=VERTEX_POINT('',#31831);
#5328=VERTEX_POINT('',#31833);
#5329=VERTEX_POINT('',#31837);
#5330=VERTEX_POINT('',#31839);
#5331=VERTEX_POINT('',#31843);
#5332=VERTEX_POINT('',#31844);
#5333=VERTEX_POINT('',#31846);
#5334=VERTEX_POINT('',#31848);
#5335=VERTEX_POINT('',#31852);
#5336=VERTEX_POINT('',#31854);
#5337=VERTEX_POINT('',#31858);
#5338=VERTEX_POINT('',#31859);
#5339=VERTEX_POINT('',#31861);
#5340=VERTEX_POINT('',#31863);
#5341=VERTEX_POINT('',#31867);
#5342=VERTEX_POINT('',#31869);
#5343=VERTEX_POINT('',#31873);
#5344=VERTEX_POINT('',#31874);
#5345=VERTEX_POINT('',#31876);
#5346=VERTEX_POINT('',#31878);
#5347=VERTEX_POINT('',#31882);
#5348=VERTEX_POINT('',#31884);
#5349=VERTEX_POINT('',#31888);
#5350=VERTEX_POINT('',#31889);
#5351=VERTEX_POINT('',#31891);
#5352=VERTEX_POINT('',#31893);
#5353=VERTEX_POINT('',#31897);
#5354=VERTEX_POINT('',#31899);
#5355=VERTEX_POINT('',#32052);
#5356=VERTEX_POINT('',#32127);
#5357=VERTEX_POINT('',#32205);
#5358=VERTEX_POINT('',#32207);
#5359=VERTEX_POINT('',#32658);
#5360=VERTEX_POINT('',#32733);
#5361=VERTEX_POINT('',#32811);
#5362=VERTEX_POINT('',#32813);
#5363=VERTEX_POINT('',#33264);
#5364=VERTEX_POINT('',#33339);
#5365=VERTEX_POINT('',#33417);
#5366=VERTEX_POINT('',#33419);
#5367=VERTEX_POINT('',#33870);
#5368=VERTEX_POINT('',#33945);
#5369=VERTEX_POINT('',#34023);
#5370=VERTEX_POINT('',#34025);
#5371=VERTEX_POINT('',#34476);
#5372=VERTEX_POINT('',#34551);
#5373=VERTEX_POINT('',#34629);
#5374=VERTEX_POINT('',#34631);
#5375=VERTEX_POINT('',#35082);
#5376=VERTEX_POINT('',#35157);
#5377=VERTEX_POINT('',#35235);
#5378=VERTEX_POINT('',#35237);
#5379=VERTEX_POINT('',#35688);
#5380=VERTEX_POINT('',#35763);
#5381=VERTEX_POINT('',#35841);
#5382=VERTEX_POINT('',#35843);
#5383=VERTEX_POINT('',#36294);
#5384=VERTEX_POINT('',#36369);
#5385=VERTEX_POINT('',#36447);
#5386=VERTEX_POINT('',#36449);
#5387=VERTEX_POINT('',#36900);
#5388=VERTEX_POINT('',#36975);
#5389=VERTEX_POINT('',#37053);
#5390=VERTEX_POINT('',#37055);
#5391=VERTEX_POINT('',#37364);
#5392=VERTEX_POINT('',#37366);
#5393=VERTEX_POINT('',#37368);
#5394=VERTEX_POINT('',#37370);
#5395=VERTEX_POINT('',#37445);
#5396=VERTEX_POINT('',#37447);
#5397=VERTEX_POINT('',#37522);
#5398=VERTEX_POINT('',#37524);
#5399=VERTEX_POINT('',#37529);
#5400=VERTEX_POINT('',#37531);
#5401=VERTEX_POINT('',#37533);
#5402=VERTEX_POINT('',#37535);
#5403=VERTEX_POINT('',#37610);
#5404=VERTEX_POINT('',#37612);
#5405=VERTEX_POINT('',#37688);
#5406=VERTEX_POINT('',#37690);
#6733=EDGE_CURVE('',#5243,#5243,#4063,.T.);
#6734=EDGE_CURVE('',#5243,#5244,#3245,.T.);
#6735=EDGE_CURVE('',#5244,#5244,#4064,.F.);
#6736=EDGE_CURVE('',#5245,#5245,#4065,.T.);
#6737=EDGE_CURVE('',#5245,#5246,#3246,.T.);
#6738=EDGE_CURVE('',#5246,#5246,#4066,.T.);
#6739=EDGE_CURVE('',#5247,#5248,#4067,.T.);
#6740=EDGE_CURVE('',#5248,#5249,#3247,.T.);
#6741=EDGE_CURVE('',#5249,#5250,#4068,.T.);
#6742=EDGE_CURVE('',#5250,#5247,#3248,.T.);
#6743=EDGE_CURVE('',#5251,#5248,#3249,.T.);
#6744=EDGE_CURVE('',#5252,#5251,#3250,.T.);
#6745=EDGE_CURVE('',#5249,#5252,#3251,.T.);
#6746=EDGE_CURVE('',#5253,#5254,#4069,.T.);
#6747=EDGE_CURVE('',#5254,#5255,#3252,.T.);
#6748=EDGE_CURVE('',#5255,#5256,#4070,.T.);
#6749=EDGE_CURVE('',#5256,#5253,#3253,.T.);
#6750=EDGE_CURVE('',#5254,#5257,#3254,.T.);
#6751=EDGE_CURVE('',#5257,#5258,#3255,.T.);
#6752=EDGE_CURVE('',#5255,#5258,#3256,.T.);
#6753=EDGE_CURVE('',#5259,#5260,#4071,.T.);
#6754=EDGE_CURVE('',#5260,#5261,#3257,.T.);
#6755=EDGE_CURVE('',#5261,#5262,#4072,.T.);
#6756=EDGE_CURVE('',#5262,#5259,#3258,.T.);
#6757=EDGE_CURVE('',#5263,#5260,#3259,.T.);
#6758=EDGE_CURVE('',#5264,#5263,#3260,.T.);
#6759=EDGE_CURVE('',#5261,#5264,#3261,.T.);
#6760=EDGE_CURVE('',#5265,#5266,#4073,.T.);
#6761=EDGE_CURVE('',#5266,#5267,#3262,.T.);
#6762=EDGE_CURVE('',#5267,#5268,#4074,.T.);
#6763=EDGE_CURVE('',#5268,#5265,#3263,.T.);
#6764=EDGE_CURVE('',#5266,#5269,#3264,.T.);
#6765=EDGE_CURVE('',#5269,#5270,#3265,.T.);
#6766=EDGE_CURVE('',#5267,#5270,#3266,.T.);
#6767=EDGE_CURVE('',#5271,#5272,#4075,.T.);
#6768=EDGE_CURVE('',#5272,#5273,#3267,.T.);
#6769=EDGE_CURVE('',#5273,#5274,#4076,.T.);
#6770=EDGE_CURVE('',#5274,#5271,#3268,.T.);
#6771=EDGE_CURVE('',#5275,#5272,#3269,.T.);
#6772=EDGE_CURVE('',#5276,#5275,#3270,.T.);
#6773=EDGE_CURVE('',#5273,#5276,#3271,.T.);
#6774=EDGE_CURVE('',#5277,#5278,#4077,.T.);
#6775=EDGE_CURVE('',#5278,#5279,#3272,.T.);
#6776=EDGE_CURVE('',#5279,#5280,#4078,.T.);
#6777=EDGE_CURVE('',#5280,#5277,#3273,.T.);
#6778=EDGE_CURVE('',#5278,#5281,#3274,.T.);
#6779=EDGE_CURVE('',#5281,#5282,#3275,.T.);
#6780=EDGE_CURVE('',#5279,#5282,#3276,.T.);
#6781=EDGE_CURVE('',#5283,#5284,#4079,.T.);
#6782=EDGE_CURVE('',#5284,#5285,#3277,.T.);
#6783=EDGE_CURVE('',#5285,#5286,#4080,.T.);
#6784=EDGE_CURVE('',#5286,#5283,#3278,.T.);
#6785=EDGE_CURVE('',#5287,#5284,#3279,.T.);
#6786=EDGE_CURVE('',#5288,#5287,#3280,.T.);
#6787=EDGE_CURVE('',#5285,#5288,#3281,.T.);
#6788=EDGE_CURVE('',#5289,#5290,#4081,.T.);
#6789=EDGE_CURVE('',#5290,#5291,#3282,.T.);
#6790=EDGE_CURVE('',#5291,#5292,#4082,.T.);
#6791=EDGE_CURVE('',#5292,#5289,#3283,.T.);
#6792=EDGE_CURVE('',#5290,#5293,#3284,.T.);
#6793=EDGE_CURVE('',#5293,#5294,#3285,.T.);
#6794=EDGE_CURVE('',#5291,#5294,#3286,.T.);
#6795=EDGE_CURVE('',#5295,#5296,#4083,.T.);
#6796=EDGE_CURVE('',#5296,#5297,#3287,.T.);
#6797=EDGE_CURVE('',#5297,#5298,#4084,.T.);
#6798=EDGE_CURVE('',#5298,#5295,#3288,.T.);
#6799=EDGE_CURVE('',#5299,#5296,#3289,.T.);
#6800=EDGE_CURVE('',#5300,#5299,#3290,.T.);
#6801=EDGE_CURVE('',#5297,#5300,#3291,.T.);
#6802=EDGE_CURVE('',#5301,#5302,#4085,.T.);
#6803=EDGE_CURVE('',#5302,#5303,#3292,.T.);
#6804=EDGE_CURVE('',#5303,#5304,#4086,.T.);
#6805=EDGE_CURVE('',#5304,#5301,#3293,.T.);
#6806=EDGE_CURVE('',#5302,#5305,#3294,.T.);
#6807=EDGE_CURVE('',#5305,#5306,#3295,.T.);
#6808=EDGE_CURVE('',#5303,#5306,#3296,.T.);
#6809=EDGE_CURVE('',#5307,#5308,#4087,.T.);
#6810=EDGE_CURVE('',#5308,#5309,#3297,.T.);
#6811=EDGE_CURVE('',#5309,#5310,#4088,.T.);
#6812=EDGE_CURVE('',#5310,#5307,#3298,.T.);
#6813=EDGE_CURVE('',#5311,#5308,#3299,.T.);
#6814=EDGE_CURVE('',#5312,#5311,#3300,.T.);
#6815=EDGE_CURVE('',#5309,#5312,#3301,.T.);
#6816=EDGE_CURVE('',#5313,#5314,#4089,.T.);
#6817=EDGE_CURVE('',#5314,#5315,#3302,.T.);
#6818=EDGE_CURVE('',#5315,#5316,#4090,.T.);
#6819=EDGE_CURVE('',#5316,#5313,#3303,.T.);
#6820=EDGE_CURVE('',#5314,#5317,#3304,.T.);
#6821=EDGE_CURVE('',#5317,#5318,#3305,.T.);
#6822=EDGE_CURVE('',#5315,#5318,#3306,.T.);
#6823=EDGE_CURVE('',#5319,#5320,#4091,.T.);
#6824=EDGE_CURVE('',#5320,#5321,#3307,.T.);
#6825=EDGE_CURVE('',#5321,#5322,#4092,.T.);
#6826=EDGE_CURVE('',#5322,#5319,#3308,.T.);
#6827=EDGE_CURVE('',#5323,#5320,#3309,.T.);
#6828=EDGE_CURVE('',#5324,#5323,#3310,.T.);
#6829=EDGE_CURVE('',#5321,#5324,#3311,.T.);
#6830=EDGE_CURVE('',#5325,#5326,#4093,.T.);
#6831=EDGE_CURVE('',#5326,#5327,#3312,.T.);
#6832=EDGE_CURVE('',#5327,#5328,#4094,.T.);
#6833=EDGE_CURVE('',#5328,#5325,#3313,.T.);
#6834=EDGE_CURVE('',#5326,#5329,#3314,.T.);
#6835=EDGE_CURVE('',#5329,#5330,#3315,.T.);
#6836=EDGE_CURVE('',#5327,#5330,#3316,.T.);
#6837=EDGE_CURVE('',#5331,#5332,#4095,.T.);
#6838=EDGE_CURVE('',#5332,#5333,#3317,.T.);
#6839=EDGE_CURVE('',#5333,#5334,#4096,.T.);
#6840=EDGE_CURVE('',#5334,#5331,#3318,.T.);
#6841=EDGE_CURVE('',#5335,#5332,#3319,.T.);
#6842=EDGE_CURVE('',#5336,#5335,#3320,.T.);
#6843=EDGE_CURVE('',#5333,#5336,#3321,.T.);
#6844=EDGE_CURVE('',#5337,#5338,#4097,.T.);
#6845=EDGE_CURVE('',#5338,#5339,#3322,.T.);
#6846=EDGE_CURVE('',#5339,#5340,#4098,.T.);
#6847=EDGE_CURVE('',#5340,#5337,#3323,.T.);
#6848=EDGE_CURVE('',#5338,#5341,#3324,.T.);
#6849=EDGE_CURVE('',#5341,#5342,#3325,.T.);
#6850=EDGE_CURVE('',#5339,#5342,#3326,.T.);
#6851=EDGE_CURVE('',#5343,#5344,#4099,.T.);
#6852=EDGE_CURVE('',#5344,#5345,#3327,.T.);
#6853=EDGE_CURVE('',#5345,#5346,#4100,.T.);
#6854=EDGE_CURVE('',#5346,#5343,#3328,.T.);
#6855=EDGE_CURVE('',#5347,#5344,#3329,.T.);
#6856=EDGE_CURVE('',#5348,#5347,#3330,.T.);
#6857=EDGE_CURVE('',#5345,#5348,#3331,.T.);
#6858=EDGE_CURVE('',#5349,#5350,#4101,.T.);
#6859=EDGE_CURVE('',#5350,#5351,#3332,.T.);
#6860=EDGE_CURVE('',#5351,#5352,#4102,.T.);
#6861=EDGE_CURVE('',#5352,#5349,#3333,.T.);
#6862=EDGE_CURVE('',#5350,#5353,#3334,.T.);
#6863=EDGE_CURVE('',#5353,#5354,#3335,.T.);
#6864=EDGE_CURVE('',#5351,#5354,#3336,.T.);
#6865=EDGE_CURVE('',#5252,#5355,#571,.T.);
#6866=EDGE_CURVE('',#5356,#5251,#572,.T.);
#6867=EDGE_CURVE('',#5355,#5356,#3337,.T.);
#6868=EDGE_CURVE('',#5357,#5355,#4103,.T.);
#6869=EDGE_CURVE('',#5358,#5356,#4104,.T.);
#6870=EDGE_CURVE('',#5357,#5358,#3338,.T.);
#6871=EDGE_CURVE('',#5257,#5357,#573,.T.);
#6872=EDGE_CURVE('',#5258,#5358,#574,.T.);
#6873=EDGE_CURVE('',#5264,#5359,#575,.T.);
#6874=EDGE_CURVE('',#5360,#5263,#576,.T.);
#6875=EDGE_CURVE('',#5359,#5360,#3339,.T.);
#6876=EDGE_CURVE('',#5361,#5359,#4105,.T.);
#6877=EDGE_CURVE('',#5362,#5360,#4106,.T.);
#6878=EDGE_CURVE('',#5361,#5362,#3340,.T.);
#6879=EDGE_CURVE('',#5269,#5361,#577,.T.);
#6880=EDGE_CURVE('',#5270,#5362,#578,.T.);
#6881=EDGE_CURVE('',#5276,#5363,#579,.T.);
#6882=EDGE_CURVE('',#5364,#5275,#580,.T.);
#6883=EDGE_CURVE('',#5363,#5364,#3341,.T.);
#6884=EDGE_CURVE('',#5365,#5363,#4107,.T.);
#6885=EDGE_CURVE('',#5366,#5364,#4108,.T.);
#6886=EDGE_CURVE('',#5365,#5366,#3342,.T.);
#6887=EDGE_CURVE('',#5281,#5365,#581,.T.);
#6888=EDGE_CURVE('',#5282,#5366,#582,.T.);
#6889=EDGE_CURVE('',#5288,#5367,#583,.T.);
#6890=EDGE_CURVE('',#5368,#5287,#584,.T.);
#6891=EDGE_CURVE('',#5367,#5368,#3343,.T.);
#6892=EDGE_CURVE('',#5369,#5367,#4109,.T.);
#6893=EDGE_CURVE('',#5370,#5368,#4110,.T.);
#6894=EDGE_CURVE('',#5369,#5370,#3344,.T.);
#6895=EDGE_CURVE('',#5293,#5369,#585,.T.);
#6896=EDGE_CURVE('',#5294,#5370,#586,.T.);
#6897=EDGE_CURVE('',#5300,#5371,#587,.T.);
#6898=EDGE_CURVE('',#5372,#5299,#588,.T.);
#6899=EDGE_CURVE('',#5371,#5372,#3345,.T.);
#6900=EDGE_CURVE('',#5373,#5371,#4111,.T.);
#6901=EDGE_CURVE('',#5374,#5372,#4112,.T.);
#6902=EDGE_CURVE('',#5373,#5374,#3346,.T.);
#6903=EDGE_CURVE('',#5305,#5373,#589,.T.);
#6904=EDGE_CURVE('',#5306,#5374,#590,.T.);
#6905=EDGE_CURVE('',#5312,#5375,#591,.T.);
#6906=EDGE_CURVE('',#5376,#5311,#592,.T.);
#6907=EDGE_CURVE('',#5375,#5376,#3347,.T.);
#6908=EDGE_CURVE('',#5377,#5375,#4113,.T.);
#6909=EDGE_CURVE('',#5378,#5376,#4114,.T.);
#6910=EDGE_CURVE('',#5377,#5378,#3348,.T.);
#6911=EDGE_CURVE('',#5317,#5377,#593,.T.);
#6912=EDGE_CURVE('',#5318,#5378,#594,.T.);
#6913=EDGE_CURVE('',#5324,#5379,#595,.T.);
#6914=EDGE_CURVE('',#5380,#5323,#596,.T.);
#6915=EDGE_CURVE('',#5379,#5380,#3349,.T.);
#6916=EDGE_CURVE('',#5381,#5379,#4115,.T.);
#6917=EDGE_CURVE('',#5382,#5380,#4116,.T.);
#6918=EDGE_CURVE('',#5381,#5382,#3350,.T.);
#6919=EDGE_CURVE('',#5329,#5381,#597,.T.);
#6920=EDGE_CURVE('',#5330,#5382,#598,.T.);
#6921=EDGE_CURVE('',#5336,#5383,#599,.T.);
#6922=EDGE_CURVE('',#5384,#5335,#600,.T.);
#6923=EDGE_CURVE('',#5383,#5384,#3351,.T.);
#6924=EDGE_CURVE('',#5385,#5383,#4117,.T.);
#6925=EDGE_CURVE('',#5386,#5384,#4118,.T.);
#6926=EDGE_CURVE('',#5385,#5386,#3352,.T.);
#6927=EDGE_CURVE('',#5341,#5385,#601,.T.);
#6928=EDGE_CURVE('',#5342,#5386,#602,.T.);
#6929=EDGE_CURVE('',#5348,#5387,#603,.T.);
#6930=EDGE_CURVE('',#5388,#5347,#604,.T.);
#6931=EDGE_CURVE('',#5387,#5388,#3353,.T.);
#6932=EDGE_CURVE('',#5389,#5387,#4119,.T.);
#6933=EDGE_CURVE('',#5390,#5388,#4120,.T.);
#6934=EDGE_CURVE('',#5389,#5390,#3354,.T.);
#6935=EDGE_CURVE('',#5353,#5389,#605,.T.);
#6936=EDGE_CURVE('',#5354,#5390,#606,.T.);
#6937=EDGE_CURVE('',#5274,#5265,#4121,.T.);
#6938=EDGE_CURVE('',#5286,#5277,#4122,.T.);
#6939=EDGE_CURVE('',#5298,#5289,#4123,.T.);
#6940=EDGE_CURVE('',#5310,#5301,#4124,.T.);
#6941=EDGE_CURVE('',#5322,#5313,#4125,.T.);
#6942=EDGE_CURVE('',#5334,#5325,#4126,.T.);
#6943=EDGE_CURVE('',#5346,#5337,#4127,.T.);
#6944=EDGE_CURVE('',#5391,#5349,#4128,.T.);
#6945=EDGE_CURVE('',#5392,#5391,#4129,.T.);
#6946=EDGE_CURVE('',#5392,#5393,#3355,.T.);
#6947=EDGE_CURVE('',#5393,#5394,#607,.T.);
#6948=EDGE_CURVE('',#5395,#5394,#4130,.T.);
#6949=EDGE_CURVE('',#5396,#5395,#608,.T.);
#6950=EDGE_CURVE('',#5397,#5396,#3356,.T.);
#6951=EDGE_CURVE('',#5398,#5397,#4131,.T.);
#6952=EDGE_CURVE('',#5250,#5398,#4132,.T.);
#6953=EDGE_CURVE('',#5262,#5253,#4133,.T.);
#6954=EDGE_CURVE('',#5247,#5399,#4134,.T.);
#6955=EDGE_CURVE('',#5400,#5399,#4135,.T.);
#6956=EDGE_CURVE('',#5400,#5401,#3357,.T.);
#6957=EDGE_CURVE('',#5401,#5402,#609,.T.);
#6958=EDGE_CURVE('',#5402,#5403,#4136,.T.);
#6959=EDGE_CURVE('',#5403,#5404,#610,.T.);
#6960=EDGE_CURVE('',#5404,#5405,#3358,.T.);
#6961=EDGE_CURVE('',#5406,#5405,#4137,.T.);
#6962=EDGE_CURVE('',#5406,#5352,#4138,.T.);
#6963=EDGE_CURVE('',#5343,#5340,#4139,.T.);
#6964=EDGE_CURVE('',#5331,#5328,#4140,.T.);
#6965=EDGE_CURVE('',#5319,#5316,#4141,.T.);
#6966=EDGE_CURVE('',#5307,#5304,#4142,.T.);
#6967=EDGE_CURVE('',#5295,#5292,#4143,.T.);
#6968=EDGE_CURVE('',#5283,#5280,#4144,.T.);
#6969=EDGE_CURVE('',#5271,#5268,#4145,.T.);
#6970=EDGE_CURVE('',#5259,#5256,#4146,.T.);
#6971=EDGE_CURVE('',#5391,#5406,#3359,.T.);
#6972=EDGE_CURVE('',#5405,#5392,#3360,.T.);
#6973=EDGE_CURVE('',#5393,#5404,#3361,.T.);
#6974=EDGE_CURVE('',#5397,#5400,#3362,.T.);
#6975=EDGE_CURVE('',#5399,#5398,#3363,.T.);
#6976=EDGE_CURVE('',#5396,#5401,#3364,.T.);
#6977=EDGE_CURVE('',#5394,#5403,#3365,.T.);
#6978=EDGE_CURVE('',#5395,#5402,#3366,.T.);
#9143=ORIENTED_EDGE('',*,*,#6733,.F.);
#9144=ORIENTED_EDGE('',*,*,#6734,.T.);
#9145=ORIENTED_EDGE('',*,*,#6735,.F.);
#9146=ORIENTED_EDGE('',*,*,#6734,.F.);
#9147=ORIENTED_EDGE('',*,*,#6736,.F.);
#9148=ORIENTED_EDGE('',*,*,#6737,.T.);
#9149=ORIENTED_EDGE('',*,*,#6738,.F.);
#9150=ORIENTED_EDGE('',*,*,#6737,.F.);
#9151=ORIENTED_EDGE('',*,*,#6735,.T.);
#9152=ORIENTED_EDGE('',*,*,#6736,.T.);
#9153=ORIENTED_EDGE('',*,*,#6739,.T.);
#9154=ORIENTED_EDGE('',*,*,#6740,.T.);
#9155=ORIENTED_EDGE('',*,*,#6741,.T.);
#9156=ORIENTED_EDGE('',*,*,#6742,.T.);
#9157=ORIENTED_EDGE('',*,*,#6740,.F.);
#9158=ORIENTED_EDGE('',*,*,#6743,.F.);
#9159=ORIENTED_EDGE('',*,*,#6744,.F.);
#9160=ORIENTED_EDGE('',*,*,#6745,.F.);
#9161=ORIENTED_EDGE('',*,*,#6746,.T.);
#9162=ORIENTED_EDGE('',*,*,#6747,.T.);
#9163=ORIENTED_EDGE('',*,*,#6748,.T.);
#9164=ORIENTED_EDGE('',*,*,#6749,.T.);
#9165=ORIENTED_EDGE('',*,*,#6747,.F.);
#9166=ORIENTED_EDGE('',*,*,#6750,.T.);
#9167=ORIENTED_EDGE('',*,*,#6751,.T.);
#9168=ORIENTED_EDGE('',*,*,#6752,.F.);
#9169=ORIENTED_EDGE('',*,*,#6753,.T.);
#9170=ORIENTED_EDGE('',*,*,#6754,.T.);
#9171=ORIENTED_EDGE('',*,*,#6755,.T.);
#9172=ORIENTED_EDGE('',*,*,#6756,.T.);
#9173=ORIENTED_EDGE('',*,*,#6754,.F.);
#9174=ORIENTED_EDGE('',*,*,#6757,.F.);
#9175=ORIENTED_EDGE('',*,*,#6758,.F.);
#9176=ORIENTED_EDGE('',*,*,#6759,.F.);
#9177=ORIENTED_EDGE('',*,*,#6760,.T.);
#9178=ORIENTED_EDGE('',*,*,#6761,.T.);
#9179=ORIENTED_EDGE('',*,*,#6762,.T.);
#9180=ORIENTED_EDGE('',*,*,#6763,.T.);
#9181=ORIENTED_EDGE('',*,*,#6761,.F.);
#9182=ORIENTED_EDGE('',*,*,#6764,.T.);
#9183=ORIENTED_EDGE('',*,*,#6765,.T.);
#9184=ORIENTED_EDGE('',*,*,#6766,.F.);
#9185=ORIENTED_EDGE('',*,*,#6767,.T.);
#9186=ORIENTED_EDGE('',*,*,#6768,.T.);
#9187=ORIENTED_EDGE('',*,*,#6769,.T.);
#9188=ORIENTED_EDGE('',*,*,#6770,.T.);
#9189=ORIENTED_EDGE('',*,*,#6768,.F.);
#9190=ORIENTED_EDGE('',*,*,#6771,.F.);
#9191=ORIENTED_EDGE('',*,*,#6772,.F.);
#9192=ORIENTED_EDGE('',*,*,#6773,.F.);
#9193=ORIENTED_EDGE('',*,*,#6774,.T.);
#9194=ORIENTED_EDGE('',*,*,#6775,.T.);
#9195=ORIENTED_EDGE('',*,*,#6776,.T.);
#9196=ORIENTED_EDGE('',*,*,#6777,.T.);
#9197=ORIENTED_EDGE('',*,*,#6775,.F.);
#9198=ORIENTED_EDGE('',*,*,#6778,.T.);
#9199=ORIENTED_EDGE('',*,*,#6779,.T.);
#9200=ORIENTED_EDGE('',*,*,#6780,.F.);
#9201=ORIENTED_EDGE('',*,*,#6781,.T.);
#9202=ORIENTED_EDGE('',*,*,#6782,.T.);
#9203=ORIENTED_EDGE('',*,*,#6783,.T.);
#9204=ORIENTED_EDGE('',*,*,#6784,.T.);
#9205=ORIENTED_EDGE('',*,*,#6782,.F.);
#9206=ORIENTED_EDGE('',*,*,#6785,.F.);
#9207=ORIENTED_EDGE('',*,*,#6786,.F.);
#9208=ORIENTED_EDGE('',*,*,#6787,.F.);
#9209=ORIENTED_EDGE('',*,*,#6788,.T.);
#9210=ORIENTED_EDGE('',*,*,#6789,.T.);
#9211=ORIENTED_EDGE('',*,*,#6790,.T.);
#9212=ORIENTED_EDGE('',*,*,#6791,.T.);
#9213=ORIENTED_EDGE('',*,*,#6789,.F.);
#9214=ORIENTED_EDGE('',*,*,#6792,.T.);
#9215=ORIENTED_EDGE('',*,*,#6793,.T.);
#9216=ORIENTED_EDGE('',*,*,#6794,.F.);
#9217=ORIENTED_EDGE('',*,*,#6795,.T.);
#9218=ORIENTED_EDGE('',*,*,#6796,.T.);
#9219=ORIENTED_EDGE('',*,*,#6797,.T.);
#9220=ORIENTED_EDGE('',*,*,#6798,.T.);
#9221=ORIENTED_EDGE('',*,*,#6796,.F.);
#9222=ORIENTED_EDGE('',*,*,#6799,.F.);
#9223=ORIENTED_EDGE('',*,*,#6800,.F.);
#9224=ORIENTED_EDGE('',*,*,#6801,.F.);
#9225=ORIENTED_EDGE('',*,*,#6802,.T.);
#9226=ORIENTED_EDGE('',*,*,#6803,.T.);
#9227=ORIENTED_EDGE('',*,*,#6804,.T.);
#9228=ORIENTED_EDGE('',*,*,#6805,.T.);
#9229=ORIENTED_EDGE('',*,*,#6803,.F.);
#9230=ORIENTED_EDGE('',*,*,#6806,.T.);
#9231=ORIENTED_EDGE('',*,*,#6807,.T.);
#9232=ORIENTED_EDGE('',*,*,#6808,.F.);
#9233=ORIENTED_EDGE('',*,*,#6809,.T.);
#9234=ORIENTED_EDGE('',*,*,#6810,.T.);
#9235=ORIENTED_EDGE('',*,*,#6811,.T.);
#9236=ORIENTED_EDGE('',*,*,#6812,.T.);
#9237=ORIENTED_EDGE('',*,*,#6810,.F.);
#9238=ORIENTED_EDGE('',*,*,#6813,.F.);
#9239=ORIENTED_EDGE('',*,*,#6814,.F.);
#9240=ORIENTED_EDGE('',*,*,#6815,.F.);
#9241=ORIENTED_EDGE('',*,*,#6816,.T.);
#9242=ORIENTED_EDGE('',*,*,#6817,.T.);
#9243=ORIENTED_EDGE('',*,*,#6818,.T.);
#9244=ORIENTED_EDGE('',*,*,#6819,.T.);
#9245=ORIENTED_EDGE('',*,*,#6817,.F.);
#9246=ORIENTED_EDGE('',*,*,#6820,.T.);
#9247=ORIENTED_EDGE('',*,*,#6821,.T.);
#9248=ORIENTED_EDGE('',*,*,#6822,.F.);
#9249=ORIENTED_EDGE('',*,*,#6823,.T.);
#9250=ORIENTED_EDGE('',*,*,#6824,.T.);
#9251=ORIENTED_EDGE('',*,*,#6825,.T.);
#9252=ORIENTED_EDGE('',*,*,#6826,.T.);
#9253=ORIENTED_EDGE('',*,*,#6824,.F.);
#9254=ORIENTED_EDGE('',*,*,#6827,.F.);
#9255=ORIENTED_EDGE('',*,*,#6828,.F.);
#9256=ORIENTED_EDGE('',*,*,#6829,.F.);
#9257=ORIENTED_EDGE('',*,*,#6830,.T.);
#9258=ORIENTED_EDGE('',*,*,#6831,.T.);
#9259=ORIENTED_EDGE('',*,*,#6832,.T.);
#9260=ORIENTED_EDGE('',*,*,#6833,.T.);
#9261=ORIENTED_EDGE('',*,*,#6831,.F.);
#9262=ORIENTED_EDGE('',*,*,#6834,.T.);
#9263=ORIENTED_EDGE('',*,*,#6835,.T.);
#9264=ORIENTED_EDGE('',*,*,#6836,.F.);
#9265=ORIENTED_EDGE('',*,*,#6837,.T.);
#9266=ORIENTED_EDGE('',*,*,#6838,.T.);
#9267=ORIENTED_EDGE('',*,*,#6839,.T.);
#9268=ORIENTED_EDGE('',*,*,#6840,.T.);
#9269=ORIENTED_EDGE('',*,*,#6838,.F.);
#9270=ORIENTED_EDGE('',*,*,#6841,.F.);
#9271=ORIENTED_EDGE('',*,*,#6842,.F.);
#9272=ORIENTED_EDGE('',*,*,#6843,.F.);
#9273=ORIENTED_EDGE('',*,*,#6844,.T.);
#9274=ORIENTED_EDGE('',*,*,#6845,.T.);
#9275=ORIENTED_EDGE('',*,*,#6846,.T.);
#9276=ORIENTED_EDGE('',*,*,#6847,.T.);
#9277=ORIENTED_EDGE('',*,*,#6845,.F.);
#9278=ORIENTED_EDGE('',*,*,#6848,.T.);
#9279=ORIENTED_EDGE('',*,*,#6849,.T.);
#9280=ORIENTED_EDGE('',*,*,#6850,.F.);
#9281=ORIENTED_EDGE('',*,*,#6851,.T.);
#9282=ORIENTED_EDGE('',*,*,#6852,.T.);
#9283=ORIENTED_EDGE('',*,*,#6853,.T.);
#9284=ORIENTED_EDGE('',*,*,#6854,.T.);
#9285=ORIENTED_EDGE('',*,*,#6852,.F.);
#9286=ORIENTED_EDGE('',*,*,#6855,.F.);
#9287=ORIENTED_EDGE('',*,*,#6856,.F.);
#9288=ORIENTED_EDGE('',*,*,#6857,.F.);
#9289=ORIENTED_EDGE('',*,*,#6858,.T.);
#9290=ORIENTED_EDGE('',*,*,#6859,.T.);
#9291=ORIENTED_EDGE('',*,*,#6860,.T.);
#9292=ORIENTED_EDGE('',*,*,#6861,.T.);
#9293=ORIENTED_EDGE('',*,*,#6859,.F.);
#9294=ORIENTED_EDGE('',*,*,#6862,.T.);
#9295=ORIENTED_EDGE('',*,*,#6863,.T.);
#9296=ORIENTED_EDGE('',*,*,#6864,.F.);
#9297=ORIENTED_EDGE('',*,*,#6865,.F.);
#9298=ORIENTED_EDGE('',*,*,#6744,.T.);
#9299=ORIENTED_EDGE('',*,*,#6866,.F.);
#9300=ORIENTED_EDGE('',*,*,#6867,.F.);
#9301=ORIENTED_EDGE('',*,*,#6868,.T.);
#9302=ORIENTED_EDGE('',*,*,#6867,.T.);
#9303=ORIENTED_EDGE('',*,*,#6869,.F.);
#9304=ORIENTED_EDGE('',*,*,#6870,.F.);
#9305=ORIENTED_EDGE('',*,*,#6871,.T.);
#9306=ORIENTED_EDGE('',*,*,#6870,.T.);
#9307=ORIENTED_EDGE('',*,*,#6872,.F.);
#9308=ORIENTED_EDGE('',*,*,#6751,.F.);
#9309=ORIENTED_EDGE('',*,*,#6873,.F.);
#9310=ORIENTED_EDGE('',*,*,#6758,.T.);
#9311=ORIENTED_EDGE('',*,*,#6874,.F.);
#9312=ORIENTED_EDGE('',*,*,#6875,.F.);
#9313=ORIENTED_EDGE('',*,*,#6876,.T.);
#9314=ORIENTED_EDGE('',*,*,#6875,.T.);
#9315=ORIENTED_EDGE('',*,*,#6877,.F.);
#9316=ORIENTED_EDGE('',*,*,#6878,.F.);
#9317=ORIENTED_EDGE('',*,*,#6879,.T.);
#9318=ORIENTED_EDGE('',*,*,#6878,.T.);
#9319=ORIENTED_EDGE('',*,*,#6880,.F.);
#9320=ORIENTED_EDGE('',*,*,#6765,.F.);
#9321=ORIENTED_EDGE('',*,*,#6881,.F.);
#9322=ORIENTED_EDGE('',*,*,#6772,.T.);
#9323=ORIENTED_EDGE('',*,*,#6882,.F.);
#9324=ORIENTED_EDGE('',*,*,#6883,.F.);
#9325=ORIENTED_EDGE('',*,*,#6884,.T.);
#9326=ORIENTED_EDGE('',*,*,#6883,.T.);
#9327=ORIENTED_EDGE('',*,*,#6885,.F.);
#9328=ORIENTED_EDGE('',*,*,#6886,.F.);
#9329=ORIENTED_EDGE('',*,*,#6887,.T.);
#9330=ORIENTED_EDGE('',*,*,#6886,.T.);
#9331=ORIENTED_EDGE('',*,*,#6888,.F.);
#9332=ORIENTED_EDGE('',*,*,#6779,.F.);
#9333=ORIENTED_EDGE('',*,*,#6889,.F.);
#9334=ORIENTED_EDGE('',*,*,#6786,.T.);
#9335=ORIENTED_EDGE('',*,*,#6890,.F.);
#9336=ORIENTED_EDGE('',*,*,#6891,.F.);
#9337=ORIENTED_EDGE('',*,*,#6892,.T.);
#9338=ORIENTED_EDGE('',*,*,#6891,.T.);
#9339=ORIENTED_EDGE('',*,*,#6893,.F.);
#9340=ORIENTED_EDGE('',*,*,#6894,.F.);
#9341=ORIENTED_EDGE('',*,*,#6895,.T.);
#9342=ORIENTED_EDGE('',*,*,#6894,.T.);
#9343=ORIENTED_EDGE('',*,*,#6896,.F.);
#9344=ORIENTED_EDGE('',*,*,#6793,.F.);
#9345=ORIENTED_EDGE('',*,*,#6897,.F.);
#9346=ORIENTED_EDGE('',*,*,#6800,.T.);
#9347=ORIENTED_EDGE('',*,*,#6898,.F.);
#9348=ORIENTED_EDGE('',*,*,#6899,.F.);
#9349=ORIENTED_EDGE('',*,*,#6900,.T.);
#9350=ORIENTED_EDGE('',*,*,#6899,.T.);
#9351=ORIENTED_EDGE('',*,*,#6901,.F.);
#9352=ORIENTED_EDGE('',*,*,#6902,.F.);
#9353=ORIENTED_EDGE('',*,*,#6903,.T.);
#9354=ORIENTED_EDGE('',*,*,#6902,.T.);
#9355=ORIENTED_EDGE('',*,*,#6904,.F.);
#9356=ORIENTED_EDGE('',*,*,#6807,.F.);
#9357=ORIENTED_EDGE('',*,*,#6905,.F.);
#9358=ORIENTED_EDGE('',*,*,#6814,.T.);
#9359=ORIENTED_EDGE('',*,*,#6906,.F.);
#9360=ORIENTED_EDGE('',*,*,#6907,.F.);
#9361=ORIENTED_EDGE('',*,*,#6908,.T.);
#9362=ORIENTED_EDGE('',*,*,#6907,.T.);
#9363=ORIENTED_EDGE('',*,*,#6909,.F.);
#9364=ORIENTED_EDGE('',*,*,#6910,.F.);
#9365=ORIENTED_EDGE('',*,*,#6911,.T.);
#9366=ORIENTED_EDGE('',*,*,#6910,.T.);
#9367=ORIENTED_EDGE('',*,*,#6912,.F.);
#9368=ORIENTED_EDGE('',*,*,#6821,.F.);
#9369=ORIENTED_EDGE('',*,*,#6913,.F.);
#9370=ORIENTED_EDGE('',*,*,#6828,.T.);
#9371=ORIENTED_EDGE('',*,*,#6914,.F.);
#9372=ORIENTED_EDGE('',*,*,#6915,.F.);
#9373=ORIENTED_EDGE('',*,*,#6916,.T.);
#9374=ORIENTED_EDGE('',*,*,#6915,.T.);
#9375=ORIENTED_EDGE('',*,*,#6917,.F.);
#9376=ORIENTED_EDGE('',*,*,#6918,.F.);
#9377=ORIENTED_EDGE('',*,*,#6919,.T.);
#9378=ORIENTED_EDGE('',*,*,#6918,.T.);
#9379=ORIENTED_EDGE('',*,*,#6920,.F.);
#9380=ORIENTED_EDGE('',*,*,#6835,.F.);
#9381=ORIENTED_EDGE('',*,*,#6921,.F.);
#9382=ORIENTED_EDGE('',*,*,#6842,.T.);
#9383=ORIENTED_EDGE('',*,*,#6922,.F.);
#9384=ORIENTED_EDGE('',*,*,#6923,.F.);
#9385=ORIENTED_EDGE('',*,*,#6924,.T.);
#9386=ORIENTED_EDGE('',*,*,#6923,.T.);
#9387=ORIENTED_EDGE('',*,*,#6925,.F.);
#9388=ORIENTED_EDGE('',*,*,#6926,.F.);
#9389=ORIENTED_EDGE('',*,*,#6927,.T.);
#9390=ORIENTED_EDGE('',*,*,#6926,.T.);
#9391=ORIENTED_EDGE('',*,*,#6928,.F.);
#9392=ORIENTED_EDGE('',*,*,#6849,.F.);
#9393=ORIENTED_EDGE('',*,*,#6929,.F.);
#9394=ORIENTED_EDGE('',*,*,#6856,.T.);
#9395=ORIENTED_EDGE('',*,*,#6930,.F.);
#9396=ORIENTED_EDGE('',*,*,#6931,.F.);
#9397=ORIENTED_EDGE('',*,*,#6932,.T.);
#9398=ORIENTED_EDGE('',*,*,#6931,.T.);
#9399=ORIENTED_EDGE('',*,*,#6933,.F.);
#9400=ORIENTED_EDGE('',*,*,#6934,.F.);
#9401=ORIENTED_EDGE('',*,*,#6935,.T.);
#9402=ORIENTED_EDGE('',*,*,#6934,.T.);
#9403=ORIENTED_EDGE('',*,*,#6936,.F.);
#9404=ORIENTED_EDGE('',*,*,#6863,.F.);
#9405=ORIENTED_EDGE('',*,*,#6755,.F.);
#9406=ORIENTED_EDGE('',*,*,#6759,.T.);
#9407=ORIENTED_EDGE('',*,*,#6873,.T.);
#9408=ORIENTED_EDGE('',*,*,#6876,.F.);
#9409=ORIENTED_EDGE('',*,*,#6879,.F.);
#9410=ORIENTED_EDGE('',*,*,#6764,.F.);
#9411=ORIENTED_EDGE('',*,*,#6760,.F.);
#9412=ORIENTED_EDGE('',*,*,#6937,.F.);
#9413=ORIENTED_EDGE('',*,*,#6769,.F.);
#9414=ORIENTED_EDGE('',*,*,#6773,.T.);
#9415=ORIENTED_EDGE('',*,*,#6881,.T.);
#9416=ORIENTED_EDGE('',*,*,#6884,.F.);
#9417=ORIENTED_EDGE('',*,*,#6887,.F.);
#9418=ORIENTED_EDGE('',*,*,#6778,.F.);
#9419=ORIENTED_EDGE('',*,*,#6774,.F.);
#9420=ORIENTED_EDGE('',*,*,#6938,.F.);
#9421=ORIENTED_EDGE('',*,*,#6783,.F.);
#9422=ORIENTED_EDGE('',*,*,#6787,.T.);
#9423=ORIENTED_EDGE('',*,*,#6889,.T.);
#9424=ORIENTED_EDGE('',*,*,#6892,.F.);
#9425=ORIENTED_EDGE('',*,*,#6895,.F.);
#9426=ORIENTED_EDGE('',*,*,#6792,.F.);
#9427=ORIENTED_EDGE('',*,*,#6788,.F.);
#9428=ORIENTED_EDGE('',*,*,#6939,.F.);
#9429=ORIENTED_EDGE('',*,*,#6797,.F.);
#9430=ORIENTED_EDGE('',*,*,#6801,.T.);
#9431=ORIENTED_EDGE('',*,*,#6897,.T.);
#9432=ORIENTED_EDGE('',*,*,#6900,.F.);
#9433=ORIENTED_EDGE('',*,*,#6903,.F.);
#9434=ORIENTED_EDGE('',*,*,#6806,.F.);
#9435=ORIENTED_EDGE('',*,*,#6802,.F.);
#9436=ORIENTED_EDGE('',*,*,#6940,.F.);
#9437=ORIENTED_EDGE('',*,*,#6811,.F.);
#9438=ORIENTED_EDGE('',*,*,#6815,.T.);
#9439=ORIENTED_EDGE('',*,*,#6905,.T.);
#9440=ORIENTED_EDGE('',*,*,#6908,.F.);
#9441=ORIENTED_EDGE('',*,*,#6911,.F.);
#9442=ORIENTED_EDGE('',*,*,#6820,.F.);
#9443=ORIENTED_EDGE('',*,*,#6816,.F.);
#9444=ORIENTED_EDGE('',*,*,#6941,.F.);
#9445=ORIENTED_EDGE('',*,*,#6825,.F.);
#9446=ORIENTED_EDGE('',*,*,#6829,.T.);
#9447=ORIENTED_EDGE('',*,*,#6913,.T.);
#9448=ORIENTED_EDGE('',*,*,#6916,.F.);
#9449=ORIENTED_EDGE('',*,*,#6919,.F.);
#9450=ORIENTED_EDGE('',*,*,#6834,.F.);
#9451=ORIENTED_EDGE('',*,*,#6830,.F.);
#9452=ORIENTED_EDGE('',*,*,#6942,.F.);
#9453=ORIENTED_EDGE('',*,*,#6839,.F.);
#9454=ORIENTED_EDGE('',*,*,#6843,.T.);
#9455=ORIENTED_EDGE('',*,*,#6921,.T.);
#9456=ORIENTED_EDGE('',*,*,#6924,.F.);
#9457=ORIENTED_EDGE('',*,*,#6927,.F.);
#9458=ORIENTED_EDGE('',*,*,#6848,.F.);
#9459=ORIENTED_EDGE('',*,*,#6844,.F.);
#9460=ORIENTED_EDGE('',*,*,#6943,.F.);
#9461=ORIENTED_EDGE('',*,*,#6853,.F.);
#9462=ORIENTED_EDGE('',*,*,#6857,.T.);
#9463=ORIENTED_EDGE('',*,*,#6929,.T.);
#9464=ORIENTED_EDGE('',*,*,#6932,.F.);
#9465=ORIENTED_EDGE('',*,*,#6935,.F.);
#9466=ORIENTED_EDGE('',*,*,#6862,.F.);
#9467=ORIENTED_EDGE('',*,*,#6858,.F.);
#9468=ORIENTED_EDGE('',*,*,#6944,.F.);
#9469=ORIENTED_EDGE('',*,*,#6945,.F.);
#9470=ORIENTED_EDGE('',*,*,#6946,.T.);
#9471=ORIENTED_EDGE('',*,*,#6947,.T.);
#9472=ORIENTED_EDGE('',*,*,#6948,.F.);
#9473=ORIENTED_EDGE('',*,*,#6949,.F.);
#9474=ORIENTED_EDGE('',*,*,#6950,.F.);
#9475=ORIENTED_EDGE('',*,*,#6951,.F.);
#9476=ORIENTED_EDGE('',*,*,#6952,.F.);
#9477=ORIENTED_EDGE('',*,*,#6741,.F.);
#9478=ORIENTED_EDGE('',*,*,#6745,.T.);
#9479=ORIENTED_EDGE('',*,*,#6865,.T.);
#9480=ORIENTED_EDGE('',*,*,#6868,.F.);
#9481=ORIENTED_EDGE('',*,*,#6871,.F.);
#9482=ORIENTED_EDGE('',*,*,#6750,.F.);
#9483=ORIENTED_EDGE('',*,*,#6746,.F.);
#9484=ORIENTED_EDGE('',*,*,#6953,.F.);
#9485=ORIENTED_EDGE('',*,*,#6738,.T.);
#9486=ORIENTED_EDGE('',*,*,#6954,.T.);
#9487=ORIENTED_EDGE('',*,*,#6955,.F.);
#9488=ORIENTED_EDGE('',*,*,#6956,.T.);
#9489=ORIENTED_EDGE('',*,*,#6957,.T.);
#9490=ORIENTED_EDGE('',*,*,#6958,.T.);
#9491=ORIENTED_EDGE('',*,*,#6959,.T.);
#9492=ORIENTED_EDGE('',*,*,#6960,.T.);
#9493=ORIENTED_EDGE('',*,*,#6961,.F.);
#9494=ORIENTED_EDGE('',*,*,#6962,.T.);
#9495=ORIENTED_EDGE('',*,*,#6860,.F.);
#9496=ORIENTED_EDGE('',*,*,#6864,.T.);
#9497=ORIENTED_EDGE('',*,*,#6936,.T.);
#9498=ORIENTED_EDGE('',*,*,#6933,.T.);
#9499=ORIENTED_EDGE('',*,*,#6930,.T.);
#9500=ORIENTED_EDGE('',*,*,#6855,.T.);
#9501=ORIENTED_EDGE('',*,*,#6851,.F.);
#9502=ORIENTED_EDGE('',*,*,#6963,.T.);
#9503=ORIENTED_EDGE('',*,*,#6846,.F.);
#9504=ORIENTED_EDGE('',*,*,#6850,.T.);
#9505=ORIENTED_EDGE('',*,*,#6928,.T.);
#9506=ORIENTED_EDGE('',*,*,#6925,.T.);
#9507=ORIENTED_EDGE('',*,*,#6922,.T.);
#9508=ORIENTED_EDGE('',*,*,#6841,.T.);
#9509=ORIENTED_EDGE('',*,*,#6837,.F.);
#9510=ORIENTED_EDGE('',*,*,#6964,.T.);
#9511=ORIENTED_EDGE('',*,*,#6832,.F.);
#9512=ORIENTED_EDGE('',*,*,#6836,.T.);
#9513=ORIENTED_EDGE('',*,*,#6920,.T.);
#9514=ORIENTED_EDGE('',*,*,#6917,.T.);
#9515=ORIENTED_EDGE('',*,*,#6914,.T.);
#9516=ORIENTED_EDGE('',*,*,#6827,.T.);
#9517=ORIENTED_EDGE('',*,*,#6823,.F.);
#9518=ORIENTED_EDGE('',*,*,#6965,.T.);
#9519=ORIENTED_EDGE('',*,*,#6818,.F.);
#9520=ORIENTED_EDGE('',*,*,#6822,.T.);
#9521=ORIENTED_EDGE('',*,*,#6912,.T.);
#9522=ORIENTED_EDGE('',*,*,#6909,.T.);
#9523=ORIENTED_EDGE('',*,*,#6906,.T.);
#9524=ORIENTED_EDGE('',*,*,#6813,.T.);
#9525=ORIENTED_EDGE('',*,*,#6809,.F.);
#9526=ORIENTED_EDGE('',*,*,#6966,.T.);
#9527=ORIENTED_EDGE('',*,*,#6804,.F.);
#9528=ORIENTED_EDGE('',*,*,#6808,.T.);
#9529=ORIENTED_EDGE('',*,*,#6904,.T.);
#9530=ORIENTED_EDGE('',*,*,#6901,.T.);
#9531=ORIENTED_EDGE('',*,*,#6898,.T.);
#9532=ORIENTED_EDGE('',*,*,#6799,.T.);
#9533=ORIENTED_EDGE('',*,*,#6795,.F.);
#9534=ORIENTED_EDGE('',*,*,#6967,.T.);
#9535=ORIENTED_EDGE('',*,*,#6790,.F.);
#9536=ORIENTED_EDGE('',*,*,#6794,.T.);
#9537=ORIENTED_EDGE('',*,*,#6896,.T.);
#9538=ORIENTED_EDGE('',*,*,#6893,.T.);
#9539=ORIENTED_EDGE('',*,*,#6890,.T.);
#9540=ORIENTED_EDGE('',*,*,#6785,.T.);
#9541=ORIENTED_EDGE('',*,*,#6781,.F.);
#9542=ORIENTED_EDGE('',*,*,#6968,.T.);
#9543=ORIENTED_EDGE('',*,*,#6776,.F.);
#9544=ORIENTED_EDGE('',*,*,#6780,.T.);
#9545=ORIENTED_EDGE('',*,*,#6888,.T.);
#9546=ORIENTED_EDGE('',*,*,#6885,.T.);
#9547=ORIENTED_EDGE('',*,*,#6882,.T.);
#9548=ORIENTED_EDGE('',*,*,#6771,.T.);
#9549=ORIENTED_EDGE('',*,*,#6767,.F.);
#9550=ORIENTED_EDGE('',*,*,#6969,.T.);
#9551=ORIENTED_EDGE('',*,*,#6762,.F.);
#9552=ORIENTED_EDGE('',*,*,#6766,.T.);
#9553=ORIENTED_EDGE('',*,*,#6880,.T.);
#9554=ORIENTED_EDGE('',*,*,#6877,.T.);
#9555=ORIENTED_EDGE('',*,*,#6874,.T.);
#9556=ORIENTED_EDGE('',*,*,#6757,.T.);
#9557=ORIENTED_EDGE('',*,*,#6753,.F.);
#9558=ORIENTED_EDGE('',*,*,#6970,.T.);
#9559=ORIENTED_EDGE('',*,*,#6748,.F.);
#9560=ORIENTED_EDGE('',*,*,#6752,.T.);
#9561=ORIENTED_EDGE('',*,*,#6872,.T.);
#9562=ORIENTED_EDGE('',*,*,#6869,.T.);
#9563=ORIENTED_EDGE('',*,*,#6866,.T.);
#9564=ORIENTED_EDGE('',*,*,#6743,.T.);
#9565=ORIENTED_EDGE('',*,*,#6739,.F.);
#9566=ORIENTED_EDGE('',*,*,#6733,.T.);
#9567=ORIENTED_EDGE('',*,*,#6861,.F.);
#9568=ORIENTED_EDGE('',*,*,#6962,.F.);
#9569=ORIENTED_EDGE('',*,*,#6971,.F.);
#9570=ORIENTED_EDGE('',*,*,#6944,.T.);
#9571=ORIENTED_EDGE('',*,*,#6847,.F.);
#9572=ORIENTED_EDGE('',*,*,#6963,.F.);
#9573=ORIENTED_EDGE('',*,*,#6854,.F.);
#9574=ORIENTED_EDGE('',*,*,#6943,.T.);
#9575=ORIENTED_EDGE('',*,*,#6833,.F.);
#9576=ORIENTED_EDGE('',*,*,#6964,.F.);
#9577=ORIENTED_EDGE('',*,*,#6840,.F.);
#9578=ORIENTED_EDGE('',*,*,#6942,.T.);
#9579=ORIENTED_EDGE('',*,*,#6819,.F.);
#9580=ORIENTED_EDGE('',*,*,#6965,.F.);
#9581=ORIENTED_EDGE('',*,*,#6826,.F.);
#9582=ORIENTED_EDGE('',*,*,#6941,.T.);
#9583=ORIENTED_EDGE('',*,*,#6805,.F.);
#9584=ORIENTED_EDGE('',*,*,#6966,.F.);
#9585=ORIENTED_EDGE('',*,*,#6812,.F.);
#9586=ORIENTED_EDGE('',*,*,#6940,.T.);
#9587=ORIENTED_EDGE('',*,*,#6791,.F.);
#9588=ORIENTED_EDGE('',*,*,#6967,.F.);
#9589=ORIENTED_EDGE('',*,*,#6798,.F.);
#9590=ORIENTED_EDGE('',*,*,#6939,.T.);
#9591=ORIENTED_EDGE('',*,*,#6777,.F.);
#9592=ORIENTED_EDGE('',*,*,#6968,.F.);
#9593=ORIENTED_EDGE('',*,*,#6784,.F.);
#9594=ORIENTED_EDGE('',*,*,#6938,.T.);
#9595=ORIENTED_EDGE('',*,*,#6763,.F.);
#9596=ORIENTED_EDGE('',*,*,#6969,.F.);
#9597=ORIENTED_EDGE('',*,*,#6770,.F.);
#9598=ORIENTED_EDGE('',*,*,#6937,.T.);
#9599=ORIENTED_EDGE('',*,*,#6749,.F.);
#9600=ORIENTED_EDGE('',*,*,#6970,.F.);
#9601=ORIENTED_EDGE('',*,*,#6756,.F.);
#9602=ORIENTED_EDGE('',*,*,#6953,.T.);
#9603=ORIENTED_EDGE('',*,*,#6961,.T.);
#9604=ORIENTED_EDGE('',*,*,#6972,.T.);
#9605=ORIENTED_EDGE('',*,*,#6945,.T.);
#9606=ORIENTED_EDGE('',*,*,#6971,.T.);
#9607=ORIENTED_EDGE('',*,*,#6972,.F.);
#9608=ORIENTED_EDGE('',*,*,#6960,.F.);
#9609=ORIENTED_EDGE('',*,*,#6973,.F.);
#9610=ORIENTED_EDGE('',*,*,#6946,.F.);
#9611=ORIENTED_EDGE('',*,*,#6951,.T.);
#9612=ORIENTED_EDGE('',*,*,#6974,.T.);
#9613=ORIENTED_EDGE('',*,*,#6955,.T.);
#9614=ORIENTED_EDGE('',*,*,#6975,.T.);
#9615=ORIENTED_EDGE('',*,*,#6974,.F.);
#9616=ORIENTED_EDGE('',*,*,#6950,.T.);
#9617=ORIENTED_EDGE('',*,*,#6976,.T.);
#9618=ORIENTED_EDGE('',*,*,#6956,.F.);
#9619=ORIENTED_EDGE('',*,*,#6947,.F.);
#9620=ORIENTED_EDGE('',*,*,#6973,.T.);
#9621=ORIENTED_EDGE('',*,*,#6959,.F.);
#9622=ORIENTED_EDGE('',*,*,#6977,.F.);
#9623=ORIENTED_EDGE('',*,*,#6948,.T.);
#9624=ORIENTED_EDGE('',*,*,#6977,.T.);
#9625=ORIENTED_EDGE('',*,*,#6958,.F.);
#9626=ORIENTED_EDGE('',*,*,#6978,.F.);
#9627=ORIENTED_EDGE('',*,*,#6949,.T.);
#9628=ORIENTED_EDGE('',*,*,#6978,.T.);
#9629=ORIENTED_EDGE('',*,*,#6957,.F.);
#9630=ORIENTED_EDGE('',*,*,#6976,.F.);
#9631=ORIENTED_EDGE('',*,*,#6742,.F.);
#9632=ORIENTED_EDGE('',*,*,#6952,.T.);
#9633=ORIENTED_EDGE('',*,*,#6975,.F.);
#9634=ORIENTED_EDGE('',*,*,#6954,.F.);
#12101=CYLINDRICAL_SURFACE('',#13477,7.50000000000001);
#12102=CYLINDRICAL_SURFACE('',#13480,7.50000000000001);
#12103=CYLINDRICAL_SURFACE('',#13485,1.);
#12104=CYLINDRICAL_SURFACE('',#13489,1.);
#12105=CYLINDRICAL_SURFACE('',#13493,1.);
#12106=CYLINDRICAL_SURFACE('',#13497,1.);
#12107=CYLINDRICAL_SURFACE('',#13501,1.);
#12108=CYLINDRICAL_SURFACE('',#13505,1.);
#12109=CYLINDRICAL_SURFACE('',#13509,1.);
#12110=CYLINDRICAL_SURFACE('',#13513,1.);
#12111=CYLINDRICAL_SURFACE('',#13517,1.);
#12112=CYLINDRICAL_SURFACE('',#13521,1.);
#12113=CYLINDRICAL_SURFACE('',#13525,1.);
#12114=CYLINDRICAL_SURFACE('',#13529,1.);
#12115=CYLINDRICAL_SURFACE('',#13533,1.);
#12116=CYLINDRICAL_SURFACE('',#13537,1.);
#12117=CYLINDRICAL_SURFACE('',#13541,1.);
#12118=CYLINDRICAL_SURFACE('',#13545,1.);
#12119=CYLINDRICAL_SURFACE('',#13549,1.);
#12120=CYLINDRICAL_SURFACE('',#13553,1.);
#12121=CYLINDRICAL_SURFACE('',#13557,23.9999999999999);
#12122=CYLINDRICAL_SURFACE('',#13560,23.9999999999999);
#12123=CYLINDRICAL_SURFACE('',#13563,23.9999999999999);
#12124=CYLINDRICAL_SURFACE('',#13566,23.9999999999999);
#12125=CYLINDRICAL_SURFACE('',#13569,23.9999999999999);
#12126=CYLINDRICAL_SURFACE('',#13572,23.9999999999999);
#12127=CYLINDRICAL_SURFACE('',#13575,23.9999999999999);
#12128=CYLINDRICAL_SURFACE('',#13578,23.9999999999999);
#12129=CYLINDRICAL_SURFACE('',#13581,23.9999999999999);
#12130=CYLINDRICAL_SURFACE('',#13612,15.372);
#12131=CYLINDRICAL_SURFACE('',#13613,15.372);
#12132=CYLINDRICAL_SURFACE('',#13614,15.372);
#12133=CYLINDRICAL_SURFACE('',#13615,15.372);
#12134=CYLINDRICAL_SURFACE('',#13616,15.372);
#12135=CYLINDRICAL_SURFACE('',#13617,15.372);
#12136=CYLINDRICAL_SURFACE('',#13618,15.372);
#12137=CYLINDRICAL_SURFACE('',#13619,15.372);
#12138=CYLINDRICAL_SURFACE('',#13620,15.372);
#12139=CYLINDRICAL_SURFACE('',#13621,1.);
#12140=CYLINDRICAL_SURFACE('',#13623,1.);
#12141=CYLINDRICAL_SURFACE('',#13625,23.9999999999999);
#12142=CYLINDRICAL_SURFACE('',#13626,15.372);
#12465=ADVANCED_FACE('',(#1453),#12101,.T.);
#12466=ADVANCED_FACE('',(#1454),#12102,.T.);
#12467=ADVANCED_FACE('',(#1455),#1051,.F.);
#12468=ADVANCED_FACE('',(#1456),#1052,.T.);
#12469=ADVANCED_FACE('',(#1457),#12103,.F.);
#12470=ADVANCED_FACE('',(#1458),#1053,.T.);
#12471=ADVANCED_FACE('',(#1459),#12104,.F.);
#12472=ADVANCED_FACE('',(#1460),#1054,.T.);
#12473=ADVANCED_FACE('',(#1461),#12105,.F.);
#12474=ADVANCED_FACE('',(#1462),#1055,.T.);
#12475=ADVANCED_FACE('',(#1463),#12106,.F.);
#12476=ADVANCED_FACE('',(#1464),#1056,.T.);
#12477=ADVANCED_FACE('',(#1465),#12107,.F.);
#12478=ADVANCED_FACE('',(#1466),#1057,.T.);
#12479=ADVANCED_FACE('',(#1467),#12108,.F.);
#12480=ADVANCED_FACE('',(#1468),#1058,.T.);
#12481=ADVANCED_FACE('',(#1469),#12109,.F.);
#12482=ADVANCED_FACE('',(#1470),#1059,.T.);
#12483=ADVANCED_FACE('',(#1471),#12110,.F.);
#12484=ADVANCED_FACE('',(#1472),#1060,.T.);
#12485=ADVANCED_FACE('',(#1473),#12111,.F.);
#12486=ADVANCED_FACE('',(#1474),#1061,.T.);
#12487=ADVANCED_FACE('',(#1475),#12112,.F.);
#12488=ADVANCED_FACE('',(#1476),#1062,.T.);
#12489=ADVANCED_FACE('',(#1477),#12113,.F.);
#12490=ADVANCED_FACE('',(#1478),#1063,.T.);
#12491=ADVANCED_FACE('',(#1479),#12114,.F.);
#12492=ADVANCED_FACE('',(#1480),#1064,.T.);
#12493=ADVANCED_FACE('',(#1481),#12115,.F.);
#12494=ADVANCED_FACE('',(#1482),#1065,.T.);
#12495=ADVANCED_FACE('',(#1483),#12116,.F.);
#12496=ADVANCED_FACE('',(#1484),#1066,.T.);
#12497=ADVANCED_FACE('',(#1485),#12117,.F.);
#12498=ADVANCED_FACE('',(#1486),#1067,.T.);
#12499=ADVANCED_FACE('',(#1487),#12118,.F.);
#12500=ADVANCED_FACE('',(#1488),#1068,.T.);
#12501=ADVANCED_FACE('',(#1489),#12119,.F.);
#12502=ADVANCED_FACE('',(#1490),#1069,.T.);
#12503=ADVANCED_FACE('',(#1491),#12120,.F.);
#12504=ADVANCED_FACE('',(#1492),#1070,.T.);
#12505=ADVANCED_FACE('',(#1493),#987,.T.);
#12506=ADVANCED_FACE('',(#1494),#12121,.T.);
#12507=ADVANCED_FACE('',(#1495),#988,.T.);
#12508=ADVANCED_FACE('',(#1496),#989,.T.);
#12509=ADVANCED_FACE('',(#1497),#12122,.T.);
#12510=ADVANCED_FACE('',(#1498),#990,.T.);
#12511=ADVANCED_FACE('',(#1499),#991,.T.);
#12512=ADVANCED_FACE('',(#1500),#12123,.T.);
#12513=ADVANCED_FACE('',(#1501),#992,.T.);
#12514=ADVANCED_FACE('',(#1502),#993,.T.);
#12515=ADVANCED_FACE('',(#1503),#12124,.T.);
#12516=ADVANCED_FACE('',(#1504),#994,.T.);
#12517=ADVANCED_FACE('',(#1505),#995,.T.);
#12518=ADVANCED_FACE('',(#1506),#12125,.T.);
#12519=ADVANCED_FACE('',(#1507),#996,.T.);
#12520=ADVANCED_FACE('',(#1508),#997,.T.);
#12521=ADVANCED_FACE('',(#1509),#12126,.T.);
#12522=ADVANCED_FACE('',(#1510),#998,.T.);
#12523=ADVANCED_FACE('',(#1511),#999,.T.);
#12524=ADVANCED_FACE('',(#1512),#12127,.T.);
#12525=ADVANCED_FACE('',(#1513),#1000,.T.);
#12526=ADVANCED_FACE('',(#1514),#1001,.T.);
#12527=ADVANCED_FACE('',(#1515),#12128,.T.);
#12528=ADVANCED_FACE('',(#1516),#1002,.T.);
#12529=ADVANCED_FACE('',(#1517),#1003,.T.);
#12530=ADVANCED_FACE('',(#1518),#12129,.T.);
#12531=ADVANCED_FACE('',(#1519),#1004,.T.);
#12532=ADVANCED_FACE('',(#1520,#281),#1071,.F.);
#12533=ADVANCED_FACE('',(#1521,#282),#1072,.T.);
#12534=ADVANCED_FACE('',(#1522),#12130,.T.);
#12535=ADVANCED_FACE('',(#1523),#12131,.T.);
#12536=ADVANCED_FACE('',(#1524),#12132,.T.);
#12537=ADVANCED_FACE('',(#1525),#12133,.T.);
#12538=ADVANCED_FACE('',(#1526),#12134,.T.);
#12539=ADVANCED_FACE('',(#1527),#12135,.T.);
#12540=ADVANCED_FACE('',(#1528),#12136,.T.);
#12541=ADVANCED_FACE('',(#1529),#12137,.T.);
#12542=ADVANCED_FACE('',(#1530),#12138,.T.);
#12543=ADVANCED_FACE('',(#1531),#12139,.F.);
#12544=ADVANCED_FACE('',(#1532),#1073,.T.);
#12545=ADVANCED_FACE('',(#1533),#12140,.F.);
#12546=ADVANCED_FACE('',(#1534),#1074,.T.);
#12547=ADVANCED_FACE('',(#1535),#1005,.T.);
#12548=ADVANCED_FACE('',(#1536),#12141,.T.);
#12549=ADVANCED_FACE('',(#1537),#1006,.T.);
#12550=ADVANCED_FACE('',(#1538),#12142,.T.);
#13052=CLOSED_SHELL('',(#12465,#12466,#12467,#12468,#12469,#12470,#12471,
#12472,#12473,#12474,#12475,#12476,#12477,#12478,#12479,#12480,#12481,#12482,
#12483,#12484,#12485,#12486,#12487,#12488,#12489,#12490,#12491,#12492,#12493,
#12494,#12495,#12496,#12497,#12498,#12499,#12500,#12501,#12502,#12503,#12504,
#12505,#12506,#12507,#12508,#12509,#12510,#12511,#12512,#12513,#12514,#12515,
#12516,#12517,#12518,#12519,#12520,#12521,#12522,#12523,#12524,#12525,#12526,
#12527,#12528,#12529,#12530,#12531,#12532,#12533,#12534,#12535,#12536,#12537,
#12538,#12539,#12540,#12541,#12542,#12543,#12544,#12545,#12546,#12547,#12548,
#12549,#12550));
#13476=AXIS2_PLACEMENT_3D('',#31617,#15739,#15740);
#13477=AXIS2_PLACEMENT_3D('',#31618,#15741,#15742);
#13478=AXIS2_PLACEMENT_3D('',#31620,#15743,#15744);
#13479=AXIS2_PLACEMENT_3D('',#31623,#15746,#15747);
#13480=AXIS2_PLACEMENT_3D('',#31624,#15748,#15749);
#13481=AXIS2_PLACEMENT_3D('',#31626,#15750,#15751);
#13482=AXIS2_PLACEMENT_3D('',#31629,#15753,#15754);
#13483=AXIS2_PLACEMENT_3D('',#31630,#15755,#15756);
#13484=AXIS2_PLACEMENT_3D('',#31631,#15757,#15758);
#13485=AXIS2_PLACEMENT_3D('',#31632,#15759,#15760);
#13486=AXIS2_PLACEMENT_3D('',#31635,#15761,#15762);
#13487=AXIS2_PLACEMENT_3D('',#31639,#15764,#15765);
#13488=AXIS2_PLACEMENT_3D('',#31641,#15767,#15768);
#13489=AXIS2_PLACEMENT_3D('',#31647,#15772,#15773);
#13490=AXIS2_PLACEMENT_3D('',#31650,#15774,#15775);
#13491=AXIS2_PLACEMENT_3D('',#31654,#15777,#15778);
#13492=AXIS2_PLACEMENT_3D('',#31656,#15780,#15781);
#13493=AXIS2_PLACEMENT_3D('',#31662,#15785,#15786);
#13494=AXIS2_PLACEMENT_3D('',#31665,#15787,#15788);
#13495=AXIS2_PLACEMENT_3D('',#31669,#15790,#15791);
#13496=AXIS2_PLACEMENT_3D('',#31671,#15793,#15794);
#13497=AXIS2_PLACEMENT_3D('',#31677,#15798,#15799);
#13498=AXIS2_PLACEMENT_3D('',#31680,#15800,#15801);
#13499=AXIS2_PLACEMENT_3D('',#31684,#15803,#15804);
#13500=AXIS2_PLACEMENT_3D('',#31686,#15806,#15807);
#13501=AXIS2_PLACEMENT_3D('',#31692,#15811,#15812);
#13502=AXIS2_PLACEMENT_3D('',#31695,#15813,#15814);
#13503=AXIS2_PLACEMENT_3D('',#31699,#15816,#15817);
#13504=AXIS2_PLACEMENT_3D('',#31701,#15819,#15820);
#13505=AXIS2_PLACEMENT_3D('',#31707,#15824,#15825);
#13506=AXIS2_PLACEMENT_3D('',#31710,#15826,#15827);
#13507=AXIS2_PLACEMENT_3D('',#31714,#15829,#15830);
#13508=AXIS2_PLACEMENT_3D('',#31716,#15832,#15833);
#13509=AXIS2_PLACEMENT_3D('',#31722,#15837,#15838);
#13510=AXIS2_PLACEMENT_3D('',#31725,#15839,#15840);
#13511=AXIS2_PLACEMENT_3D('',#31729,#15842,#15843);
#13512=AXIS2_PLACEMENT_3D('',#31731,#15845,#15846);
#13513=AXIS2_PLACEMENT_3D('',#31737,#15850,#15851);
#13514=AXIS2_PLACEMENT_3D('',#31740,#15852,#15853);
#13515=AXIS2_PLACEMENT_3D('',#31744,#15855,#15856);
#13516=AXIS2_PLACEMENT_3D('',#31746,#15858,#15859);
#13517=AXIS2_PLACEMENT_3D('',#31752,#15863,#15864);
#13518=AXIS2_PLACEMENT_3D('',#31755,#15865,#15866);
#13519=AXIS2_PLACEMENT_3D('',#31759,#15868,#15869);
#13520=AXIS2_PLACEMENT_3D('',#31761,#15871,#15872);
#13521=AXIS2_PLACEMENT_3D('',#31767,#15876,#15877);
#13522=AXIS2_PLACEMENT_3D('',#31770,#15878,#15879);
#13523=AXIS2_PLACEMENT_3D('',#31774,#15881,#15882);
#13524=AXIS2_PLACEMENT_3D('',#31776,#15884,#15885);
#13525=AXIS2_PLACEMENT_3D('',#31782,#15889,#15890);
#13526=AXIS2_PLACEMENT_3D('',#31785,#15891,#15892);
#13527=AXIS2_PLACEMENT_3D('',#31789,#15894,#15895);
#13528=AXIS2_PLACEMENT_3D('',#31791,#15897,#15898);
#13529=AXIS2_PLACEMENT_3D('',#31797,#15902,#15903);
#13530=AXIS2_PLACEMENT_3D('',#31800,#15904,#15905);
#13531=AXIS2_PLACEMENT_3D('',#31804,#15907,#15908);
#13532=AXIS2_PLACEMENT_3D('',#31806,#15910,#15911);
#13533=AXIS2_PLACEMENT_3D('',#31812,#15915,#15916);
#13534=AXIS2_PLACEMENT_3D('',#31815,#15917,#15918);
#13535=AXIS2_PLACEMENT_3D('',#31819,#15920,#15921);
#13536=AXIS2_PLACEMENT_3D('',#31821,#15923,#15924);
#13537=AXIS2_PLACEMENT_3D('',#31827,#15928,#15929);
#13538=AXIS2_PLACEMENT_3D('',#31830,#15930,#15931);
#13539=AXIS2_PLACEMENT_3D('',#31834,#15933,#15934);
#13540=AXIS2_PLACEMENT_3D('',#31836,#15936,#15937);
#13541=AXIS2_PLACEMENT_3D('',#31842,#15941,#15942);
#13542=AXIS2_PLACEMENT_3D('',#31845,#15943,#15944);
#13543=AXIS2_PLACEMENT_3D('',#31849,#15946,#15947);
#13544=AXIS2_PLACEMENT_3D('',#31851,#15949,#15950);
#13545=AXIS2_PLACEMENT_3D('',#31857,#15954,#15955);
#13546=AXIS2_PLACEMENT_3D('',#31860,#15956,#15957);
#13547=AXIS2_PLACEMENT_3D('',#31864,#15959,#15960);
#13548=AXIS2_PLACEMENT_3D('',#31866,#15962,#15963);
#13549=AXIS2_PLACEMENT_3D('',#31872,#15967,#15968);
#13550=AXIS2_PLACEMENT_3D('',#31875,#15969,#15970);
#13551=AXIS2_PLACEMENT_3D('',#31879,#15972,#15973);
#13552=AXIS2_PLACEMENT_3D('',#31881,#15975,#15976);
#13553=AXIS2_PLACEMENT_3D('',#31887,#15980,#15981);
#13554=AXIS2_PLACEMENT_3D('',#31890,#15982,#15983);
#13555=AXIS2_PLACEMENT_3D('',#31894,#15985,#15986);
#13556=AXIS2_PLACEMENT_3D('',#31896,#15988,#15989);
#13557=AXIS2_PLACEMENT_3D('',#32204,#15994,#15995);
#13558=AXIS2_PLACEMENT_3D('',#32206,#15996,#15997);
#13559=AXIS2_PLACEMENT_3D('',#32208,#15998,#15999);
#13560=AXIS2_PLACEMENT_3D('',#32810,#16002,#16003);
#13561=AXIS2_PLACEMENT_3D('',#32812,#16004,#16005);
#13562=AXIS2_PLACEMENT_3D('',#32814,#16006,#16007);
#13563=AXIS2_PLACEMENT_3D('',#33416,#16010,#16011);
#13564=AXIS2_PLACEMENT_3D('',#33418,#16012,#16013);
#13565=AXIS2_PLACEMENT_3D('',#33420,#16014,#16015);
#13566=AXIS2_PLACEMENT_3D('',#34022,#16018,#16019);
#13567=AXIS2_PLACEMENT_3D('',#34024,#16020,#16021);
#13568=AXIS2_PLACEMENT_3D('',#34026,#16022,#16023);
#13569=AXIS2_PLACEMENT_3D('',#34628,#16026,#16027);
#13570=AXIS2_PLACEMENT_3D('',#34630,#16028,#16029);
#13571=AXIS2_PLACEMENT_3D('',#34632,#16030,#16031);
#13572=AXIS2_PLACEMENT_3D('',#35234,#16034,#16035);
#13573=AXIS2_PLACEMENT_3D('',#35236,#16036,#16037);
#13574=AXIS2_PLACEMENT_3D('',#35238,#16038,#16039);
#13575=AXIS2_PLACEMENT_3D('',#35840,#16042,#16043);
#13576=AXIS2_PLACEMENT_3D('',#35842,#16044,#16045);
#13577=AXIS2_PLACEMENT_3D('',#35844,#16046,#16047);
#13578=AXIS2_PLACEMENT_3D('',#36446,#16050,#16051);
#13579=AXIS2_PLACEMENT_3D('',#36448,#16052,#16053);
#13580=AXIS2_PLACEMENT_3D('',#36450,#16054,#16055);
#13581=AXIS2_PLACEMENT_3D('',#37052,#16058,#16059);
#13582=AXIS2_PLACEMENT_3D('',#37054,#16060,#16061);
#13583=AXIS2_PLACEMENT_3D('',#37056,#16062,#16063);
#13584=AXIS2_PLACEMENT_3D('',#37356,#16065,#16066);
#13585=AXIS2_PLACEMENT_3D('',#37357,#16067,#16068);
#13586=AXIS2_PLACEMENT_3D('',#37358,#16069,#16070);
#13587=AXIS2_PLACEMENT_3D('',#37359,#16071,#16072);
#13588=AXIS2_PLACEMENT_3D('',#37360,#16073,#16074);
#13589=AXIS2_PLACEMENT_3D('',#37361,#16075,#16076);
#13590=AXIS2_PLACEMENT_3D('',#37362,#16077,#16078);
#13591=AXIS2_PLACEMENT_3D('',#37363,#16079,#16080);
#13592=AXIS2_PLACEMENT_3D('',#37365,#16081,#16082);
#13593=AXIS2_PLACEMENT_3D('',#37367,#16083,#16084);
#13594=AXIS2_PLACEMENT_3D('',#37446,#16086,#16087);
#13595=AXIS2_PLACEMENT_3D('',#37525,#16089,#16090);
#13596=AXIS2_PLACEMENT_3D('',#37526,#16091,#16092);
#13597=AXIS2_PLACEMENT_3D('',#37527,#16093,#16094);
#13598=AXIS2_PLACEMENT_3D('',#37528,#16095,#16096);
#13599=AXIS2_PLACEMENT_3D('',#37530,#16097,#16098);
#13600=AXIS2_PLACEMENT_3D('',#37532,#16099,#16100);
#13601=AXIS2_PLACEMENT_3D('',#37611,#16102,#16103);
#13602=AXIS2_PLACEMENT_3D('',#37691,#16105,#16106);
#13603=AXIS2_PLACEMENT_3D('',#37692,#16107,#16108);
#13604=AXIS2_PLACEMENT_3D('',#37693,#16109,#16110);
#13605=AXIS2_PLACEMENT_3D('',#37694,#16111,#16112);
#13606=AXIS2_PLACEMENT_3D('',#37695,#16113,#16114);
#13607=AXIS2_PLACEMENT_3D('',#37696,#16115,#16116);
#13608=AXIS2_PLACEMENT_3D('',#37697,#16117,#16118);
#13609=AXIS2_PLACEMENT_3D('',#37698,#16119,#16120);
#13610=AXIS2_PLACEMENT_3D('',#37699,#16121,#16122);
#13611=AXIS2_PLACEMENT_3D('',#37700,#16123,#16124);
#13612=AXIS2_PLACEMENT_3D('',#37701,#16125,#16126);
#13613=AXIS2_PLACEMENT_3D('',#37703,#16128,#16129);
#13614=AXIS2_PLACEMENT_3D('',#37704,#16130,#16131);
#13615=AXIS2_PLACEMENT_3D('',#37705,#16132,#16133);
#13616=AXIS2_PLACEMENT_3D('',#37706,#16134,#16135);
#13617=AXIS2_PLACEMENT_3D('',#37707,#16136,#16137);
#13618=AXIS2_PLACEMENT_3D('',#37708,#16138,#16139);
#13619=AXIS2_PLACEMENT_3D('',#37709,#16140,#16141);
#13620=AXIS2_PLACEMENT_3D('',#37710,#16142,#16143);
#13621=AXIS2_PLACEMENT_3D('',#37711,#16144,#16145);
#13622=AXIS2_PLACEMENT_3D('',#37713,#16147,#16148);
#13623=AXIS2_PLACEMENT_3D('',#37715,#16150,#16151);
#13624=AXIS2_PLACEMENT_3D('',#37718,#16154,#16155);
#13625=AXIS2_PLACEMENT_3D('',#37871,#16158,#16159);
#13626=AXIS2_PLACEMENT_3D('',#38023,#16161,#16162);
#15739=DIRECTION('axis',(0.,0.,1.));
#15740=DIRECTION('refdir',(1.,0.,0.));
#15741=DIRECTION('center_axis',(0.,9.02056207507939E-16,-1.));
#15742=DIRECTION('ref_axis',(1.,0.,0.));
#15743=DIRECTION('center_axis',(0.,8.7430063189231E-16,-1.));
#15744=DIRECTION('ref_axis',(1.,0.,0.));
#15745=DIRECTION('',(0.,-9.02056207507939E-16,1.));
#15746=DIRECTION('center_axis',(0.,8.7430063189231E-16,-1.));
#15747=DIRECTION('ref_axis',(1.,0.,0.));
#15748=DIRECTION('center_axis',(0.,9.02056207507939E-16,-1.));
#15749=DIRECTION('ref_axis',(1.,0.,0.));
#15750=DIRECTION('center_axis',(0.,8.7430063189231E-16,-1.));
#15751=DIRECTION('ref_axis',(1.,0.,0.));
#15752=DIRECTION('',(0.,-9.02056207507939E-16,1.));
#15753=DIRECTION('center_axis',(0.,-8.7430063189231E-16,1.));
#15754=DIRECTION('ref_axis',(1.,0.,0.));
#15755=DIRECTION('center_axis',(0.,8.7430063189231E-16,-1.));
#15756=DIRECTION('ref_axis',(1.,0.,0.));
#15757=DIRECTION('center_axis',(0.,8.7430063189231E-16,-1.));
#15758=DIRECTION('ref_axis',(1.,0.,0.));
#15759=DIRECTION('center_axis',(0.,0.,-1.));
#15760=DIRECTION('ref_axis',(-0.936029699362847,-0.351921016579996,0.));
#15761=DIRECTION('center_axis',(0.,0.,1.));
#15762=DIRECTION('ref_axis',(-0.936029699362847,-0.351921016579996,0.));
#15763=DIRECTION('',(0.,0.,-1.));
#15764=DIRECTION('center_axis',(0.,0.,-1.));
#15765=DIRECTION('ref_axis',(-0.936029699362847,-0.351921016579996,0.));
#15766=DIRECTION('',(0.,0.,1.));
#15767=DIRECTION('center_axis',(0.440660664196194,0.897673759798163,0.));
#15768=DIRECTION('ref_axis',(-0.897673759798163,0.440660664196194,0.));
#15769=DIRECTION('',(-0.897673759798163,0.440660664196194,0.));
#15770=DIRECTION('',(0.,0.,1.));
#15771=DIRECTION('',(0.897673759798163,-0.440660664196194,0.));
#15772=DIRECTION('center_axis',(0.,0.,1.));
#15773=DIRECTION('ref_axis',(0.0454476916968278,0.998966719825756,0.));
#15774=DIRECTION('center_axis',(0.,0.,-1.));
#15775=DIRECTION('ref_axis',(0.0454476916968278,0.998966719825756,0.));
#15776=DIRECTION('',(0.,0.,1.));
#15777=DIRECTION('center_axis',(0.,0.,1.));
#15778=DIRECTION('ref_axis',(0.0454476916968278,0.998966719825756,0.));
#15779=DIRECTION('',(0.,0.,-1.));
#15780=DIRECTION('center_axis',(-0.717566844774038,-0.696489643340827,0.));
#15781=DIRECTION('ref_axis',(0.696489643340827,-0.717566844774038,0.));
#15782=DIRECTION('',(0.696489643340827,-0.717566844774038,0.));
#15783=DIRECTION('',(0.,0.,1.));
#15784=DIRECTION('',(0.696489643340827,-0.717566844774038,0.));
#15785=DIRECTION('center_axis',(0.,0.,-1.));
#15786=DIRECTION('ref_axis',(-0.964117917541714,0.265474369902311,0.));
#15787=DIRECTION('center_axis',(0.,0.,1.));
#15788=DIRECTION('ref_axis',(-0.964117917541714,0.265474369902311,0.));
#15789=DIRECTION('',(0.,0.,-1.));
#15790=DIRECTION('center_axis',(0.,0.,-1.));
#15791=DIRECTION('ref_axis',(-0.964117917541714,0.265474369902311,0.));
#15792=DIRECTION('',(0.,0.,1.));
#15793=DIRECTION('center_axis',(0.884141363466569,0.46721948740124,0.));
#15794=DIRECTION('ref_axis',(-0.46721948740124,0.884141363466569,0.));
#15795=DIRECTION('',(-0.46721948740124,0.884141363466569,0.));
#15796=DIRECTION('',(0.,0.,1.));
#15797=DIRECTION('',(0.46721948740124,-0.884141363466569,0.));
#15798=DIRECTION('center_axis',(0.,0.,1.));
#15799=DIRECTION('ref_axis',(0.623945860382415,0.781467570223901,0.));
#15800=DIRECTION('center_axis',(0.,0.,-1.));
#15801=DIRECTION('ref_axis',(0.623945860382415,0.781467570223901,0.));
#15802=DIRECTION('',(0.,0.,1.));
#15803=DIRECTION('center_axis',(0.,0.,1.));
#15804=DIRECTION('ref_axis',(0.623945860382415,0.781467570223901,0.));
#15805=DIRECTION('',(0.,0.,-1.));
#15806=DIRECTION('center_axis',(-0.989910112752389,-0.141696748976653,0.));
#15807=DIRECTION('ref_axis',(0.141696748976653,-0.989910112752389,0.));
#15808=DIRECTION('',(0.141696748976653,-0.989910112752389,0.));
#15809=DIRECTION('',(0.,0.,1.));
#15810=DIRECTION('',(0.141696748976653,-0.989910112752389,0.));
#15811=DIRECTION('center_axis',(0.,0.,-1.));
#15812=DIRECTION('ref_axis',(-0.623945860382415,0.781467570223901,0.));
#15813=DIRECTION('center_axis',(0.,0.,1.));
#15814=DIRECTION('ref_axis',(-0.623945860382415,0.781467570223901,0.));
#15815=DIRECTION('',(0.,0.,-1.));
#15816=DIRECTION('center_axis',(0.,0.,-1.));
#15817=DIRECTION('ref_axis',(-0.623945860382415,0.781467570223901,0.));
#15818=DIRECTION('',(0.,0.,1.));
#15819=DIRECTION('center_axis',(0.989910112752389,-0.141696748976654,0.));
#15820=DIRECTION('ref_axis',(0.141696748976654,0.989910112752389,0.));
#15821=DIRECTION('',(0.141696748976654,0.989910112752389,0.));
#15822=DIRECTION('',(0.,0.,1.));
#15823=DIRECTION('',(-0.141696748976654,-0.989910112752389,0.));
#15824=DIRECTION('center_axis',(0.,0.,1.));
#15825=DIRECTION('ref_axis',(0.964117917541713,0.265474369902315,0.));
#15826=DIRECTION('center_axis',(0.,0.,-1.));
#15827=DIRECTION('ref_axis',(0.964117917541713,0.265474369902315,0.));
#15828=DIRECTION('',(0.,0.,1.));
#15829=DIRECTION('center_axis',(0.,0.,1.));
#15830=DIRECTION('ref_axis',(0.964117917541713,0.265474369902315,0.));
#15831=DIRECTION('',(0.,0.,-1.));
#15832=DIRECTION('center_axis',(-0.884141363466568,0.46721948740124,0.));
#15833=DIRECTION('ref_axis',(-0.46721948740124,-0.884141363466568,0.));
#15834=DIRECTION('',(-0.46721948740124,-0.884141363466568,0.));
#15835=DIRECTION('',(0.,0.,1.));
#15836=DIRECTION('',(-0.46721948740124,-0.884141363466568,0.));
#15837=DIRECTION('center_axis',(0.,0.,-1.));
#15838=DIRECTION('ref_axis',(-0.0454476916968278,0.998966719825756,0.));
#15839=DIRECTION('center_axis',(0.,0.,1.));
#15840=DIRECTION('ref_axis',(-0.0454476916968278,0.998966719825756,0.));
#15841=DIRECTION('',(0.,0.,-1.));
#15842=DIRECTION('center_axis',(0.,0.,-1.));
#15843=DIRECTION('ref_axis',(-0.0454476916968278,0.998966719825756,0.));
#15844=DIRECTION('',(0.,0.,1.));
#15845=DIRECTION('center_axis',(0.717566844774037,-0.696489643340827,0.));
#15846=DIRECTION('ref_axis',(0.696489643340827,0.717566844774037,0.));
#15847=DIRECTION('',(0.696489643340827,0.717566844774037,0.));
#15848=DIRECTION('',(0.,0.,1.));
#15849=DIRECTION('',(-0.696489643340827,-0.717566844774037,0.));
#15850=DIRECTION('center_axis',(0.,0.,1.));
#15851=DIRECTION('ref_axis',(0.936029699362847,-0.351921016579998,0.));
#15852=DIRECTION('center_axis',(0.,0.,-1.));
#15853=DIRECTION('ref_axis',(0.936029699362847,-0.351921016579998,0.));
#15854=DIRECTION('',(0.,0.,1.));
#15855=DIRECTION('center_axis',(0.,0.,1.));
#15856=DIRECTION('ref_axis',(0.936029699362847,-0.351921016579998,0.));
#15857=DIRECTION('',(0.,0.,-1.));
#15858=DIRECTION('center_axis',(-0.440660664196193,0.897673759798163,0.));
#15859=DIRECTION('ref_axis',(-0.897673759798163,-0.440660664196193,0.));
#15860=DIRECTION('',(-0.897673759798163,-0.440660664196193,0.));
#15861=DIRECTION('',(0.,0.,1.));
#15862=DIRECTION('',(-0.897673759798163,-0.440660664196193,0.));
#15863=DIRECTION('center_axis',(0.,0.,-1.));
#15864=DIRECTION('ref_axis',(0.550409950506719,0.834894536084164,0.));
#15865=DIRECTION('center_axis',(0.,0.,1.));
#15866=DIRECTION('ref_axis',(0.550409950506719,0.834894536084164,0.));
#15867=DIRECTION('',(0.,0.,-1.));
#15868=DIRECTION('center_axis',(0.,0.,-1.));
#15869=DIRECTION('ref_axis',(0.550409950506719,0.834894536084164,0.));
#15870=DIRECTION('',(0.,0.,1.));
#15871=DIRECTION('center_axis',(0.171137431292023,-0.985247166761097,0.));
#15872=DIRECTION('ref_axis',(0.985247166761097,0.171137431292023,0.));
#15873=DIRECTION('',(0.985247166761096,0.171137431292023,0.));
#15874=DIRECTION('',(0.,0.,1.));
#15875=DIRECTION('',(-0.985247166761096,-0.171137431292023,0.));
#15876=DIRECTION('center_axis',(0.,0.,1.));
#15877=DIRECTION('ref_axis',(0.550409950506721,-0.834894536084163,0.));
#15878=DIRECTION('center_axis',(0.,0.,-1.));
#15879=DIRECTION('ref_axis',(0.550409950506721,-0.834894536084163,0.));
#15880=DIRECTION('',(0.,0.,1.));
#15881=DIRECTION('center_axis',(0.,0.,1.));
#15882=DIRECTION('ref_axis',(0.550409950506721,-0.834894536084163,0.));
#15883=DIRECTION('',(0.,0.,-1.));
#15884=DIRECTION('center_axis',(0.171137431292024,0.985247166761096,0.));
#15885=DIRECTION('ref_axis',(-0.985247166761096,0.171137431292024,0.));
#15886=DIRECTION('',(-0.985247166761096,0.171137431292024,0.));
#15887=DIRECTION('',(0.,0.,1.));
#15888=DIRECTION('',(-0.985247166761096,0.171137431292024,0.));
#15889=DIRECTION('center_axis',(0.,0.,-1.));
#15890=DIRECTION('ref_axis',(0.936029699362847,0.351921016579996,0.));
#15891=DIRECTION('center_axis',(0.,0.,1.));
#15892=DIRECTION('ref_axis',(0.936029699362847,0.351921016579996,0.));
#15893=DIRECTION('',(0.,0.,-1.));
#15894=DIRECTION('center_axis',(0.,0.,-1.));
#15895=DIRECTION('ref_axis',(0.936029699362847,0.351921016579996,0.));
#15896=DIRECTION('',(0.,0.,1.));
#15897=DIRECTION('center_axis',(-0.440660664196194,-0.897673759798163,0.));
#15898=DIRECTION('ref_axis',(0.897673759798163,-0.440660664196194,0.));
#15899=DIRECTION('',(0.897673759798163,-0.440660664196194,0.));
#15900=DIRECTION('',(0.,0.,1.));
#15901=DIRECTION('',(-0.897673759798163,0.440660664196194,0.));
#15902=DIRECTION('center_axis',(0.,0.,1.));
#15903=DIRECTION('ref_axis',(-0.0454476916968339,-0.998966719825755,0.));
#15904=DIRECTION('center_axis',(0.,0.,-1.));
#15905=DIRECTION('ref_axis',(-0.0454476916968339,-0.998966719825755,0.));
#15906=DIRECTION('',(0.,0.,1.));
#15907=DIRECTION('center_axis',(0.,0.,1.));
#15908=DIRECTION('ref_axis',(-0.0454476916968339,-0.998966719825755,0.));
#15909=DIRECTION('',(0.,0.,-1.));
#15910=DIRECTION('center_axis',(0.717566844774038,0.696489643340827,0.));
#15911=DIRECTION('ref_axis',(-0.696489643340827,0.717566844774038,0.));
#15912=DIRECTION('',(-0.696489643340827,0.717566844774038,0.));
#15913=DIRECTION('',(0.,0.,1.));
#15914=DIRECTION('',(-0.696489643340827,0.717566844774038,0.));
#15915=DIRECTION('center_axis',(0.,0.,-1.));
#15916=DIRECTION('ref_axis',(0.964117917541713,-0.265474369902315,0.));
#15917=DIRECTION('center_axis',(0.,0.,1.));
#15918=DIRECTION('ref_axis',(0.964117917541713,-0.265474369902315,0.));
#15919=DIRECTION('',(0.,0.,-1.));
#15920=DIRECTION('center_axis',(0.,0.,-1.));
#15921=DIRECTION('ref_axis',(0.964117917541713,-0.265474369902315,0.));
#15922=DIRECTION('',(0.,0.,1.));
#15923=DIRECTION('center_axis',(-0.884141363466569,-0.46721948740124,0.));
#15924=DIRECTION('ref_axis',(0.46721948740124,-0.884141363466569,0.));
#15925=DIRECTION('',(0.46721948740124,-0.884141363466568,0.));
#15926=DIRECTION('',(0.,0.,1.));
#15927=DIRECTION('',(-0.46721948740124,0.884141363466568,0.));
#15928=DIRECTION('center_axis',(0.,0.,1.));
#15929=DIRECTION('ref_axis',(-0.623945860382415,-0.781467570223901,0.));
#15930=DIRECTION('center_axis',(0.,0.,-1.));
#15931=DIRECTION('ref_axis',(-0.623945860382415,-0.781467570223901,0.));
#15932=DIRECTION('',(0.,0.,1.));
#15933=DIRECTION('center_axis',(0.,0.,1.));
#15934=DIRECTION('ref_axis',(-0.623945860382415,-0.781467570223901,0.));
#15935=DIRECTION('',(0.,0.,-1.));
#15936=DIRECTION('center_axis',(0.989910112752389,0.141696748976653,0.));
#15937=DIRECTION('ref_axis',(-0.141696748976653,0.989910112752389,0.));
#15938=DIRECTION('',(-0.141696748976653,0.989910112752389,0.));
#15939=DIRECTION('',(0.,0.,1.));
#15940=DIRECTION('',(-0.141696748976653,0.989910112752389,0.));
#15941=DIRECTION('center_axis',(0.,0.,-1.));
#15942=DIRECTION('ref_axis',(0.623945860382414,-0.781467570223902,0.));
#15943=DIRECTION('center_axis',(0.,0.,1.));
#15944=DIRECTION('ref_axis',(0.623945860382414,-0.781467570223902,0.));
#15945=DIRECTION('',(0.,0.,-1.));
#15946=DIRECTION('center_axis',(0.,0.,-1.));
#15947=DIRECTION('ref_axis',(0.623945860382414,-0.781467570223902,0.));
#15948=DIRECTION('',(0.,0.,1.));
#15949=DIRECTION('center_axis',(-0.989910112752389,0.141696748976654,0.));
#15950=DIRECTION('ref_axis',(-0.141696748976654,-0.989910112752389,0.));
#15951=DIRECTION('',(-0.141696748976654,-0.989910112752389,0.));
#15952=DIRECTION('',(0.,0.,1.));
#15953=DIRECTION('',(0.141696748976654,0.989910112752389,0.));
#15954=DIRECTION('center_axis',(0.,0.,1.));
#15955=DIRECTION('ref_axis',(-0.964117917541714,-0.265474369902312,0.));
#15956=DIRECTION('center_axis',(0.,0.,-1.));
#15957=DIRECTION('ref_axis',(-0.964117917541714,-0.265474369902312,0.));
#15958=DIRECTION('',(0.,0.,1.));
#15959=DIRECTION('center_axis',(0.,0.,1.));
#15960=DIRECTION('ref_axis',(-0.964117917541714,-0.265474369902312,0.));
#15961=DIRECTION('',(0.,0.,-1.));
#15962=DIRECTION('center_axis',(0.884141363466569,-0.46721948740124,0.));
#15963=DIRECTION('ref_axis',(0.46721948740124,0.884141363466569,0.));
#15964=DIRECTION('',(0.46721948740124,0.884141363466568,0.));
#15965=DIRECTION('',(0.,0.,1.));
#15966=DIRECTION('',(0.46721948740124,0.884141363466568,0.));
#15967=DIRECTION('center_axis',(0.,0.,-1.));
#15968=DIRECTION('ref_axis',(0.0454476916968278,-0.998966719825756,0.));
#15969=DIRECTION('center_axis',(0.,0.,1.));
#15970=DIRECTION('ref_axis',(0.0454476916968278,-0.998966719825756,0.));
#15971=DIRECTION('',(0.,0.,-1.));
#15972=DIRECTION('center_axis',(0.,0.,-1.));
#15973=DIRECTION('ref_axis',(0.0454476916968278,-0.998966719825756,0.));
#15974=DIRECTION('',(0.,0.,1.));
#15975=DIRECTION('center_axis',(-0.717566844774037,0.696489643340827,0.));
#15976=DIRECTION('ref_axis',(-0.696489643340827,-0.717566844774037,0.));
#15977=DIRECTION('',(-0.696489643340827,-0.717566844774037,0.));
#15978=DIRECTION('',(0.,0.,1.));
#15979=DIRECTION('',(0.696489643340827,0.717566844774037,0.));
#15980=DIRECTION('center_axis',(0.,0.,1.));
#15981=DIRECTION('ref_axis',(-0.936029699362846,0.351921016579999,0.));
#15982=DIRECTION('center_axis',(0.,0.,-1.));
#15983=DIRECTION('ref_axis',(-0.936029699362846,0.351921016579999,0.));
#15984=DIRECTION('',(0.,0.,1.));
#15985=DIRECTION('center_axis',(0.,0.,1.));
#15986=DIRECTION('ref_axis',(-0.936029699362846,0.351921016579999,0.));
#15987=DIRECTION('',(0.,0.,-1.));
#15988=DIRECTION('center_axis',(0.440660664196194,-0.897673759798163,0.));
#15989=DIRECTION('ref_axis',(0.897673759798163,0.440660664196194,0.));
#15990=DIRECTION('',(0.897673759798163,0.440660664196194,0.));
#15991=DIRECTION('',(0.,0.,1.));
#15992=DIRECTION('',(0.897673759798163,0.440660664196194,0.));
#15993=DIRECTION('',(0.,0.,1.));
#15994=DIRECTION('center_axis',(0.,0.,1.));
#15995=DIRECTION('ref_axis',(0.779271010009485,-0.62668707738296,0.));
#15996=DIRECTION('center_axis',(0.,0.,1.));
#15997=DIRECTION('ref_axis',(0.779271010009485,-0.62668707738296,0.));
#15998=DIRECTION('center_axis',(0.,0.,1.));
#15999=DIRECTION('ref_axis',(0.779271010009485,-0.62668707738296,0.));
#16000=DIRECTION('',(0.,0.,1.));
#16001=DIRECTION('',(0.,0.,1.));
#16002=DIRECTION('center_axis',(0.,0.,1.));
#16003=DIRECTION('ref_axis',(0.262086068433427,-0.965044502980618,0.));
#16004=DIRECTION('center_axis',(0.,0.,1.));
#16005=DIRECTION('ref_axis',(0.262086068433427,-0.965044502980618,0.));
#16006=DIRECTION('center_axis',(0.,0.,1.));
#16007=DIRECTION('ref_axis',(0.262086068433427,-0.965044502980618,0.));
#16008=DIRECTION('',(0.,0.,1.));
#16009=DIRECTION('',(0.,0.,1.));
#16010=DIRECTION('center_axis',(0.,0.,1.));
#16011=DIRECTION('ref_axis',(-0.355206843306369,-0.934787729095929,0.));
#16012=DIRECTION('center_axis',(0.,0.,1.));
#16013=DIRECTION('ref_axis',(-0.355206843306369,-0.934787729095929,0.));
#16014=DIRECTION('center_axis',(0.,0.,1.));
#16015=DIRECTION('ref_axis',(-0.355206843306369,-0.934787729095929,0.));
#16016=DIRECTION('',(0.,0.,1.));
#16017=DIRECTION('',(0.,0.,1.));
#16018=DIRECTION('center_axis',(0.,0.,1.));
#16019=DIRECTION('ref_axis',(-0.83682281393969,-0.547473814962924,0.));
#16020=DIRECTION('center_axis',(0.,0.,1.));
#16021=DIRECTION('ref_axis',(-0.83682281393969,-0.547473814962924,0.));
#16022=DIRECTION('center_axis',(0.,0.,1.));
#16023=DIRECTION('ref_axis',(-0.83682281393969,-0.547473814962924,0.));
#16024=DIRECTION('',(0.,0.,1.));
#16025=DIRECTION('',(0.,0.,1.));
#16026=DIRECTION('center_axis',(0.,0.,1.));
#16027=DIRECTION('ref_axis',(-0.998800912209379,0.048956488535347,0.));
#16028=DIRECTION('center_axis',(0.,0.,1.));
#16029=DIRECTION('ref_axis',(-0.998800912209379,0.048956488535347,0.));
#16030=DIRECTION('center_axis',(0.,0.,1.));
#16031=DIRECTION('ref_axis',(-0.998800912209379,0.048956488535347,0.));
#16032=DIRECTION('',(0.,0.,1.));
#16033=DIRECTION('',(0.,0.,1.));
#16034=DIRECTION('center_axis',(0.,0.,1.));
#16035=DIRECTION('ref_axis',(-0.779271010009485,0.62668707738296,0.));
#16036=DIRECTION('center_axis',(0.,0.,1.));
#16037=DIRECTION('ref_axis',(-0.779271010009485,0.62668707738296,0.));
#16038=DIRECTION('center_axis',(0.,0.,1.));
#16039=DIRECTION('ref_axis',(-0.779271010009485,0.62668707738296,0.));
#16040=DIRECTION('',(0.,0.,1.));
#16041=DIRECTION('',(0.,0.,1.));
#16042=DIRECTION('center_axis',(0.,0.,1.));
#16043=DIRECTION('ref_axis',(-0.262086068433428,0.965044502980618,0.));
#16044=DIRECTION('center_axis',(0.,0.,1.));
#16045=DIRECTION('ref_axis',(-0.262086068433428,0.965044502980618,0.));
#16046=DIRECTION('center_axis',(0.,0.,1.));
#16047=DIRECTION('ref_axis',(-0.262086068433428,0.965044502980618,0.));
#16048=DIRECTION('',(0.,0.,1.));
#16049=DIRECTION('',(0.,0.,1.));
#16050=DIRECTION('center_axis',(0.,0.,1.));
#16051=DIRECTION('ref_axis',(0.355206843306369,0.934787729095929,0.));
#16052=DIRECTION('center_axis',(0.,0.,1.));
#16053=DIRECTION('ref_axis',(0.355206843306369,0.934787729095929,0.));
#16054=DIRECTION('center_axis',(0.,0.,1.));
#16055=DIRECTION('ref_axis',(0.355206843306369,0.934787729095929,0.));
#16056=DIRECTION('',(0.,0.,1.));
#16057=DIRECTION('',(0.,0.,1.));
#16058=DIRECTION('center_axis',(0.,0.,1.));
#16059=DIRECTION('ref_axis',(0.83682281393969,0.547473814962924,0.));
#16060=DIRECTION('center_axis',(0.,0.,1.));
#16061=DIRECTION('ref_axis',(0.83682281393969,0.547473814962924,0.));
#16062=DIRECTION('center_axis',(0.,0.,1.));
#16063=DIRECTION('ref_axis',(0.83682281393969,0.547473814962924,0.));
#16064=DIRECTION('',(0.,0.,1.));
#16065=DIRECTION('center_axis',(0.,0.,1.));
#16066=DIRECTION('ref_axis',(1.,0.,0.));
#16067=DIRECTION('center_axis',(0.,0.,1.));
#16068=DIRECTION('ref_axis',(1.,0.,0.));
#16069=DIRECTION('center_axis',(0.,0.,1.));
#16070=DIRECTION('ref_axis',(1.,0.,0.));
#16071=DIRECTION('center_axis',(0.,0.,1.));
#16072=DIRECTION('ref_axis',(1.,0.,0.));
#16073=DIRECTION('center_axis',(0.,0.,1.));
#16074=DIRECTION('ref_axis',(1.,0.,0.));
#16075=DIRECTION('center_axis',(0.,0.,1.));
#16076=DIRECTION('ref_axis',(1.,0.,0.));
#16077=DIRECTION('center_axis',(0.,0.,1.));
#16078=DIRECTION('ref_axis',(1.,0.,0.));
#16079=DIRECTION('center_axis',(0.,0.,1.));
#16080=DIRECTION('ref_axis',(1.,0.,0.));
#16081=DIRECTION('center_axis',(0.,0.,1.));
#16082=DIRECTION('ref_axis',(1.,0.,0.));
#16083=DIRECTION('center_axis',(0.,0.,-1.));
#16084=DIRECTION('ref_axis',(-0.55040995050672,-0.834894536084163,0.));
#16085=DIRECTION('',(0.985247166761096,0.171137431292024,0.));
#16086=DIRECTION('center_axis',(0.,0.,1.));
#16087=DIRECTION('ref_axis',(0.998800912209379,-0.0489564885353468,0.));
#16088=DIRECTION('',(0.985247166761096,-0.171137431292024,0.));
#16089=DIRECTION('center_axis',(0.,0.,-1.));
#16090=DIRECTION('ref_axis',(-0.55040995050672,0.834894536084163,0.));
#16091=DIRECTION('center_axis',(0.,0.,1.));
#16092=DIRECTION('ref_axis',(1.,0.,0.));
#16093=DIRECTION('center_axis',(0.,0.,1.));
#16094=DIRECTION('ref_axis',(1.,0.,0.));
#16095=DIRECTION('center_axis',(0.,0.,1.));
#16096=DIRECTION('ref_axis',(1.,0.,0.));
#16097=DIRECTION('center_axis',(0.,0.,1.));
#16098=DIRECTION('ref_axis',(1.,0.,0.));
#16099=DIRECTION('center_axis',(0.,0.,1.));
#16100=DIRECTION('ref_axis',(-0.55040995050672,0.834894536084163,0.));
#16101=DIRECTION('',(0.985247166761096,-0.171137431292024,0.));
#16102=DIRECTION('center_axis',(0.,0.,1.));
#16103=DIRECTION('ref_axis',(0.998800912209379,-0.0489564885353468,0.));
#16104=DIRECTION('',(-0.985247166761096,-0.171137431292024,0.));
#16105=DIRECTION('center_axis',(0.,0.,1.));
#16106=DIRECTION('ref_axis',(-0.55040995050672,-0.834894536084163,0.));
#16107=DIRECTION('center_axis',(0.,0.,1.));
#16108=DIRECTION('ref_axis',(1.,0.,0.));
#16109=DIRECTION('center_axis',(0.,0.,1.));
#16110=DIRECTION('ref_axis',(1.,0.,0.));
#16111=DIRECTION('center_axis',(0.,0.,1.));
#16112=DIRECTION('ref_axis',(1.,0.,0.));
#16113=DIRECTION('center_axis',(0.,0.,1.));
#16114=DIRECTION('ref_axis',(1.,0.,0.));
#16115=DIRECTION('center_axis',(0.,0.,1.));
#16116=DIRECTION('ref_axis',(1.,0.,0.));
#16117=DIRECTION('center_axis',(0.,0.,1.));
#16118=DIRECTION('ref_axis',(1.,0.,0.));
#16119=DIRECTION('center_axis',(0.,0.,1.));
#16120=DIRECTION('ref_axis',(1.,0.,0.));
#16121=DIRECTION('center_axis',(0.,0.,1.));
#16122=DIRECTION('ref_axis',(1.,0.,0.));
#16123=DIRECTION('center_axis',(0.,0.,1.));
#16124=DIRECTION('ref_axis',(1.,0.,0.));
#16125=DIRECTION('center_axis',(0.,0.,1.));
#16126=DIRECTION('ref_axis',(1.,0.,0.));
#16127=DIRECTION('',(0.,0.,1.));
#16128=DIRECTION('center_axis',(0.,0.,1.));
#16129=DIRECTION('ref_axis',(1.,0.,0.));
#16130=DIRECTION('center_axis',(0.,0.,1.));
#16131=DIRECTION('ref_axis',(1.,0.,0.));
#16132=DIRECTION('center_axis',(0.,0.,1.));
#16133=DIRECTION('ref_axis',(1.,0.,0.));
#16134=DIRECTION('center_axis',(0.,0.,1.));
#16135=DIRECTION('ref_axis',(1.,0.,0.));
#16136=DIRECTION('center_axis',(0.,0.,1.));
#16137=DIRECTION('ref_axis',(1.,0.,0.));
#16138=DIRECTION('center_axis',(0.,0.,1.));
#16139=DIRECTION('ref_axis',(1.,0.,0.));
#16140=DIRECTION('center_axis',(0.,0.,1.));
#16141=DIRECTION('ref_axis',(1.,0.,0.));
#16142=DIRECTION('center_axis',(0.,0.,1.));
#16143=DIRECTION('ref_axis',(1.,0.,0.));
#16144=DIRECTION('center_axis',(0.,0.,-1.));
#16145=DIRECTION('ref_axis',(-0.55040995050672,-0.834894536084163,0.));
#16146=DIRECTION('',(0.,0.,-1.));
#16147=DIRECTION('center_axis',(-0.171137431292024,0.985247166761097,0.));
#16148=DIRECTION('ref_axis',(-0.985247166761096,-0.171137431292024,0.));
#16149=DIRECTION('',(0.,0.,1.));
#16150=DIRECTION('center_axis',(0.,0.,1.));
#16151=DIRECTION('ref_axis',(-0.55040995050672,0.834894536084163,0.));
#16152=DIRECTION('',(0.,0.,1.));
#16153=DIRECTION('',(0.,0.,-1.));
#16154=DIRECTION('center_axis',(-0.171137431292024,-0.985247166761097,0.));
#16155=DIRECTION('ref_axis',(0.985247166761096,-0.171137431292024,0.));
#16156=DIRECTION('',(0.,0.,1.));
#16157=DIRECTION('',(0.,0.,1.));
#16158=DIRECTION('center_axis',(0.,0.,1.));
#16159=DIRECTION('ref_axis',(0.998800912209379,-0.0489564885353468,0.));
#16160=DIRECTION('',(0.,0.,1.));
#16161=DIRECTION('center_axis',(0.,0.,1.));
#16162=DIRECTION('ref_axis',(1.,0.,0.));
#31617=CARTESIAN_POINT('',(0.,0.,0.));
#31618=CARTESIAN_POINT('Origin',(3.70814490224802E-12,-1.04805053524615E-12,
7.49999782838924));
#31619=CARTESIAN_POINT('',(-7.49999999999629,-1.12798659301916E-12,14.9999978283892));
#31620=CARTESIAN_POINT('Origin',(3.70814490224802E-12,-1.12798659301916E-12,
14.9999978283892));
#31621=CARTESIAN_POINT('',(-7.4999999999963,-1.09223486052218E-12,57.4999978283893));
#31622=CARTESIAN_POINT('',(-7.4999999999963,-1.04713205014679E-12,7.49999782838924));
#31623=CARTESIAN_POINT('Origin',(3.70814490224802E-12,-1.09315334562154E-12,
57.4999978283893));
#31624=CARTESIAN_POINT('Origin',(3.70814490224802E-12,-1.04805053524615E-12,
7.49999782838924));
#31625=CARTESIAN_POINT('',(-7.4999999999963,-1.00112718356388E-12,-43.5000021716108));
#31626=CARTESIAN_POINT('Origin',(3.70814490224802E-12,-1.00204566866324E-12,
-43.5000021716108));
#31627=CARTESIAN_POINT('',(-7.49999999999629,-1.11022302462516E-12,-2.17161075816152E-6));
#31628=CARTESIAN_POINT('',(-7.4999999999963,-1.04713205014679E-12,7.49999782838924));
#31629=CARTESIAN_POINT('Origin',(3.70814490224802E-12,-1.11022302462516E-12,
-2.17161075816152E-6));
#31630=CARTESIAN_POINT('Origin',(3.70814490224802E-12,-1.09232067835308E-12,
57.4999978283893));
#31631=CARTESIAN_POINT('Origin',(3.70814490224802E-12,-1.00290609150733E-12,
-43.5000021716108));
#31632=CARTESIAN_POINT('Origin',(15.1099349338646,-6.30335230606528,0.));
#31633=CARTESIAN_POINT('',(14.1870217324314,-5.91834422482504,15.));
#31634=CARTESIAN_POINT('',(14.6692742696684,-7.20102606586345,15.));
#31635=CARTESIAN_POINT('Origin',(15.1099349338646,-6.30335230606528,15.));
#31636=CARTESIAN_POINT('',(14.6692742696684,-7.20102606586345,0.));
#31637=CARTESIAN_POINT('',(14.6692742696684,-7.20102606586345,0.));
#31638=CARTESIAN_POINT('',(14.1870217324314,-5.91834422482504,0.));
#31639=CARTESIAN_POINT('Origin',(15.1099349338646,-6.30335230606528,0.));
#31640=CARTESIAN_POINT('',(14.1870217324314,-5.91834422482504,0.));
#31641=CARTESIAN_POINT('Origin',(16.8707481591095,-8.28171148831561,0.));
#31642=CARTESIAN_POINT('',(16.8707481591095,-8.28171148831561,15.));
#31643=CARTESIAN_POINT('',(13.7900642980194,-6.76942912338193,15.));
#31644=CARTESIAN_POINT('',(16.8707481591095,-8.28171148831561,0.));
#31645=CARTESIAN_POINT('',(16.8707481591095,-8.28171148831561,0.));
#31646=CARTESIAN_POINT('',(13.7900642980194,-6.76942912338193,0.));
#31647=CARTESIAN_POINT('Origin',(10.6640709636513,-12.422559095541,0.));
#31648=CARTESIAN_POINT('',(10.0127106555856,-11.6637905214181,0.));
#31649=CARTESIAN_POINT('',(11.3816378084254,-11.7260694522002,0.));
#31650=CARTESIAN_POINT('Origin',(10.6640709636513,-12.422559095541,0.));
#31651=CARTESIAN_POINT('',(11.3816378084254,-11.7260694522002,15.));
#31652=CARTESIAN_POINT('',(11.3816378084254,-11.7260694522002,0.));
#31653=CARTESIAN_POINT('',(10.0127106555856,-11.6637905214181,15.));
#31654=CARTESIAN_POINT('Origin',(10.6640709636513,-12.422559095541,15.));
#31655=CARTESIAN_POINT('',(10.0127106555856,-11.6637905214181,0.));
#31656=CARTESIAN_POINT('Origin',(10.6994739010018,-11.0232618694188,0.));
#31657=CARTESIAN_POINT('',(13.0897235660237,-13.4858453790958,0.));
#31658=CARTESIAN_POINT('',(10.6994739010018,-11.0232618694188,0.));
#31659=CARTESIAN_POINT('',(13.0897235660237,-13.4858453790958,15.));
#31660=CARTESIAN_POINT('',(13.0897235660237,-13.4858453790958,0.));
#31661=CARTESIAN_POINT('',(10.6994739010018,-11.0232618694188,15.));
#31662=CARTESIAN_POINT('Origin',(8.51917661988723,-13.9809160543638,0.));
#31663=CARTESIAN_POINT('',(7.9988262277612,-13.1269632047203,15.));
#31664=CARTESIAN_POINT('',(7.63503525642066,-14.448135541765,15.));
#31665=CARTESIAN_POINT('Origin',(8.51917661988723,-13.9809160543638,15.));
#31666=CARTESIAN_POINT('',(7.63503525642066,-14.448135541765,0.));
#31667=CARTESIAN_POINT('',(7.63503525642066,-14.448135541765,0.));
#31668=CARTESIAN_POINT('',(7.9988262277612,-13.1269632047203,0.));
#31669=CARTESIAN_POINT('Origin',(8.51917661988723,-13.9809160543638,0.));
#31670=CARTESIAN_POINT('',(7.9988262277612,-13.1269632047203,0.));
#31671=CARTESIAN_POINT('Origin',(8.78085409196639,-16.6164222996225,0.));
#31672=CARTESIAN_POINT('',(8.78085409196639,-16.6164222996225,15.));
#31673=CARTESIAN_POINT('',(7.17742576545784,-13.5821796255734,15.));
#31674=CARTESIAN_POINT('',(8.78085409196639,-16.6164222996225,0.));
#31675=CARTESIAN_POINT('',(8.78085409196639,-16.6164222996225,0.));
#31676=CARTESIAN_POINT('',(7.17742576545784,-13.5821796255734,0.));
#31677=CARTESIAN_POINT('Origin',(1.32561760672361,-16.3182450637544,0.));
#31678=CARTESIAN_POINT('',(1.24464902580963,-15.3215284094816,0.));
#31679=CARTESIAN_POINT('',(2.315527719476,-16.1765483147777,0.));
#31680=CARTESIAN_POINT('Origin',(1.32561760672361,-16.3182450637544,0.));
#31681=CARTESIAN_POINT('',(2.315527719476,-16.1765483147777,15.));
#31682=CARTESIAN_POINT('',(2.315527719476,-16.1765483147777,0.));
#31683=CARTESIAN_POINT('',(1.24464902580963,-15.3215284094816,15.));
#31684=CARTESIAN_POINT('Origin',(1.32561760672361,-16.3182450637544,15.));
#31685=CARTESIAN_POINT('',(1.24464902580963,-15.3215284094816,0.));
#31686=CARTESIAN_POINT('Origin',(2.17674545777935,-15.2069991521022,0.));
#31687=CARTESIAN_POINT('',(2.66302778805429,-18.6042245638953,0.));
#31688=CARTESIAN_POINT('',(2.17674545777935,-15.2069991521022,0.));
#31689=CARTESIAN_POINT('',(2.66302778805429,-18.6042245638953,15.));
#31690=CARTESIAN_POINT('',(2.66302778805429,-18.6042245638953,0.));
#31691=CARTESIAN_POINT('',(2.17674545777935,-15.2069991521022,15.));
#31692=CARTESIAN_POINT('Origin',(-1.32561760672361,-16.3182450637544,0.));
#31693=CARTESIAN_POINT('',(-1.24464902580964,-15.3215284094816,15.));
#31694=CARTESIAN_POINT('',(-2.315527719476,-16.1765483147777,15.));
#31695=CARTESIAN_POINT('Origin',(-1.32561760672361,-16.3182450637544,15.));
#31696=CARTESIAN_POINT('',(-2.315527719476,-16.1765483147777,0.));
#31697=CARTESIAN_POINT('',(-2.315527719476,-16.1765483147777,0.));
#31698=CARTESIAN_POINT('',(-1.24464902580964,-15.3215284094816,0.));
#31699=CARTESIAN_POINT('Origin',(-1.32561760672361,-16.3182450637544,0.));
#31700=CARTESIAN_POINT('',(-1.24464902580964,-15.3215284094816,0.));
#31701=CARTESIAN_POINT('Origin',(-2.6630277880543,-18.6042245638953,0.));
#31702=CARTESIAN_POINT('',(-2.6630277880543,-18.6042245638953,15.));
#31703=CARTESIAN_POINT('',(-2.17674545777936,-15.2069991521022,15.));
#31704=CARTESIAN_POINT('',(-2.6630277880543,-18.6042245638953,0.));
#31705=CARTESIAN_POINT('',(-2.6630277880543,-18.6042245638953,0.));
#31706=CARTESIAN_POINT('',(-2.17674545777936,-15.2069991521022,0.));
#31707=CARTESIAN_POINT('Origin',(-8.51917661988722,-13.9809160543638,0.));
#31708=CARTESIAN_POINT('',(-7.9988262277612,-13.1269632047203,0.));
#31709=CARTESIAN_POINT('',(-7.63503525642066,-14.448135541765,0.));
#31710=CARTESIAN_POINT('Origin',(-8.51917661988722,-13.9809160543638,0.));
#31711=CARTESIAN_POINT('',(-7.63503525642066,-14.448135541765,15.));
#31712=CARTESIAN_POINT('',(-7.63503525642066,-14.448135541765,0.));
#31713=CARTESIAN_POINT('',(-7.9988262277612,-13.1269632047203,15.));
#31714=CARTESIAN_POINT('Origin',(-8.51917661988722,-13.9809160543638,15.));
#31715=CARTESIAN_POINT('',(-7.9988262277612,-13.1269632047203,0.));
#31716=CARTESIAN_POINT('Origin',(-7.17742576545785,-13.5821796255734,0.));
#31717=CARTESIAN_POINT('',(-8.7808540919664,-16.6164222996225,0.));
#31718=CARTESIAN_POINT('',(-7.17742576545785,-13.5821796255734,0.));
#31719=CARTESIAN_POINT('',(-8.7808540919664,-16.6164222996225,15.));
#31720=CARTESIAN_POINT('',(-8.7808540919664,-16.6164222996225,0.));
#31721=CARTESIAN_POINT('',(-7.17742576545785,-13.5821796255734,15.));
#31722=CARTESIAN_POINT('Origin',(-10.6640709636513,-12.422559095541,0.));
#31723=CARTESIAN_POINT('',(-10.0127106555856,-11.6637905214181,15.));
#31724=CARTESIAN_POINT('',(-11.3816378084254,-11.7260694522002,15.));
#31725=CARTESIAN_POINT('Origin',(-10.6640709636513,-12.422559095541,15.));
#31726=CARTESIAN_POINT('',(-11.3816378084254,-11.7260694522002,0.));
#31727=CARTESIAN_POINT('',(-11.3816378084254,-11.7260694522002,0.));
#31728=CARTESIAN_POINT('',(-10.0127106555856,-11.6637905214181,0.));
#31729=CARTESIAN_POINT('Origin',(-10.6640709636513,-12.422559095541,0.));
#31730=CARTESIAN_POINT('',(-10.0127106555856,-11.6637905214181,0.));
#31731=CARTESIAN_POINT('Origin',(-13.0897235660237,-13.4858453790958,0.));
#31732=CARTESIAN_POINT('',(-13.0897235660237,-13.4858453790958,15.));
#31733=CARTESIAN_POINT('',(-10.6994739010018,-11.0232618694188,15.));
#31734=CARTESIAN_POINT('',(-13.0897235660237,-13.4858453790958,0.));
#31735=CARTESIAN_POINT('',(-13.0897235660237,-13.4858453790958,0.));
#31736=CARTESIAN_POINT('',(-10.6994739010018,-11.0232618694188,0.));
#31737=CARTESIAN_POINT('Origin',(-15.1099349338646,-6.30335230606528,0.));
#31738=CARTESIAN_POINT('',(-14.1870217324314,-5.91834422482503,0.));
#31739=CARTESIAN_POINT('',(-14.6692742696684,-7.20102606586344,0.));
#31740=CARTESIAN_POINT('Origin',(-15.1099349338646,-6.30335230606528,0.));
#31741=CARTESIAN_POINT('',(-14.6692742696684,-7.20102606586344,15.));
#31742=CARTESIAN_POINT('',(-14.6692742696684,-7.20102606586344,0.));
#31743=CARTESIAN_POINT('',(-14.1870217324314,-5.91834422482503,15.));
#31744=CARTESIAN_POINT('Origin',(-15.1099349338646,-6.30335230606528,15.));
#31745=CARTESIAN_POINT('',(-14.1870217324314,-5.91834422482503,0.));
#31746=CARTESIAN_POINT('Origin',(-13.7900642980194,-6.76942912338193,0.));
#31747=CARTESIAN_POINT('',(-16.8707481591095,-8.28171148831561,0.));
#31748=CARTESIAN_POINT('',(-13.7900642980194,-6.76942912338193,0.));
#31749=CARTESIAN_POINT('',(-16.8707481591095,-8.28171148831561,15.));
#31750=CARTESIAN_POINT('',(-16.8707481591095,-8.28171148831561,0.));
#31751=CARTESIAN_POINT('',(-13.7900642980194,-6.76942912338193,15.));
#31752=CARTESIAN_POINT('Origin',(-15.9292116709051,-3.78187778008512,0.));
#31753=CARTESIAN_POINT('',(-14.9562571344462,-3.5508810918317,15.));
#31754=CARTESIAN_POINT('',(-16.1003491021971,-2.79663061332402,15.));
#31755=CARTESIAN_POINT('Origin',(-15.9292116709051,-3.78187778008512,15.));
#31756=CARTESIAN_POINT('',(-16.1003491021971,-2.79663061332402,0.));
#31757=CARTESIAN_POINT('',(-16.1003491021971,-2.79663061332403,0.));
#31758=CARTESIAN_POINT('',(-14.9562571344462,-3.5508810918317,0.));
#31759=CARTESIAN_POINT('Origin',(-15.9292116709051,-3.78187778008512,0.));
#31760=CARTESIAN_POINT('',(-14.9562571344462,-3.5508810918317,0.));
#31761=CARTESIAN_POINT('Origin',(-18.5165898451125,-3.21633162650739,0.));
#31762=CARTESIAN_POINT('',(-18.5165898451125,-3.21633162650739,15.));
#31763=CARTESIAN_POINT('',(-15.135366975784,-2.62901321950806,15.));
#31764=CARTESIAN_POINT('',(-18.5165898451125,-3.21633162650739,0.));
#31765=CARTESIAN_POINT('',(-18.5165898451125,-3.21633162650739,0.));
#31766=CARTESIAN_POINT('',(-15.135366975784,-2.62901321950806,0.));
#31767=CARTESIAN_POINT('Origin',(-15.9292116709051,3.78187778008512,0.));
#31768=CARTESIAN_POINT('',(-14.9562571344462,3.5508810918317,0.));
#31769=CARTESIAN_POINT('',(-16.1003491021971,2.79663061332403,0.));
#31770=CARTESIAN_POINT('Origin',(-15.9292116709051,3.78187778008512,0.));
#31771=CARTESIAN_POINT('',(-16.1003491021971,2.79663061332403,15.));
#31772=CARTESIAN_POINT('',(-16.1003491021971,2.79663061332403,0.));
#31773=CARTESIAN_POINT('',(-14.9562571344462,3.5508810918317,15.));
#31774=CARTESIAN_POINT('Origin',(-15.9292116709051,3.78187778008512,15.));
#31775=CARTESIAN_POINT('',(-14.9562571344462,3.5508810918317,0.));
#31776=CARTESIAN_POINT('Origin',(-15.135366975784,2.62901321950807,0.));
#31777=CARTESIAN_POINT('',(-18.5165898451125,3.2163316265074,0.));
#31778=CARTESIAN_POINT('',(-15.135366975784,2.62901321950807,0.));
#31779=CARTESIAN_POINT('',(-18.5165898451125,3.2163316265074,15.));
#31780=CARTESIAN_POINT('',(-18.5165898451125,3.2163316265074,0.));
#31781=CARTESIAN_POINT('',(-15.135366975784,2.62901321950807,15.));
#31782=CARTESIAN_POINT('Origin',(-15.1099349338646,6.30335230606528,0.));
#31783=CARTESIAN_POINT('',(-14.1870217324314,5.91834422482504,15.));
#31784=CARTESIAN_POINT('',(-14.6692742696684,7.20102606586345,15.));
#31785=CARTESIAN_POINT('Origin',(-15.1099349338646,6.30335230606528,15.));
#31786=CARTESIAN_POINT('',(-14.6692742696684,7.20102606586345,0.));
#31787=CARTESIAN_POINT('',(-14.6692742696684,7.20102606586345,0.));
#31788=CARTESIAN_POINT('',(-14.1870217324314,5.91834422482504,0.));
#31789=CARTESIAN_POINT('Origin',(-15.1099349338646,6.30335230606528,0.));
#31790=CARTESIAN_POINT('',(-14.1870217324314,5.91834422482504,0.));
#31791=CARTESIAN_POINT('Origin',(-16.8707481591095,8.28171148831561,0.));
#31792=CARTESIAN_POINT('',(-16.8707481591095,8.28171148831561,15.));
#31793=CARTESIAN_POINT('',(-13.7900642980194,6.76942912338193,15.));
#31794=CARTESIAN_POINT('',(-16.8707481591095,8.28171148831561,0.));
#31795=CARTESIAN_POINT('',(-16.8707481591095,8.28171148831561,0.));
#31796=CARTESIAN_POINT('',(-13.7900642980194,6.76942912338193,0.));
#31797=CARTESIAN_POINT('Origin',(-10.6640709636513,12.422559095541,0.));
#31798=CARTESIAN_POINT('',(-10.0127106555856,11.6637905214181,0.));
#31799=CARTESIAN_POINT('',(-11.3816378084254,11.7260694522002,0.));
#31800=CARTESIAN_POINT('Origin',(-10.6640709636513,12.422559095541,0.));
#31801=CARTESIAN_POINT('',(-11.3816378084254,11.7260694522002,15.));
#31802=CARTESIAN_POINT('',(-11.3816378084254,11.7260694522002,0.));
#31803=CARTESIAN_POINT('',(-10.0127106555856,11.6637905214181,15.));
#31804=CARTESIAN_POINT('Origin',(-10.6640709636513,12.422559095541,15.));
#31805=CARTESIAN_POINT('',(-10.0127106555856,11.6637905214181,0.));
#31806=CARTESIAN_POINT('Origin',(-10.6994739010018,11.0232618694188,0.));
#31807=CARTESIAN_POINT('',(-13.0897235660237,13.4858453790958,0.));
#31808=CARTESIAN_POINT('',(-10.6994739010018,11.0232618694188,0.));
#31809=CARTESIAN_POINT('',(-13.0897235660237,13.4858453790958,15.));
#31810=CARTESIAN_POINT('',(-13.0897235660237,13.4858453790958,0.));
#31811=CARTESIAN_POINT('',(-10.6994739010018,11.0232618694188,15.));
#31812=CARTESIAN_POINT('Origin',(-8.51917661988722,13.9809160543638,0.));
#31813=CARTESIAN_POINT('',(-7.9988262277612,13.1269632047203,15.));
#31814=CARTESIAN_POINT('',(-7.63503525642066,14.448135541765,15.));
#31815=CARTESIAN_POINT('Origin',(-8.51917661988722,13.9809160543638,15.));
#31816=CARTESIAN_POINT('',(-7.63503525642066,14.448135541765,0.));
#31817=CARTESIAN_POINT('',(-7.63503525642066,14.448135541765,0.));
#31818=CARTESIAN_POINT('',(-7.9988262277612,13.1269632047203,0.));
#31819=CARTESIAN_POINT('Origin',(-8.51917661988722,13.9809160543638,0.));
#31820=CARTESIAN_POINT('',(-7.9988262277612,13.1269632047203,0.));
#31821=CARTESIAN_POINT('Origin',(-8.78085409196639,16.6164222996225,0.));
#31822=CARTESIAN_POINT('',(-8.78085409196639,16.6164222996225,15.));
#31823=CARTESIAN_POINT('',(-7.17742576545784,13.5821796255734,15.));
#31824=CARTESIAN_POINT('',(-8.78085409196639,16.6164222996225,0.));
#31825=CARTESIAN_POINT('',(-8.78085409196639,16.6164222996225,0.));
#31826=CARTESIAN_POINT('',(-7.17742576545784,13.5821796255734,0.));
#31827=CARTESIAN_POINT('Origin',(-1.32561760672361,16.3182450637544,0.));
#31828=CARTESIAN_POINT('',(-1.24464902580963,15.3215284094816,0.));
#31829=CARTESIAN_POINT('',(-2.315527719476,16.1765483147777,0.));
#31830=CARTESIAN_POINT('Origin',(-1.32561760672361,16.3182450637544,0.));
#31831=CARTESIAN_POINT('',(-2.315527719476,16.1765483147777,15.));
#31832=CARTESIAN_POINT('',(-2.315527719476,16.1765483147777,0.));
#31833=CARTESIAN_POINT('',(-1.24464902580963,15.3215284094816,15.));
#31834=CARTESIAN_POINT('Origin',(-1.32561760672361,16.3182450637544,15.));
#31835=CARTESIAN_POINT('',(-1.24464902580963,15.3215284094816,0.));
#31836=CARTESIAN_POINT('Origin',(-2.17674545777935,15.2069991521022,0.));
#31837=CARTESIAN_POINT('',(-2.66302778805429,18.6042245638953,0.));
#31838=CARTESIAN_POINT('',(-2.17674545777935,15.2069991521022,0.));
#31839=CARTESIAN_POINT('',(-2.66302778805429,18.6042245638953,15.));
#31840=CARTESIAN_POINT('',(-2.66302778805429,18.6042245638953,0.));
#31841=CARTESIAN_POINT('',(-2.17674545777935,15.2069991521022,15.));
#31842=CARTESIAN_POINT('Origin',(1.32561760672361,16.3182450637544,0.));
#31843=CARTESIAN_POINT('',(1.24464902580964,15.3215284094816,15.));
#31844=CARTESIAN_POINT('',(2.315527719476,16.1765483147777,15.));
#31845=CARTESIAN_POINT('Origin',(1.32561760672361,16.3182450637544,15.));
#31846=CARTESIAN_POINT('',(2.315527719476,16.1765483147777,0.));
#31847=CARTESIAN_POINT('',(2.315527719476,16.1765483147777,0.));
#31848=CARTESIAN_POINT('',(1.24464902580964,15.3215284094816,0.));
#31849=CARTESIAN_POINT('Origin',(1.32561760672361,16.3182450637544,0.));
#31850=CARTESIAN_POINT('',(1.24464902580964,15.3215284094816,0.));
#31851=CARTESIAN_POINT('Origin',(2.66302778805429,18.6042245638953,0.));
#31852=CARTESIAN_POINT('',(2.66302778805429,18.6042245638953,15.));
#31853=CARTESIAN_POINT('',(2.17674545777935,15.2069991521022,15.));
#31854=CARTESIAN_POINT('',(2.66302778805429,18.6042245638953,0.));
#31855=CARTESIAN_POINT('',(2.66302778805429,18.6042245638953,0.));
#31856=CARTESIAN_POINT('',(2.17674545777935,15.2069991521022,0.));
#31857=CARTESIAN_POINT('Origin',(8.51917661988723,13.9809160543638,0.));
#31858=CARTESIAN_POINT('',(7.9988262277612,13.1269632047203,0.));
#31859=CARTESIAN_POINT('',(7.63503525642066,14.448135541765,0.));
#31860=CARTESIAN_POINT('Origin',(8.51917661988723,13.9809160543638,0.));
#31861=CARTESIAN_POINT('',(7.63503525642066,14.448135541765,15.));
#31862=CARTESIAN_POINT('',(7.63503525642066,14.448135541765,0.));
#31863=CARTESIAN_POINT('',(7.9988262277612,13.1269632047203,15.));
#31864=CARTESIAN_POINT('Origin',(8.51917661988723,13.9809160543638,15.));
#31865=CARTESIAN_POINT('',(7.9988262277612,13.1269632047203,0.));
#31866=CARTESIAN_POINT('Origin',(7.17742576545784,13.5821796255734,0.));
#31867=CARTESIAN_POINT('',(8.78085409196639,16.6164222996225,0.));
#31868=CARTESIAN_POINT('',(7.17742576545784,13.5821796255734,0.));
#31869=CARTESIAN_POINT('',(8.78085409196639,16.6164222996225,15.));
#31870=CARTESIAN_POINT('',(8.78085409196639,16.6164222996225,0.));
#31871=CARTESIAN_POINT('',(7.17742576545784,13.5821796255734,15.));
#31872=CARTESIAN_POINT('Origin',(10.6640709636513,12.422559095541,0.));
#31873=CARTESIAN_POINT('',(10.0127106555856,11.6637905214181,15.));
#31874=CARTESIAN_POINT('',(11.3816378084254,11.7260694522002,15.));
#31875=CARTESIAN_POINT('Origin',(10.6640709636513,12.422559095541,15.));
#31876=CARTESIAN_POINT('',(11.3816378084254,11.7260694522002,0.));
#31877=CARTESIAN_POINT('',(11.3816378084254,11.7260694522002,0.));
#31878=CARTESIAN_POINT('',(10.0127106555856,11.6637905214181,0.));
#31879=CARTESIAN_POINT('Origin',(10.6640709636513,12.422559095541,0.));
#31880=CARTESIAN_POINT('',(10.0127106555856,11.6637905214181,0.));
#31881=CARTESIAN_POINT('Origin',(13.0897235660237,13.4858453790958,0.));
#31882=CARTESIAN_POINT('',(13.0897235660237,13.4858453790958,15.));
#31883=CARTESIAN_POINT('',(10.6994739010018,11.0232618694188,15.));
#31884=CARTESIAN_POINT('',(13.0897235660237,13.4858453790958,0.));
#31885=CARTESIAN_POINT('',(13.0897235660237,13.4858453790958,0.));
#31886=CARTESIAN_POINT('',(10.6994739010018,11.0232618694188,0.));
#31887=CARTESIAN_POINT('Origin',(15.1099349338646,6.30335230606528,0.));
#31888=CARTESIAN_POINT('',(14.1870217324314,5.91834422482504,0.));
#31889=CARTESIAN_POINT('',(14.6692742696684,7.20102606586344,0.));
#31890=CARTESIAN_POINT('Origin',(15.1099349338646,6.30335230606528,0.));
#31891=CARTESIAN_POINT('',(14.6692742696684,7.20102606586344,15.));
#31892=CARTESIAN_POINT('',(14.6692742696684,7.20102606586344,0.));
#31893=CARTESIAN_POINT('',(14.1870217324314,5.91834422482504,15.));
#31894=CARTESIAN_POINT('Origin',(15.1099349338646,6.30335230606528,15.));
#31895=CARTESIAN_POINT('',(14.1870217324314,5.91834422482504,0.));
#31896=CARTESIAN_POINT('Origin',(13.7900642980194,6.76942912338193,0.));
#31897=CARTESIAN_POINT('',(16.8707481591095,8.28171148831561,0.));
#31898=CARTESIAN_POINT('',(13.7900642980194,6.76942912338193,0.));
#31899=CARTESIAN_POINT('',(16.8707481591095,8.28171148831561,15.));
#31900=CARTESIAN_POINT('',(16.8707481591095,8.28171148831561,0.));
#31901=CARTESIAN_POINT('',(13.7900642980194,6.76942912338193,15.));
#31902=CARTESIAN_POINT('Ctrl Pts',(20.0837475345526,-13.1393715591102,0.));
#31903=CARTESIAN_POINT('Ctrl Pts',(20.0837475345526,-13.1393715591102,18.));
#31904=CARTESIAN_POINT('Ctrl Pts',(20.0780177478283,-13.1220955868173,0.));
#31905=CARTESIAN_POINT('Ctrl Pts',(20.0780177478283,-13.1220955868173,18.));
#31906=CARTESIAN_POINT('Ctrl Pts',(20.0665110891946,-13.0875783330728,0.));
#31907=CARTESIAN_POINT('Ctrl Pts',(20.0665110891946,-13.0875783330728,18.));
#31908=CARTESIAN_POINT('Ctrl Pts',(20.0491098457044,-13.0359065249991,0.));
#31909=CARTESIAN_POINT('Ctrl Pts',(20.0491098457044,-13.0359065249991,18.));
#31910=CARTESIAN_POINT('Ctrl Pts',(20.0256255826397,-12.9672189949731,0.));
#31911=CARTESIAN_POINT('Ctrl Pts',(20.0256255826397,-12.9672189949731,18.));
#31912=CARTESIAN_POINT('Ctrl Pts',(19.9957986945787,-12.8817072534696,0.));
#31913=CARTESIAN_POINT('Ctrl Pts',(19.9957986945787,-12.8817072534696,18.));
#31914=CARTESIAN_POINT('Ctrl Pts',(19.9654995335894,-12.7965444294443,0.));
#31915=CARTESIAN_POINT('Ctrl Pts',(19.9654995335894,-12.7965444294443,18.));
#31916=CARTESIAN_POINT('Ctrl Pts',(19.9347273847264,-12.7117325003719,0.));
#31917=CARTESIAN_POINT('Ctrl Pts',(19.9347273847264,-12.7117325003719,18.));
#31918=CARTESIAN_POINT('Ctrl Pts',(19.9034816813503,-12.6272742843372,0.));
#31919=CARTESIAN_POINT('Ctrl Pts',(19.9034816813503,-12.6272742843372,18.));
#31920=CARTESIAN_POINT('Ctrl Pts',(19.8717621942733,-12.5431736030596,0.));
#31921=CARTESIAN_POINT('Ctrl Pts',(19.8717621942733,-12.5431736030596,18.));
#31922=CARTESIAN_POINT('Ctrl Pts',(19.839568972011,-12.4594350764989,0.));
#31923=CARTESIAN_POINT('Ctrl Pts',(19.839568972011,-12.4594350764989,18.));
#31924=CARTESIAN_POINT('Ctrl Pts',(19.8069022248387,-12.3760638341708,0.));
#31925=CARTESIAN_POINT('Ctrl Pts',(19.8069022248387,-12.3760638341708,18.));
#31926=CARTESIAN_POINT('Ctrl Pts',(19.7737622285562,-12.2930652417987,0.));
#31927=CARTESIAN_POINT('Ctrl Pts',(19.7737622285562,-12.2930652417987,18.));
#31928=CARTESIAN_POINT('Ctrl Pts',(19.7401492304335,-12.2104446447874,0.));
#31929=CARTESIAN_POINT('Ctrl Pts',(19.7401492304335,-12.2104446447874,18.));
#31930=CARTESIAN_POINT('Ctrl Pts',(19.7060633406705,-12.1282070378972,0.));
#31931=CARTESIAN_POINT('Ctrl Pts',(19.7060633406705,-12.1282070378972,18.));
#31932=CARTESIAN_POINT('Ctrl Pts',(19.6715045149944,-12.0463570680309,0.));
#31933=CARTESIAN_POINT('Ctrl Pts',(19.6715045149944,-12.0463570680309,18.));
#31934=CARTESIAN_POINT('Ctrl Pts',(19.6364725931695,-11.9648992312094,0.));
#31935=CARTESIAN_POINT('Ctrl Pts',(19.6364725931695,-11.9648992312094,18.));
#31936=CARTESIAN_POINT('Ctrl Pts',(19.6009673241771,-11.8838380136222,0.));
#31937=CARTESIAN_POINT('Ctrl Pts',(19.6009673241771,-11.8838380136222,18.));
#31938=CARTESIAN_POINT('Ctrl Pts',(19.5649883985826,-11.8031780389346,0.));
#31939=CARTESIAN_POINT('Ctrl Pts',(19.5649883985826,-11.8031780389346,18.));
#31940=CARTESIAN_POINT('Ctrl Pts',(19.5285354853626,-11.722924244195,0.));
#31941=CARTESIAN_POINT('Ctrl Pts',(19.5285354853626,-11.722924244195,18.));
#31942=CARTESIAN_POINT('Ctrl Pts',(19.4916082541529,-11.6430819099846,0.));
#31943=CARTESIAN_POINT('Ctrl Pts',(19.4916082541529,-11.6430819099846,18.));
#31944=CARTESIAN_POINT('Ctrl Pts',(19.4542063779876,-11.5636565297382,0.));
#31945=CARTESIAN_POINT('Ctrl Pts',(19.4542063779876,-11.5636565297382,18.));
#31946=CARTESIAN_POINT('Ctrl Pts',(19.4163295466324,-11.4846537135043,0.));
#31947=CARTESIAN_POINT('Ctrl Pts',(19.4163295466324,-11.4846537135043,18.));
#31948=CARTESIAN_POINT('Ctrl Pts',(19.3779774742875,-11.4060790880015,0.));
#31949=CARTESIAN_POINT('Ctrl Pts',(19.3779774742875,-11.4060790880015,18.));
#31950=CARTESIAN_POINT('Ctrl Pts',(19.3391499248083,-11.3279381634523,0.));
#31951=CARTESIAN_POINT('Ctrl Pts',(19.3391499248083,-11.3279381634523,18.));
#31952=CARTESIAN_POINT('Ctrl Pts',(19.2998466936739,-11.2502363198588,0.));
#31953=CARTESIAN_POINT('Ctrl Pts',(19.2998466936739,-11.2502363198588,18.));
#31954=CARTESIAN_POINT('Ctrl Pts',(19.2600675167206,-11.1729790050543,0.));
#31955=CARTESIAN_POINT('Ctrl Pts',(19.2600675167206,-11.1729790050543,18.));
#31956=CARTESIAN_POINT('Ctrl Pts',(19.2198119937835,-11.0961718903994,0.));
#31957=CARTESIAN_POINT('Ctrl Pts',(19.2198119937835,-11.0961718903994,18.));
#31958=CARTESIAN_POINT('Ctrl Pts',(19.1790795192393,-11.0198210228993,0.));
#31959=CARTESIAN_POINT('Ctrl Pts',(19.1790795192393,-11.0198210228993,18.));
#31960=CARTESIAN_POINT('Ctrl Pts',(19.1378691901023,-10.9439330179206,0.));
#31961=CARTESIAN_POINT('Ctrl Pts',(19.1378691901023,-10.9439330179206,18.));
#31962=CARTESIAN_POINT('Ctrl Pts',(19.0961797996403,-10.868515097783,0.));
#31963=CARTESIAN_POINT('Ctrl Pts',(19.0961797996403,-10.868515097783,18.));
#31964=CARTESIAN_POINT('Ctrl Pts',(19.0540100416943,-10.7935747414879,0.));
#31965=CARTESIAN_POINT('Ctrl Pts',(19.0540100416943,-10.7935747414879,18.));
#31966=CARTESIAN_POINT('Ctrl Pts',(19.0113586878152,-10.7191193896586,0.));
#31967=CARTESIAN_POINT('Ctrl Pts',(19.0113586878152,-10.7191193896586,18.));
#31968=CARTESIAN_POINT('Ctrl Pts',(18.9682247574834,-10.6451561585969,0.));
#31969=CARTESIAN_POINT('Ctrl Pts',(18.9682247574834,-10.6451561585969,18.));
#31970=CARTESIAN_POINT('Ctrl Pts',(18.9246077453188,-10.5716914651544,0.));
#31971=CARTESIAN_POINT('Ctrl Pts',(18.9246077453188,-10.5716914651544,18.));
#31972=CARTESIAN_POINT('Ctrl Pts',(18.8805076729356,-10.4987309368494,0.));
#31973=CARTESIAN_POINT('Ctrl Pts',(18.8805076729356,-10.4987309368494,18.));
#31974=CARTESIAN_POINT('Ctrl Pts',(18.8359245594214,-10.4262802670211,0.));
#31975=CARTESIAN_POINT('Ctrl Pts',(18.8359245594214,-10.4262802670211,18.));
#31976=CARTESIAN_POINT('Ctrl Pts',(18.7908579693851,-10.3543459451258,0.));
#31977=CARTESIAN_POINT('Ctrl Pts',(18.7908579693851,-10.3543459451258,18.));
#31978=CARTESIAN_POINT('Ctrl Pts',(18.7453065790062,-10.2829359603685,0.));
#31979=CARTESIAN_POINT('Ctrl Pts',(18.7453065790062,-10.2829359603685,18.));
#31980=CARTESIAN_POINT('Ctrl Pts',(18.699267629819,-10.2120606864872,0.));
#31981=CARTESIAN_POINT('Ctrl Pts',(18.699267629819,-10.2120606864872,18.));
#31982=CARTESIAN_POINT('Ctrl Pts',(18.6527367592664,-10.1417331637795,0.));
#31983=CARTESIAN_POINT('Ctrl Pts',(18.6527367592664,-10.1417331637795,18.));
#31984=CARTESIAN_POINT('Ctrl Pts',(18.605709190442,-10.0719672018851,0.));
#31985=CARTESIAN_POINT('Ctrl Pts',(18.605709190442,-10.0719672018851,18.));
#31986=CARTESIAN_POINT('Ctrl Pts',(18.5581807679204,-10.0027757313807,0.));
#31987=CARTESIAN_POINT('Ctrl Pts',(18.5581807679204,-10.0027757313807,18.));
#31988=CARTESIAN_POINT('Ctrl Pts',(18.5101489409161,-9.93416923996829,0.));
#31989=CARTESIAN_POINT('Ctrl Pts',(18.5101489409161,-9.93416923996829,18.));
#31990=CARTESIAN_POINT('Ctrl Pts',(18.461614050347,-9.86615372541685,0.));
#31991=CARTESIAN_POINT('Ctrl Pts',(18.461614050347,-9.86615372541685,18.));
#31992=CARTESIAN_POINT('Ctrl Pts',(18.4125796444662,-9.79873019947434,0.));
#31993=CARTESIAN_POINT('Ctrl Pts',(18.4125796444662,-9.79873019947434,18.));
#31994=CARTESIAN_POINT('Ctrl Pts',(18.3630495772677,-9.73189932619939,0.));
#31995=CARTESIAN_POINT('Ctrl Pts',(18.3630495772677,-9.73189932619939,18.));
#31996=CARTESIAN_POINT('Ctrl Pts',(18.3130254811852,-9.6656654640326,0.));
#31997=CARTESIAN_POINT('Ctrl Pts',(18.3130254811852,-9.6656654640326,18.));
#31998=CARTESIAN_POINT('Ctrl Pts',(18.2625044208165,-9.60004042085347,0.));
#31999=CARTESIAN_POINT('Ctrl Pts',(18.2625044208165,-9.60004042085347,18.));
#32000=CARTESIAN_POINT('Ctrl Pts',(18.2114756946126,-9.53504856811686,0.));
#32001=CARTESIAN_POINT('Ctrl Pts',(18.2114756946126,-9.53504856811686,18.));
#32002=CARTESIAN_POINT('Ctrl Pts',(18.1599204445014,-9.47072748065832,0.));
#32003=CARTESIAN_POINT('Ctrl Pts',(18.1599204445014,-9.47072748065832,18.));
#32004=CARTESIAN_POINT('Ctrl Pts',(18.1078184146735,-9.40711718355464,0.));
#32005=CARTESIAN_POINT('Ctrl Pts',(18.1078184146735,-9.40711718355464,18.));
#32006=CARTESIAN_POINT('Ctrl Pts',(18.0551538338035,-9.34425079614396,0.));
#32007=CARTESIAN_POINT('Ctrl Pts',(18.0551538338035,-9.34425079614396,18.));
#32008=CARTESIAN_POINT('Ctrl Pts',(18.0019206847747,-9.28214615574471,0.));
#32009=CARTESIAN_POINT('Ctrl Pts',(18.0019206847747,-9.28214615574471,18.));
#32010=CARTESIAN_POINT('Ctrl Pts',(17.9481305624284,-9.22079331175917,0.));
#32011=CARTESIAN_POINT('Ctrl Pts',(17.9481305624284,-9.22079331175917,18.));
#32012=CARTESIAN_POINT('Ctrl Pts',(17.8938116696237,-9.1601561636161,0.));
#32013=CARTESIAN_POINT('Ctrl Pts',(17.8938116696237,-9.1601561636161,18.));
#32014=CARTESIAN_POINT('Ctrl Pts',(17.8389924349283,-9.10019864472208,0.));
#32015=CARTESIAN_POINT('Ctrl Pts',(17.8389924349283,-9.10019864472208,18.));
#32016=CARTESIAN_POINT('Ctrl Pts',(17.7836872744016,-9.04090748239097,0.));
#32017=CARTESIAN_POINT('Ctrl Pts',(17.7836872744016,-9.04090748239097,18.));
#32018=CARTESIAN_POINT('Ctrl Pts',(17.7278841963319,-8.98231202490686,0.));
#32019=CARTESIAN_POINT('Ctrl Pts',(17.7278841963319,-8.98231202490686,18.));
#32020=CARTESIAN_POINT('Ctrl Pts',(17.6715250120654,-8.92451585185175,0.));
#32021=CARTESIAN_POINT('Ctrl Pts',(17.6715250120654,-8.92451585185175,18.));
#32022=CARTESIAN_POINT('Ctrl Pts',(17.614513388992,-8.86768402115344,0.));
#32023=CARTESIAN_POINT('Ctrl Pts',(17.614513388992,-8.86768402115344,18.));
#32024=CARTESIAN_POINT('Ctrl Pts',(17.5567525798882,-8.81198307239551,0.));
#32025=CARTESIAN_POINT('Ctrl Pts',(17.5567525798882,-8.81198307239551,18.));
#32026=CARTESIAN_POINT('Ctrl Pts',(17.4981785296199,-8.75752832625955,0.));
#32027=CARTESIAN_POINT('Ctrl Pts',(17.4981785296199,-8.75752832625955,18.));
#32028=CARTESIAN_POINT('Ctrl Pts',(17.438788019753,-8.70433925112174,0.));
#32029=CARTESIAN_POINT('Ctrl Pts',(17.438788019753,-8.70433925112174,18.));
#32030=CARTESIAN_POINT('Ctrl Pts',(17.3786861166843,-8.65226368112816,0.));
#32031=CARTESIAN_POINT('Ctrl Pts',(17.3786861166843,-8.65226368112816,18.));
#32032=CARTESIAN_POINT('Ctrl Pts',(17.3180459442745,-8.60104338529165,0.));
#32033=CARTESIAN_POINT('Ctrl Pts',(17.3180459442745,-8.60104338529165,18.));
#32034=CARTESIAN_POINT('Ctrl Pts',(17.2570167183611,-8.55046295192434,0.));
#32035=CARTESIAN_POINT('Ctrl Pts',(17.2570167183611,-8.55046295192434,18.));
#32036=CARTESIAN_POINT('Ctrl Pts',(17.1956428575086,-8.50048099003883,0.));
#32037=CARTESIAN_POINT('Ctrl Pts',(17.1956428575086,-8.50048099003883,18.));
#32038=CARTESIAN_POINT('Ctrl Pts',(17.1337886602855,-8.45135198307877,0.));
#32039=CARTESIAN_POINT('Ctrl Pts',(17.1337886602855,-8.45135198307877,18.));
#32040=CARTESIAN_POINT('Ctrl Pts',(17.071033847921,-8.40379607744266,0.));
#32041=CARTESIAN_POINT('Ctrl Pts',(17.071033847921,-8.40379607744266,18.));
#32042=CARTESIAN_POINT('Ctrl Pts',(17.0067806259695,-8.35882146841244,0.));
#32043=CARTESIAN_POINT('Ctrl Pts',(17.0067806259695,-8.35882146841244,18.));
#32044=CARTESIAN_POINT('Ctrl Pts',(16.9536879065132,-8.32573081382563,0.));
#32045=CARTESIAN_POINT('Ctrl Pts',(16.9536879065132,-8.32573081382563,18.));
#32046=CARTESIAN_POINT('Ctrl Pts',(16.9126979078877,-8.30290517019115,0.));
#32047=CARTESIAN_POINT('Ctrl Pts',(16.9126979078877,-8.30290517019115,18.));
#32048=CARTESIAN_POINT('Ctrl Pts',(16.8848228151885,-8.28862062120315,0.));
#32049=CARTESIAN_POINT('Ctrl Pts',(16.8848228151885,-8.28862062120315,18.));
#32050=CARTESIAN_POINT('Ctrl Pts',(16.8707481591095,-8.28171148831561,0.));
#32051=CARTESIAN_POINT('Ctrl Pts',(16.8707481591095,-8.28171148831561,18.));
#32052=CARTESIAN_POINT('',(20.0837475345525,-13.1393715591102,0.));
#32053=CARTESIAN_POINT('Ctrl Pts',(16.8707481591095,-8.28171148831561,0.));
#32054=CARTESIAN_POINT('Ctrl Pts',(16.8848228151885,-8.28862062120315,0.));
#32055=CARTESIAN_POINT('Ctrl Pts',(16.9126979078877,-8.30290517019115,0.));
#32056=CARTESIAN_POINT('Ctrl Pts',(16.9536879065132,-8.32573081382563,0.));
#32057=CARTESIAN_POINT('Ctrl Pts',(17.0067806259695,-8.35882146841244,0.));
#32058=CARTESIAN_POINT('Ctrl Pts',(17.071033847921,-8.40379607744266,0.));
#32059=CARTESIAN_POINT('Ctrl Pts',(17.1337886602855,-8.45135198307877,0.));
#32060=CARTESIAN_POINT('Ctrl Pts',(17.1956428575086,-8.50048099003883,0.));
#32061=CARTESIAN_POINT('Ctrl Pts',(17.2570167183611,-8.55046295192434,0.));
#32062=CARTESIAN_POINT('Ctrl Pts',(17.3180459442745,-8.60104338529165,0.));
#32063=CARTESIAN_POINT('Ctrl Pts',(17.3786861166843,-8.65226368112816,0.));
#32064=CARTESIAN_POINT('Ctrl Pts',(17.438788019753,-8.70433925112174,0.));
#32065=CARTESIAN_POINT('Ctrl Pts',(17.4981785296199,-8.75752832625955,0.));
#32066=CARTESIAN_POINT('Ctrl Pts',(17.5567525798882,-8.81198307239551,0.));
#32067=CARTESIAN_POINT('Ctrl Pts',(17.614513388992,-8.86768402115344,0.));
#32068=CARTESIAN_POINT('Ctrl Pts',(17.6715250120654,-8.92451585185175,0.));
#32069=CARTESIAN_POINT('Ctrl Pts',(17.7278841963319,-8.98231202490686,0.));
#32070=CARTESIAN_POINT('Ctrl Pts',(17.7836872744016,-9.04090748239097,0.));
#32071=CARTESIAN_POINT('Ctrl Pts',(17.8389924349283,-9.10019864472208,0.));
#32072=CARTESIAN_POINT('Ctrl Pts',(17.8938116696237,-9.1601561636161,0.));
#32073=CARTESIAN_POINT('Ctrl Pts',(17.9481305624284,-9.22079331175917,0.));
#32074=CARTESIAN_POINT('Ctrl Pts',(18.0019206847747,-9.28214615574471,0.));
#32075=CARTESIAN_POINT('Ctrl Pts',(18.0551538338035,-9.34425079614396,0.));
#32076=CARTESIAN_POINT('Ctrl Pts',(18.1078184146735,-9.40711718355464,0.));
#32077=CARTESIAN_POINT('Ctrl Pts',(18.1599204445014,-9.47072748065832,0.));
#32078=CARTESIAN_POINT('Ctrl Pts',(18.2114756946126,-9.53504856811686,0.));
#32079=CARTESIAN_POINT('Ctrl Pts',(18.2625044208165,-9.60004042085347,0.));
#32080=CARTESIAN_POINT('Ctrl Pts',(18.3130254811852,-9.6656654640326,0.));
#32081=CARTESIAN_POINT('Ctrl Pts',(18.3630495772677,-9.73189932619939,0.));
#32082=CARTESIAN_POINT('Ctrl Pts',(18.4125796444662,-9.79873019947434,0.));
#32083=CARTESIAN_POINT('Ctrl Pts',(18.461614050347,-9.86615372541685,0.));
#32084=CARTESIAN_POINT('Ctrl Pts',(18.5101489409161,-9.93416923996829,0.));
#32085=CARTESIAN_POINT('Ctrl Pts',(18.5581807679204,-10.0027757313807,0.));
#32086=CARTESIAN_POINT('Ctrl Pts',(18.605709190442,-10.0719672018851,0.));
#32087=CARTESIAN_POINT('Ctrl Pts',(18.6527367592664,-10.1417331637795,0.));
#32088=CARTESIAN_POINT('Ctrl Pts',(18.699267629819,-10.2120606864872,0.));
#32089=CARTESIAN_POINT('Ctrl Pts',(18.7453065790062,-10.2829359603685,0.));
#32090=CARTESIAN_POINT('Ctrl Pts',(18.7908579693851,-10.3543459451258,0.));
#32091=CARTESIAN_POINT('Ctrl Pts',(18.8359245594214,-10.4262802670211,0.));
#32092=CARTESIAN_POINT('Ctrl Pts',(18.8805076729356,-10.4987309368494,0.));
#32093=CARTESIAN_POINT('Ctrl Pts',(18.9246077453188,-10.5716914651544,0.));
#32094=CARTESIAN_POINT('Ctrl Pts',(18.9682247574834,-10.6451561585969,0.));
#32095=CARTESIAN_POINT('Ctrl Pts',(19.0113586878152,-10.7191193896586,0.));
#32096=CARTESIAN_POINT('Ctrl Pts',(19.0540100416943,-10.7935747414879,0.));
#32097=CARTESIAN_POINT('Ctrl Pts',(19.0961797996403,-10.868515097783,0.));
#32098=CARTESIAN_POINT('Ctrl Pts',(19.1378691901023,-10.9439330179206,0.));
#32099=CARTESIAN_POINT('Ctrl Pts',(19.1790795192393,-11.0198210228993,0.));
#32100=CARTESIAN_POINT('Ctrl Pts',(19.2198119937835,-11.0961718903994,0.));
#32101=CARTESIAN_POINT('Ctrl Pts',(19.2600675167206,-11.1729790050543,0.));
#32102=CARTESIAN_POINT('Ctrl Pts',(19.2998466936739,-11.2502363198588,0.));
#32103=CARTESIAN_POINT('Ctrl Pts',(19.3391499248083,-11.3279381634523,0.));
#32104=CARTESIAN_POINT('Ctrl Pts',(19.3779774742875,-11.4060790880015,0.));
#32105=CARTESIAN_POINT('Ctrl Pts',(19.4163295466324,-11.4846537135043,0.));
#32106=CARTESIAN_POINT('Ctrl Pts',(19.4542063779876,-11.5636565297382,0.));
#32107=CARTESIAN_POINT('Ctrl Pts',(19.4916082541529,-11.6430819099846,0.));
#32108=CARTESIAN_POINT('Ctrl Pts',(19.5285354853626,-11.722924244195,0.));
#32109=CARTESIAN_POINT('Ctrl Pts',(19.5649883985826,-11.8031780389346,0.));
#32110=CARTESIAN_POINT('Ctrl Pts',(19.6009673241771,-11.8838380136222,0.));
#32111=CARTESIAN_POINT('Ctrl Pts',(19.6364725931695,-11.9648992312094,0.));
#32112=CARTESIAN_POINT('Ctrl Pts',(19.6715045149944,-12.0463570680309,0.));
#32113=CARTESIAN_POINT('Ctrl Pts',(19.7060633406705,-12.1282070378972,0.));
#32114=CARTESIAN_POINT('Ctrl Pts',(19.7401492304335,-12.2104446447874,0.));
#32115=CARTESIAN_POINT('Ctrl Pts',(19.7737622285562,-12.2930652417987,0.));
#32116=CARTESIAN_POINT('Ctrl Pts',(19.8069022248387,-12.3760638341708,0.));
#32117=CARTESIAN_POINT('Ctrl Pts',(19.839568972011,-12.4594350764989,0.));
#32118=CARTESIAN_POINT('Ctrl Pts',(19.8717621942733,-12.5431736030596,0.));
#32119=CARTESIAN_POINT('Ctrl Pts',(19.9034816813503,-12.6272742843372,0.));
#32120=CARTESIAN_POINT('Ctrl Pts',(19.9347273847264,-12.7117325003719,0.));
#32121=CARTESIAN_POINT('Ctrl Pts',(19.9654995335894,-12.7965444294443,0.));
#32122=CARTESIAN_POINT('Ctrl Pts',(20.0018585267766,-12.8987398182747,0.));
#32123=CARTESIAN_POINT('Ctrl Pts',(20.0315673466055,-12.9843387891477,0.));
#32124=CARTESIAN_POINT('Ctrl Pts',(20.054957345404,-13.0530957702829,0.));
#32125=CARTESIAN_POINT('Ctrl Pts',(20.0722879610899,-13.1048196144678,0.));
#32126=CARTESIAN_POINT('Ctrl Pts',(20.0837475345526,-13.1393715591102,0.));
#32127=CARTESIAN_POINT('',(20.0837475345525,-13.1393715591102,15.));
#32128=CARTESIAN_POINT('Ctrl Pts',(20.0837475345526,-13.1393715591102,15.));
#32129=CARTESIAN_POINT('Ctrl Pts',(20.0780177478283,-13.1220955868173,15.));
#32130=CARTESIAN_POINT('Ctrl Pts',(20.0665110891946,-13.0875783330728,15.));
#32131=CARTESIAN_POINT('Ctrl Pts',(20.0491098457044,-13.0359065249991,15.));
#32132=CARTESIAN_POINT('Ctrl Pts',(20.0256255826397,-12.9672189949731,15.));
#32133=CARTESIAN_POINT('Ctrl Pts',(19.9957986945787,-12.8817072534696,15.));
#32134=CARTESIAN_POINT('Ctrl Pts',(19.9654995335894,-12.7965444294443,15.));
#32135=CARTESIAN_POINT('Ctrl Pts',(19.9347273847264,-12.7117325003719,15.));
#32136=CARTESIAN_POINT('Ctrl Pts',(19.9034816813503,-12.6272742843372,15.));
#32137=CARTESIAN_POINT('Ctrl Pts',(19.8717621942733,-12.5431736030596,15.));
#32138=CARTESIAN_POINT('Ctrl Pts',(19.839568972011,-12.4594350764989,15.));
#32139=CARTESIAN_POINT('Ctrl Pts',(19.8069022248387,-12.3760638341708,15.));
#32140=CARTESIAN_POINT('Ctrl Pts',(19.7737622285562,-12.2930652417987,15.));
#32141=CARTESIAN_POINT('Ctrl Pts',(19.7401492304335,-12.2104446447874,15.));
#32142=CARTESIAN_POINT('Ctrl Pts',(19.7060633406705,-12.1282070378972,15.));
#32143=CARTESIAN_POINT('Ctrl Pts',(19.6715045149944,-12.0463570680309,15.));
#32144=CARTESIAN_POINT('Ctrl Pts',(19.6364725931695,-11.9648992312094,15.));
#32145=CARTESIAN_POINT('Ctrl Pts',(19.6009673241771,-11.8838380136222,15.));
#32146=CARTESIAN_POINT('Ctrl Pts',(19.5649883985826,-11.8031780389346,15.));
#32147=CARTESIAN_POINT('Ctrl Pts',(19.5285354853626,-11.722924244195,15.));
#32148=CARTESIAN_POINT('Ctrl Pts',(19.4916082541529,-11.6430819099846,15.));
#32149=CARTESIAN_POINT('Ctrl Pts',(19.4542063779876,-11.5636565297382,15.));
#32150=CARTESIAN_POINT('Ctrl Pts',(19.4163295466324,-11.4846537135043,15.));
#32151=CARTESIAN_POINT('Ctrl Pts',(19.3779774742875,-11.4060790880015,15.));
#32152=CARTESIAN_POINT('Ctrl Pts',(19.3391499248083,-11.3279381634523,15.));
#32153=CARTESIAN_POINT('Ctrl Pts',(19.2998466936739,-11.2502363198588,15.));
#32154=CARTESIAN_POINT('Ctrl Pts',(19.2600675167206,-11.1729790050543,15.));
#32155=CARTESIAN_POINT('Ctrl Pts',(19.2198119937835,-11.0961718903994,15.));
#32156=CARTESIAN_POINT('Ctrl Pts',(19.1790795192393,-11.0198210228993,15.));
#32157=CARTESIAN_POINT('Ctrl Pts',(19.1378691901023,-10.9439330179206,15.));
#32158=CARTESIAN_POINT('Ctrl Pts',(19.0961797996403,-10.868515097783,15.));
#32159=CARTESIAN_POINT('Ctrl Pts',(19.0540100416943,-10.7935747414879,15.));
#32160=CARTESIAN_POINT('Ctrl Pts',(19.0113586878152,-10.7191193896586,15.));
#32161=CARTESIAN_POINT('Ctrl Pts',(18.9682247574834,-10.6451561585969,15.));
#32162=CARTESIAN_POINT('Ctrl Pts',(18.9246077453188,-10.5716914651544,15.));
#32163=CARTESIAN_POINT('Ctrl Pts',(18.8805076729356,-10.4987309368494,15.));
#32164=CARTESIAN_POINT('Ctrl Pts',(18.8359245594214,-10.4262802670211,15.));
#32165=CARTESIAN_POINT('Ctrl Pts',(18.7908579693851,-10.3543459451258,15.));
#32166=CARTESIAN_POINT('Ctrl Pts',(18.7453065790062,-10.2829359603685,15.));
#32167=CARTESIAN_POINT('Ctrl Pts',(18.699267629819,-10.2120606864872,15.));
#32168=CARTESIAN_POINT('Ctrl Pts',(18.6527367592664,-10.1417331637795,15.));
#32169=CARTESIAN_POINT('Ctrl Pts',(18.605709190442,-10.0719672018851,15.));
#32170=CARTESIAN_POINT('Ctrl Pts',(18.5581807679204,-10.0027757313807,15.));
#32171=CARTESIAN_POINT('Ctrl Pts',(18.5101489409161,-9.93416923996829,15.));
#32172=CARTESIAN_POINT('Ctrl Pts',(18.461614050347,-9.86615372541685,15.));
#32173=CARTESIAN_POINT('Ctrl Pts',(18.4125796444662,-9.79873019947434,15.));
#32174=CARTESIAN_POINT('Ctrl Pts',(18.3630495772677,-9.73189932619939,15.));
#32175=CARTESIAN_POINT('Ctrl Pts',(18.3130254811852,-9.6656654640326,15.));
#32176=CARTESIAN_POINT('Ctrl Pts',(18.2625044208165,-9.60004042085347,15.));
#32177=CARTESIAN_POINT('Ctrl Pts',(18.2114756946126,-9.53504856811686,15.));
#32178=CARTESIAN_POINT('Ctrl Pts',(18.1599204445014,-9.47072748065832,15.));
#32179=CARTESIAN_POINT('Ctrl Pts',(18.1078184146735,-9.40711718355464,15.));
#32180=CARTESIAN_POINT('Ctrl Pts',(18.0551538338035,-9.34425079614396,15.));
#32181=CARTESIAN_POINT('Ctrl Pts',(18.0019206847747,-9.28214615574471,15.));
#32182=CARTESIAN_POINT('Ctrl Pts',(17.9481305624284,-9.22079331175917,15.));
#32183=CARTESIAN_POINT('Ctrl Pts',(17.8938116696237,-9.1601561636161,15.));
#32184=CARTESIAN_POINT('Ctrl Pts',(17.8389924349283,-9.10019864472208,15.));
#32185=CARTESIAN_POINT('Ctrl Pts',(17.7836872744016,-9.04090748239097,15.));
#32186=CARTESIAN_POINT('Ctrl Pts',(17.7278841963319,-8.98231202490686,15.));
#32187=CARTESIAN_POINT('Ctrl Pts',(17.6715250120654,-8.92451585185175,15.));
#32188=CARTESIAN_POINT('Ctrl Pts',(17.614513388992,-8.86768402115344,15.));
#32189=CARTESIAN_POINT('Ctrl Pts',(17.5567525798882,-8.81198307239551,15.));
#32190=CARTESIAN_POINT('Ctrl Pts',(17.4981785296199,-8.75752832625955,15.));
#32191=CARTESIAN_POINT('Ctrl Pts',(17.438788019753,-8.70433925112174,15.));
#32192=CARTESIAN_POINT('Ctrl Pts',(17.3786861166843,-8.65226368112816,15.));
#32193=CARTESIAN_POINT('Ctrl Pts',(17.3180459442745,-8.60104338529165,15.));
#32194=CARTESIAN_POINT('Ctrl Pts',(17.2570167183611,-8.55046295192434,15.));
#32195=CARTESIAN_POINT('Ctrl Pts',(17.1956428575086,-8.50048099003883,15.));
#32196=CARTESIAN_POINT('Ctrl Pts',(17.1337886602855,-8.45135198307877,15.));
#32197=CARTESIAN_POINT('Ctrl Pts',(17.071033847921,-8.40379607744266,15.));
#32198=CARTESIAN_POINT('Ctrl Pts',(17.0067806259695,-8.35882146841244,15.));
#32199=CARTESIAN_POINT('Ctrl Pts',(16.9536879065132,-8.32573081382563,15.));
#32200=CARTESIAN_POINT('Ctrl Pts',(16.9126979078877,-8.30290517019115,15.));
#32201=CARTESIAN_POINT('Ctrl Pts',(16.8848228151885,-8.28862062120315,15.));
#32202=CARTESIAN_POINT('Ctrl Pts',(16.8707481591095,-8.28171148831561,15.));
#32203=CARTESIAN_POINT('',(20.0837475345525,-13.1393715591102,0.));
#32204=CARTESIAN_POINT('Origin',(9.33709008296438E-14,-6.79236997764462E-14,
0.));
#32205=CARTESIAN_POINT('',(18.7025042402277,-15.0404898571911,0.));
#32206=CARTESIAN_POINT('Origin',(9.33709008296438E-14,-6.79236997764462E-14,
0.));
#32207=CARTESIAN_POINT('',(18.7025042402277,-15.0404898571911,15.));
#32208=CARTESIAN_POINT('Origin',(9.33709008296438E-14,-6.79236997764462E-14,
15.));
#32209=CARTESIAN_POINT('',(18.7025042402277,-15.0404898571911,0.));
#32210=CARTESIAN_POINT('Ctrl Pts',(13.0897235660237,-13.4858453790958,0.));
#32211=CARTESIAN_POINT('Ctrl Pts',(13.0897235660237,-13.4858453790958,18.));
#32212=CARTESIAN_POINT('Ctrl Pts',(13.1006438497967,-13.4970961329957,0.));
#32213=CARTESIAN_POINT('Ctrl Pts',(13.1006438497967,-13.4970961329957,18.));
#32214=CARTESIAN_POINT('Ctrl Pts',(13.1228431405579,-13.5191927531554,0.));
#32215=CARTESIAN_POINT('Ctrl Pts',(13.1228431405579,-13.5191927531554,18.));
#32216=CARTESIAN_POINT('Ctrl Pts',(13.1572182238498,-13.5511230466604,0.));
#32217=CARTESIAN_POINT('Ctrl Pts',(13.1572182238498,-13.5511230466604,18.));
#32218=CARTESIAN_POINT('Ctrl Pts',(13.2050958591127,-13.5913916488449,0.));
#32219=CARTESIAN_POINT('Ctrl Pts',(13.2050958591127,-13.5913916488449,18.));
#32220=CARTESIAN_POINT('Ctrl Pts',(13.267724591625,-13.6386021757691,0.));
#32221=CARTESIAN_POINT('Ctrl Pts',(13.267724591625,-13.6386021757691,18.));
#32222=CARTESIAN_POINT('Ctrl Pts',(13.332345249068,-13.6835899659728,0.));
#32223=CARTESIAN_POINT('Ctrl Pts',(13.332345249068,-13.6835899659728,18.));
#32224=CARTESIAN_POINT('Ctrl Pts',(13.3981837093918,-13.7272351052346,0.));
#32225=CARTESIAN_POINT('Ctrl Pts',(13.3981837093918,-13.7272351052346,18.));
#32226=CARTESIAN_POINT('Ctrl Pts',(13.4646849459541,-13.7701598398937,0.));
#32227=CARTESIAN_POINT('Ctrl Pts',(13.4646849459541,-13.7701598398937,18.));
#32228=CARTESIAN_POINT('Ctrl Pts',(13.5316488646659,-13.8125718693898,0.));
#32229=CARTESIAN_POINT('Ctrl Pts',(13.5316488646659,-13.8125718693898,18.));
#32230=CARTESIAN_POINT('Ctrl Pts',(13.5991011046042,-13.854416158639,0.));
#32231=CARTESIAN_POINT('Ctrl Pts',(13.5991011046042,-13.854416158639,18.));
#32232=CARTESIAN_POINT('Ctrl Pts',(13.6672004242289,-13.8954842290745,0.));
#32233=CARTESIAN_POINT('Ctrl Pts',(13.6672004242289,-13.8954842290745,18.));
#32234=CARTESIAN_POINT('Ctrl Pts',(13.7361389175879,-13.9355316323567,0.));
#32235=CARTESIAN_POINT('Ctrl Pts',(13.7361389175879,-13.9355316323567,18.));
#32236=CARTESIAN_POINT('Ctrl Pts',(13.806028835706,-13.9744114225699,0.));
#32237=CARTESIAN_POINT('Ctrl Pts',(13.806028835706,-13.9744114225699,18.));
#32238=CARTESIAN_POINT('Ctrl Pts',(13.876852657608,-14.0121326766855,0.));
#32239=CARTESIAN_POINT('Ctrl Pts',(13.876852657608,-14.0121326766855,18.));
#32240=CARTESIAN_POINT('Ctrl Pts',(13.9485205009332,-14.0487919508068,0.));
#32241=CARTESIAN_POINT('Ctrl Pts',(13.9485205009332,-14.0487919508068,18.));
#32242=CARTESIAN_POINT('Ctrl Pts',(14.0209038736616,-14.0845327205726,0.));
#32243=CARTESIAN_POINT('Ctrl Pts',(14.0209038736616,-14.0845327205726,18.));
#32244=CARTESIAN_POINT('Ctrl Pts',(14.0938755647891,-14.1194976094444,0.));
#32245=CARTESIAN_POINT('Ctrl Pts',(14.0938755647891,-14.1194976094444,18.));
#32246=CARTESIAN_POINT('Ctrl Pts',(14.1673550455622,-14.1537739659715,0.));
#32247=CARTESIAN_POINT('Ctrl Pts',(14.1673550455622,-14.1537739659715,18.));
#32248=CARTESIAN_POINT('Ctrl Pts',(14.2413181097468,-14.1873822640681,0.));
#32249=CARTESIAN_POINT('Ctrl Pts',(14.2413181097468,-14.1873822640681,18.));
#32250=CARTESIAN_POINT('Ctrl Pts',(14.3157729256101,-14.2203046917613,0.));
#32251=CARTESIAN_POINT('Ctrl Pts',(14.3157729256101,-14.2203046917613,18.));
#32252=CARTESIAN_POINT('Ctrl Pts',(14.3907450096103,-14.2525030666863,0.));
#32253=CARTESIAN_POINT('Ctrl Pts',(14.3907450096103,-14.2525030666863,18.));
#32254=CARTESIAN_POINT('Ctrl Pts',(14.4662599802681,-14.2839394106401,0.));
#32255=CARTESIAN_POINT('Ctrl Pts',(14.4662599802681,-14.2839394106401,18.));
#32256=CARTESIAN_POINT('Ctrl Pts',(14.5423237181615,-14.3145996213697,0.));
#32257=CARTESIAN_POINT('Ctrl Pts',(14.5423237181615,-14.3145996213697,18.));
#32258=CARTESIAN_POINT('Ctrl Pts',(14.6189211183837,-14.3444949335274,0.));
#32259=CARTESIAN_POINT('Ctrl Pts',(14.6189211183837,-14.3444949335274,18.));
#32260=CARTESIAN_POINT('Ctrl Pts',(14.6960255561799,-14.3736505809735,0.));
#32261=CARTESIAN_POINT('Ctrl Pts',(14.6960255561799,-14.3736505809735,18.));
#32262=CARTESIAN_POINT('Ctrl Pts',(14.7736052248294,-14.4020981965564,0.));
#32263=CARTESIAN_POINT('Ctrl Pts',(14.7736052248294,-14.4020981965564,18.));
#32264=CARTESIAN_POINT('Ctrl Pts',(14.8516302160049,-14.4298673266313,0.));
#32265=CARTESIAN_POINT('Ctrl Pts',(14.8516302160049,-14.4298673266313,18.));
#32266=CARTESIAN_POINT('Ctrl Pts',(14.9300806580357,-14.4569756801697,0.));
#32267=CARTESIAN_POINT('Ctrl Pts',(14.9300806580357,-14.4569756801697,18.));
#32268=CARTESIAN_POINT('Ctrl Pts',(15.0089462280504,-14.4834296977405,0.));
#32269=CARTESIAN_POINT('Ctrl Pts',(15.0089462280504,-14.4834296977405,18.));
#32270=CARTESIAN_POINT('Ctrl Pts',(15.0882222764759,-14.5092291736391,0.));
#32271=CARTESIAN_POINT('Ctrl Pts',(15.0882222764759,-14.5092291736391,18.));
#32272=CARTESIAN_POINT('Ctrl Pts',(15.1679069808052,-14.5343706477051,0.));
#32273=CARTESIAN_POINT('Ctrl Pts',(15.1679069808052,-14.5343706477051,18.));
#32274=CARTESIAN_POINT('Ctrl Pts',(15.2479982823383,-14.5588510579962,0.));
#32275=CARTESIAN_POINT('Ctrl Pts',(15.2479982823383,-14.5588510579962,18.));
#32276=CARTESIAN_POINT('Ctrl Pts',(15.3284903715086,-14.5826719336929,0.));
#32277=CARTESIAN_POINT('Ctrl Pts',(15.3284903715086,-14.5826719336929,18.));
#32278=CARTESIAN_POINT('Ctrl Pts',(15.4093740621547,-14.6058389416146,0.));
#32279=CARTESIAN_POINT('Ctrl Pts',(15.4093740621547,-14.6058389416146,18.));
#32280=CARTESIAN_POINT('Ctrl Pts',(15.4906383406647,-14.6283600295736,0.));
#32281=CARTESIAN_POINT('Ctrl Pts',(15.4906383406647,-14.6283600295736,18.));
#32282=CARTESIAN_POINT('Ctrl Pts',(15.5722715494357,-14.6502440080912,0.));
#32283=CARTESIAN_POINT('Ctrl Pts',(15.5722715494357,-14.6502440080912,18.));
#32284=CARTESIAN_POINT('Ctrl Pts',(15.6542626345121,-14.6714990558793,0.));
#32285=CARTESIAN_POINT('Ctrl Pts',(15.6542626345121,-14.6714990558793,18.));
#32286=CARTESIAN_POINT('Ctrl Pts',(15.7366025822956,-14.692131002056,0.));
#32287=CARTESIAN_POINT('Ctrl Pts',(15.7366025822956,-14.692131002056,18.));
#32288=CARTESIAN_POINT('Ctrl Pts',(15.8192842036838,-14.7121435744495,0.));
#32289=CARTESIAN_POINT('Ctrl Pts',(15.8192842036838,-14.7121435744495,18.));
#32290=CARTESIAN_POINT('Ctrl Pts',(15.9023014613802,-14.7315391924939,0.));
#32291=CARTESIAN_POINT('Ctrl Pts',(15.9023014613802,-14.7315391924939,18.));
#32292=CARTESIAN_POINT('Ctrl Pts',(15.9856489347991,-14.7503195973741,0.));
#32293=CARTESIAN_POINT('Ctrl Pts',(15.9856489347991,-14.7503195973741,18.));
#32294=CARTESIAN_POINT('Ctrl Pts',(16.0693212651732,-14.7684865075326,0.));
#32295=CARTESIAN_POINT('Ctrl Pts',(16.0693212651732,-14.7684865075326,18.));
#32296=CARTESIAN_POINT('Ctrl Pts',(16.1533125058853,-14.7860423865308,0.));
#32297=CARTESIAN_POINT('Ctrl Pts',(16.1533125058853,-14.7860423865308,18.));
#32298=CARTESIAN_POINT('Ctrl Pts',(16.2376161919272,-14.8029903659562,0.));
#32299=CARTESIAN_POINT('Ctrl Pts',(16.2376161919272,-14.8029903659562,18.));
#32300=CARTESIAN_POINT('Ctrl Pts',(16.3222256264574,-14.8193339134125,0.));
#32301=CARTESIAN_POINT('Ctrl Pts',(16.3222256264574,-14.8193339134125,18.));
#32302=CARTESIAN_POINT('Ctrl Pts',(16.4071341001481,-14.8350765822692,0.));
#32303=CARTESIAN_POINT('Ctrl Pts',(16.4071341001481,-14.8350765822692,18.));
#32304=CARTESIAN_POINT('Ctrl Pts',(16.492335117066,-14.8502217520165,0.));
#32305=CARTESIAN_POINT('Ctrl Pts',(16.492335117066,-14.8502217520165,18.));
#32306=CARTESIAN_POINT('Ctrl Pts',(16.5778226646614,-14.8647723257055,0.));
#32307=CARTESIAN_POINT('Ctrl Pts',(16.5778226646614,-14.8647723257055,18.));
#32308=CARTESIAN_POINT('Ctrl Pts',(16.6635911790385,-14.8787307479454,0.));
#32309=CARTESIAN_POINT('Ctrl Pts',(16.6635911790385,-14.8787307479454,18.));
#32310=CARTESIAN_POINT('Ctrl Pts',(16.7496353900706,-14.8920991518626,0.));
#32311=CARTESIAN_POINT('Ctrl Pts',(16.7496353900706,-14.8920991518626,18.));
#32312=CARTESIAN_POINT('Ctrl Pts',(16.8359501981915,-14.9048794721647,0.));
#32313=CARTESIAN_POINT('Ctrl Pts',(16.8359501981915,-14.9048794721647,18.));
#32314=CARTESIAN_POINT('Ctrl Pts',(16.9225305499155,-14.9170735658747,0.));
#32315=CARTESIAN_POINT('Ctrl Pts',(16.9225305499155,-14.9170735658747,18.));
#32316=CARTESIAN_POINT('Ctrl Pts',(17.0093712776822,-14.9286833603319,0.));
#32317=CARTESIAN_POINT('Ctrl Pts',(17.0093712776822,-14.9286833603319,18.));
#32318=CARTESIAN_POINT('Ctrl Pts',(17.0964671184813,-14.9397108660998,0.));
#32319=CARTESIAN_POINT('Ctrl Pts',(17.0964671184813,-14.9397108660998,18.));
#32320=CARTESIAN_POINT('Ctrl Pts',(17.1838128327073,-14.9501581118289,0.));
#32321=CARTESIAN_POINT('Ctrl Pts',(17.1838128327073,-14.9501581118289,18.));
#32322=CARTESIAN_POINT('Ctrl Pts',(17.2714032968314,-14.9600271060471,0.));
#32323=CARTESIAN_POINT('Ctrl Pts',(17.2714032968314,-14.9600271060471,18.));
#32324=CARTESIAN_POINT('Ctrl Pts',(17.3592335908102,-14.9693197947387,0.));
#32325=CARTESIAN_POINT('Ctrl Pts',(17.3592335908102,-14.9693197947387,18.));
#32326=CARTESIAN_POINT('Ctrl Pts',(17.4472991215239,-14.9780380183576,0.));
#32327=CARTESIAN_POINT('Ctrl Pts',(17.4472991215239,-14.9780380183576,18.));
#32328=CARTESIAN_POINT('Ctrl Pts',(17.5355955872257,-14.9861834999847,0.));
#32329=CARTESIAN_POINT('Ctrl Pts',(17.5355955872257,-14.9861834999847,18.));
#32330=CARTESIAN_POINT('Ctrl Pts',(17.6241187988652,-14.9937578646616,0.));
#32331=CARTESIAN_POINT('Ctrl Pts',(17.6241187988652,-14.9937578646616,18.));
#32332=CARTESIAN_POINT('Ctrl Pts',(17.7128645299878,-15.0007626541287,0.));
#32333=CARTESIAN_POINT('Ctrl Pts',(17.7128645299878,-15.0007626541287,18.));
#32334=CARTESIAN_POINT('Ctrl Pts',(17.8018283748074,-15.0071993464636,0.));
#32335=CARTESIAN_POINT('Ctrl Pts',(17.8018283748074,-15.0071993464636,18.));
#32336=CARTESIAN_POINT('Ctrl Pts',(17.891005548971,-15.0130693803259,0.));
#32337=CARTESIAN_POINT('Ctrl Pts',(17.891005548971,-15.0130693803259,18.));
#32338=CARTESIAN_POINT('Ctrl Pts',(17.980390892286,-15.0183741723687,0.));
#32339=CARTESIAN_POINT('Ctrl Pts',(17.980390892286,-15.0183741723687,18.));
#32340=CARTESIAN_POINT('Ctrl Pts',(18.0699792164192,-15.0231151183906,0.));
#32341=CARTESIAN_POINT('Ctrl Pts',(18.0699792164192,-15.0231151183906,18.));
#32342=CARTESIAN_POINT('Ctrl Pts',(18.1597655779328,-15.0272936035154,0.));
#32343=CARTESIAN_POINT('Ctrl Pts',(18.1597655779328,-15.0272936035154,18.));
#32344=CARTESIAN_POINT('Ctrl Pts',(18.2497455679917,-15.0309110092482,0.));
#32345=CARTESIAN_POINT('Ctrl Pts',(18.2497455679917,-15.0309110092482,18.));
#32346=CARTESIAN_POINT('Ctrl Pts',(18.3399156227477,-15.0339687345357,0.));
#32347=CARTESIAN_POINT('Ctrl Pts',(18.3399156227477,-15.0339687345357,18.));
#32348=CARTESIAN_POINT('Ctrl Pts',(18.430273237144,-15.0364681891201,0.));
#32349=CARTESIAN_POINT('Ctrl Pts',(18.430273237144,-15.0364681891201,18.));
#32350=CARTESIAN_POINT('Ctrl Pts',(18.5208167514208,-15.0384106640282,0.));
#32351=CARTESIAN_POINT('Ctrl Pts',(18.5208167514208,-15.0384106640282,18.));
#32352=CARTESIAN_POINT('Ctrl Pts',(18.5933995108277,-15.0395199113665,0.));
#32353=CARTESIAN_POINT('Ctrl Pts',(18.5933995108277,-15.0395199113665,18.));
#32354=CARTESIAN_POINT('Ctrl Pts',(18.6479196005666,-15.0401020105546,0.));
#32355=CARTESIAN_POINT('Ctrl Pts',(18.6479196005666,-15.0401020105546,18.));
#32356=CARTESIAN_POINT('Ctrl Pts',(18.6843032127312,-15.0403790752228,0.));
#32357=CARTESIAN_POINT('Ctrl Pts',(18.6843032127312,-15.0403790752228,18.));
#32358=CARTESIAN_POINT('Ctrl Pts',(18.7025042402277,-15.0404898571911,0.));
#32359=CARTESIAN_POINT('Ctrl Pts',(18.7025042402277,-15.0404898571911,18.));
#32360=CARTESIAN_POINT('Ctrl Pts',(13.0897235660237,-13.4858453790958,0.));
#32361=CARTESIAN_POINT('Ctrl Pts',(13.1006438497967,-13.4970961329957,0.));
#32362=CARTESIAN_POINT('Ctrl Pts',(13.1228431405579,-13.5191927531554,0.));
#32363=CARTESIAN_POINT('Ctrl Pts',(13.1572182238498,-13.5511230466604,0.));
#32364=CARTESIAN_POINT('Ctrl Pts',(13.2050958591127,-13.5913916488449,0.));
#32365=CARTESIAN_POINT('Ctrl Pts',(13.267724591625,-13.6386021757691,0.));
#32366=CARTESIAN_POINT('Ctrl Pts',(13.332345249068,-13.6835899659728,0.));
#32367=CARTESIAN_POINT('Ctrl Pts',(13.3981837093918,-13.7272351052346,0.));
#32368=CARTESIAN_POINT('Ctrl Pts',(13.4646849459541,-13.7701598398937,0.));
#32369=CARTESIAN_POINT('Ctrl Pts',(13.5316488646659,-13.8125718693898,0.));
#32370=CARTESIAN_POINT('Ctrl Pts',(13.5991011046042,-13.854416158639,0.));
#32371=CARTESIAN_POINT('Ctrl Pts',(13.6672004242289,-13.8954842290745,0.));
#32372=CARTESIAN_POINT('Ctrl Pts',(13.7361389175879,-13.9355316323567,0.));
#32373=CARTESIAN_POINT('Ctrl Pts',(13.806028835706,-13.9744114225699,0.));
#32374=CARTESIAN_POINT('Ctrl Pts',(13.876852657608,-14.0121326766855,0.));
#32375=CARTESIAN_POINT('Ctrl Pts',(13.9485205009332,-14.0487919508068,0.));
#32376=CARTESIAN_POINT('Ctrl Pts',(14.0209038736616,-14.0845327205726,0.));
#32377=CARTESIAN_POINT('Ctrl Pts',(14.0938755647891,-14.1194976094444,0.));
#32378=CARTESIAN_POINT('Ctrl Pts',(14.1673550455622,-14.1537739659715,0.));
#32379=CARTESIAN_POINT('Ctrl Pts',(14.2413181097468,-14.1873822640681,0.));
#32380=CARTESIAN_POINT('Ctrl Pts',(14.3157729256101,-14.2203046917613,0.));
#32381=CARTESIAN_POINT('Ctrl Pts',(14.3907450096103,-14.2525030666863,0.));
#32382=CARTESIAN_POINT('Ctrl Pts',(14.4662599802681,-14.2839394106401,0.));
#32383=CARTESIAN_POINT('Ctrl Pts',(14.5423237181615,-14.3145996213697,0.));
#32384=CARTESIAN_POINT('Ctrl Pts',(14.6189211183837,-14.3444949335274,0.));
#32385=CARTESIAN_POINT('Ctrl Pts',(14.6960255561799,-14.3736505809735,0.));
#32386=CARTESIAN_POINT('Ctrl Pts',(14.7736052248294,-14.4020981965564,0.));
#32387=CARTESIAN_POINT('Ctrl Pts',(14.8516302160049,-14.4298673266313,0.));
#32388=CARTESIAN_POINT('Ctrl Pts',(14.9300806580357,-14.4569756801697,0.));
#32389=CARTESIAN_POINT('Ctrl Pts',(15.0089462280504,-14.4834296977405,0.));
#32390=CARTESIAN_POINT('Ctrl Pts',(15.0882222764759,-14.5092291736391,0.));
#32391=CARTESIAN_POINT('Ctrl Pts',(15.1679069808052,-14.5343706477051,0.));
#32392=CARTESIAN_POINT('Ctrl Pts',(15.2479982823383,-14.5588510579962,0.));
#32393=CARTESIAN_POINT('Ctrl Pts',(15.3284903715086,-14.5826719336929,0.));
#32394=CARTESIAN_POINT('Ctrl Pts',(15.4093740621547,-14.6058389416146,0.));
#32395=CARTESIAN_POINT('Ctrl Pts',(15.4906383406647,-14.6283600295736,0.));
#32396=CARTESIAN_POINT('Ctrl Pts',(15.5722715494357,-14.6502440080912,0.));
#32397=CARTESIAN_POINT('Ctrl Pts',(15.6542626345121,-14.6714990558793,0.));
#32398=CARTESIAN_POINT('Ctrl Pts',(15.7366025822956,-14.692131002056,0.));
#32399=CARTESIAN_POINT('Ctrl Pts',(15.8192842036838,-14.7121435744495,0.));
#32400=CARTESIAN_POINT('Ctrl Pts',(15.9023014613802,-14.7315391924939,0.));
#32401=CARTESIAN_POINT('Ctrl Pts',(15.9856489347991,-14.7503195973741,0.));
#32402=CARTESIAN_POINT('Ctrl Pts',(16.0693212651732,-14.7684865075326,0.));
#32403=CARTESIAN_POINT('Ctrl Pts',(16.1533125058853,-14.7860423865308,0.));
#32404=CARTESIAN_POINT('Ctrl Pts',(16.2376161919272,-14.8029903659562,0.));
#32405=CARTESIAN_POINT('Ctrl Pts',(16.3222256264574,-14.8193339134125,0.));
#32406=CARTESIAN_POINT('Ctrl Pts',(16.4071341001481,-14.8350765822692,0.));
#32407=CARTESIAN_POINT('Ctrl Pts',(16.492335117066,-14.8502217520165,0.));
#32408=CARTESIAN_POINT('Ctrl Pts',(16.5778226646614,-14.8647723257055,0.));
#32409=CARTESIAN_POINT('Ctrl Pts',(16.6635911790385,-14.8787307479454,0.));
#32410=CARTESIAN_POINT('Ctrl Pts',(16.7496353900706,-14.8920991518626,0.));
#32411=CARTESIAN_POINT('Ctrl Pts',(16.8359501981915,-14.9048794721647,0.));
#32412=CARTESIAN_POINT('Ctrl Pts',(16.9225305499155,-14.9170735658747,0.));
#32413=CARTESIAN_POINT('Ctrl Pts',(17.0093712776822,-14.9286833603319,0.));
#32414=CARTESIAN_POINT('Ctrl Pts',(17.0964671184813,-14.9397108660998,0.));
#32415=CARTESIAN_POINT('Ctrl Pts',(17.1838128327073,-14.9501581118289,0.));
#32416=CARTESIAN_POINT('Ctrl Pts',(17.2714032968314,-14.9600271060471,0.));
#32417=CARTESIAN_POINT('Ctrl Pts',(17.3592335908102,-14.9693197947387,0.));
#32418=CARTESIAN_POINT('Ctrl Pts',(17.4472991215239,-14.9780380183576,0.));
#32419=CARTESIAN_POINT('Ctrl Pts',(17.5355955872257,-14.9861834999847,0.));
#32420=CARTESIAN_POINT('Ctrl Pts',(17.6241187988652,-14.9937578646616,0.));
#32421=CARTESIAN_POINT('Ctrl Pts',(17.7128645299878,-15.0007626541287,0.));
#32422=CARTESIAN_POINT('Ctrl Pts',(17.8018283748074,-15.0071993464636,0.));
#32423=CARTESIAN_POINT('Ctrl Pts',(17.891005548971,-15.0130693803259,0.));
#32424=CARTESIAN_POINT('Ctrl Pts',(17.980390892286,-15.0183741723687,0.));
#32425=CARTESIAN_POINT('Ctrl Pts',(18.0699792164192,-15.0231151183906,0.));
#32426=CARTESIAN_POINT('Ctrl Pts',(18.1597655779328,-15.0272936035154,0.));
#32427=CARTESIAN_POINT('Ctrl Pts',(18.2497455679917,-15.0309110092482,0.));
#32428=CARTESIAN_POINT('Ctrl Pts',(18.3399156227477,-15.0339687345357,0.));
#32429=CARTESIAN_POINT('Ctrl Pts',(18.4483447600233,-15.036968080037,0.));
#32430=CARTESIAN_POINT('Ctrl Pts',(18.5389347492702,-15.038771310026,0.));
#32431=CARTESIAN_POINT('Ctrl Pts',(18.6115544313469,-15.0397694451467,0.));
#32432=CARTESIAN_POINT('Ctrl Pts',(18.6661021851765,-15.0402682932586,0.));
#32433=CARTESIAN_POINT('Ctrl Pts',(18.7025042402277,-15.0404898571911,0.));
#32434=CARTESIAN_POINT('Ctrl Pts',(13.0897235660237,-13.4858453790958,15.));
#32435=CARTESIAN_POINT('Ctrl Pts',(13.1006438497967,-13.4970961329957,15.));
#32436=CARTESIAN_POINT('Ctrl Pts',(13.1228431405579,-13.5191927531554,15.));
#32437=CARTESIAN_POINT('Ctrl Pts',(13.1572182238498,-13.5511230466604,15.));
#32438=CARTESIAN_POINT('Ctrl Pts',(13.2050958591127,-13.5913916488449,15.));
#32439=CARTESIAN_POINT('Ctrl Pts',(13.267724591625,-13.6386021757691,15.));
#32440=CARTESIAN_POINT('Ctrl Pts',(13.332345249068,-13.6835899659728,15.));
#32441=CARTESIAN_POINT('Ctrl Pts',(13.3981837093918,-13.7272351052346,15.));
#32442=CARTESIAN_POINT('Ctrl Pts',(13.4646849459541,-13.7701598398937,15.));
#32443=CARTESIAN_POINT('Ctrl Pts',(13.5316488646659,-13.8125718693898,15.));
#32444=CARTESIAN_POINT('Ctrl Pts',(13.5991011046042,-13.854416158639,15.));
#32445=CARTESIAN_POINT('Ctrl Pts',(13.6672004242289,-13.8954842290745,15.));
#32446=CARTESIAN_POINT('Ctrl Pts',(13.7361389175879,-13.9355316323567,15.));
#32447=CARTESIAN_POINT('Ctrl Pts',(13.806028835706,-13.9744114225699,15.));
#32448=CARTESIAN_POINT('Ctrl Pts',(13.876852657608,-14.0121326766855,15.));
#32449=CARTESIAN_POINT('Ctrl Pts',(13.9485205009332,-14.0487919508068,15.));
#32450=CARTESIAN_POINT('Ctrl Pts',(14.0209038736616,-14.0845327205726,15.));
#32451=CARTESIAN_POINT('Ctrl Pts',(14.0938755647891,-14.1194976094444,15.));
#32452=CARTESIAN_POINT('Ctrl Pts',(14.1673550455622,-14.1537739659715,15.));
#32453=CARTESIAN_POINT('Ctrl Pts',(14.2413181097468,-14.1873822640681,15.));
#32454=CARTESIAN_POINT('Ctrl Pts',(14.3157729256101,-14.2203046917613,15.));
#32455=CARTESIAN_POINT('Ctrl Pts',(14.3907450096103,-14.2525030666863,15.));
#32456=CARTESIAN_POINT('Ctrl Pts',(14.4662599802681,-14.2839394106401,15.));
#32457=CARTESIAN_POINT('Ctrl Pts',(14.5423237181615,-14.3145996213697,15.));
#32458=CARTESIAN_POINT('Ctrl Pts',(14.6189211183837,-14.3444949335274,15.));
#32459=CARTESIAN_POINT('Ctrl Pts',(14.6960255561799,-14.3736505809735,15.));
#32460=CARTESIAN_POINT('Ctrl Pts',(14.7736052248294,-14.4020981965564,15.));
#32461=CARTESIAN_POINT('Ctrl Pts',(14.8516302160049,-14.4298673266313,15.));
#32462=CARTESIAN_POINT('Ctrl Pts',(14.9300806580357,-14.4569756801697,15.));
#32463=CARTESIAN_POINT('Ctrl Pts',(15.0089462280504,-14.4834296977405,15.));
#32464=CARTESIAN_POINT('Ctrl Pts',(15.0882222764759,-14.5092291736391,15.));
#32465=CARTESIAN_POINT('Ctrl Pts',(15.1679069808052,-14.5343706477051,15.));
#32466=CARTESIAN_POINT('Ctrl Pts',(15.2479982823383,-14.5588510579962,15.));
#32467=CARTESIAN_POINT('Ctrl Pts',(15.3284903715086,-14.5826719336929,15.));
#32468=CARTESIAN_POINT('Ctrl Pts',(15.4093740621547,-14.6058389416146,15.));
#32469=CARTESIAN_POINT('Ctrl Pts',(15.4906383406647,-14.6283600295736,15.));
#32470=CARTESIAN_POINT('Ctrl Pts',(15.5722715494357,-14.6502440080912,15.));
#32471=CARTESIAN_POINT('Ctrl Pts',(15.6542626345121,-14.6714990558793,15.));
#32472=CARTESIAN_POINT('Ctrl Pts',(15.7366025822956,-14.692131002056,15.));
#32473=CARTESIAN_POINT('Ctrl Pts',(15.8192842036838,-14.7121435744495,15.));
#32474=CARTESIAN_POINT('Ctrl Pts',(15.9023014613802,-14.7315391924939,15.));
#32475=CARTESIAN_POINT('Ctrl Pts',(15.9856489347991,-14.7503195973741,15.));
#32476=CARTESIAN_POINT('Ctrl Pts',(16.0693212651732,-14.7684865075326,15.));
#32477=CARTESIAN_POINT('Ctrl Pts',(16.1533125058853,-14.7860423865308,15.));
#32478=CARTESIAN_POINT('Ctrl Pts',(16.2376161919272,-14.8029903659562,15.));
#32479=CARTESIAN_POINT('Ctrl Pts',(16.3222256264574,-14.8193339134125,15.));
#32480=CARTESIAN_POINT('Ctrl Pts',(16.4071341001481,-14.8350765822692,15.));
#32481=CARTESIAN_POINT('Ctrl Pts',(16.492335117066,-14.8502217520165,15.));
#32482=CARTESIAN_POINT('Ctrl Pts',(16.5778226646614,-14.8647723257055,15.));
#32483=CARTESIAN_POINT('Ctrl Pts',(16.6635911790385,-14.8787307479454,15.));
#32484=CARTESIAN_POINT('Ctrl Pts',(16.7496353900706,-14.8920991518626,15.));
#32485=CARTESIAN_POINT('Ctrl Pts',(16.8359501981915,-14.9048794721647,15.));
#32486=CARTESIAN_POINT('Ctrl Pts',(16.9225305499155,-14.9170735658747,15.));
#32487=CARTESIAN_POINT('Ctrl Pts',(17.0093712776822,-14.9286833603319,15.));
#32488=CARTESIAN_POINT('Ctrl Pts',(17.0964671184813,-14.9397108660998,15.));
#32489=CARTESIAN_POINT('Ctrl Pts',(17.1838128327073,-14.9501581118289,15.));
#32490=CARTESIAN_POINT('Ctrl Pts',(17.2714032968314,-14.9600271060471,15.));
#32491=CARTESIAN_POINT('Ctrl Pts',(17.3592335908102,-14.9693197947387,15.));
#32492=CARTESIAN_POINT('Ctrl Pts',(17.4472991215239,-14.9780380183576,15.));
#32493=CARTESIAN_POINT('Ctrl Pts',(17.5355955872257,-14.9861834999847,15.));
#32494=CARTESIAN_POINT('Ctrl Pts',(17.6241187988652,-14.9937578646616,15.));
#32495=CARTESIAN_POINT('Ctrl Pts',(17.7128645299878,-15.0007626541287,15.));
#32496=CARTESIAN_POINT('Ctrl Pts',(17.8018283748074,-15.0071993464636,15.));
#32497=CARTESIAN_POINT('Ctrl Pts',(17.891005548971,-15.0130693803259,15.));
#32498=CARTESIAN_POINT('Ctrl Pts',(17.980390892286,-15.0183741723687,15.));
#32499=CARTESIAN_POINT('Ctrl Pts',(18.0699792164192,-15.0231151183906,15.));
#32500=CARTESIAN_POINT('Ctrl Pts',(18.1597655779328,-15.0272936035154,15.));
#32501=CARTESIAN_POINT('Ctrl Pts',(18.2497455679917,-15.0309110092482,15.));
#32502=CARTESIAN_POINT('Ctrl Pts',(18.3399156227477,-15.0339687345357,15.));
#32503=CARTESIAN_POINT('Ctrl Pts',(18.4483447600233,-15.036968080037,15.));
#32504=CARTESIAN_POINT('Ctrl Pts',(18.5389347492702,-15.038771310026,15.));
#32505=CARTESIAN_POINT('Ctrl Pts',(18.6115544313469,-15.0397694451467,15.));
#32506=CARTESIAN_POINT('Ctrl Pts',(18.6661021851765,-15.0402682932586,15.));
#32507=CARTESIAN_POINT('Ctrl Pts',(18.7025042402277,-15.0404898571911,15.));
#32508=CARTESIAN_POINT('Ctrl Pts',(8.52496423935284,-22.4349054983023,0.));
#32509=CARTESIAN_POINT('Ctrl Pts',(8.52496423935284,-22.4349054983023,18.));
#32510=CARTESIAN_POINT('Ctrl Pts',(8.53048330625154,-22.4175610589877,0.));
#32511=CARTESIAN_POINT('Ctrl Pts',(8.53048330625154,-22.4175610589877,18.));
#32512=CARTESIAN_POINT('Ctrl Pts',(8.54146295656906,-22.3828725698612,0.));
#32513=CARTESIAN_POINT('Ctrl Pts',(8.54146295656906,-22.3828725698612,18.));
#32514=CARTESIAN_POINT('Ctrl Pts',(8.55775698160721,-22.3308410047044,0.));
#32515=CARTESIAN_POINT('Ctrl Pts',(8.55775698160721,-22.3308410047044,18.));
#32516=CARTESIAN_POINT('Ctrl Pts',(8.57913133085326,-22.2614679221214,0.));
#32517=CARTESIAN_POINT('Ctrl Pts',(8.57913133085326,-22.2614679221214,18.));
#32518=CARTESIAN_POINT('Ctrl Pts',(8.60526341207613,-22.1747556651024,0.));
#32519=CARTESIAN_POINT('Ctrl Pts',(8.60526341207613,-22.1747556651024,18.));
#32520=CARTESIAN_POINT('Ctrl Pts',(8.63080832792612,-22.0880480931906,0.));
#32521=CARTESIAN_POINT('Ctrl Pts',(8.63080832792612,-22.0880480931906,18.));
#32522=CARTESIAN_POINT('Ctrl Pts',(8.6557643376698,-22.0013463859623,0.));
#32523=CARTESIAN_POINT('Ctrl Pts',(8.6557643376698,-22.0013463859623,18.));
#32524=CARTESIAN_POINT('Ctrl Pts',(8.68012932645739,-21.9146524902336,0.));
#32525=CARTESIAN_POINT('Ctrl Pts',(8.68012932645739,-21.9146524902336,18.));
#32526=CARTESIAN_POINT('Ctrl Pts',(8.70390086252202,-21.8279693631274,0.));
#32527=CARTESIAN_POINT('Ctrl Pts',(8.70390086252202,-21.8279693631274,18.));
#32528=CARTESIAN_POINT('Ctrl Pts',(8.72707626956921,-21.7413007707864,0.));
#32529=CARTESIAN_POINT('Ctrl Pts',(8.72707626956921,-21.7413007707864,18.));
#32530=CARTESIAN_POINT('Ctrl Pts',(8.74965270266163,-21.6546509866725,0.));
#32531=CARTESIAN_POINT('Ctrl Pts',(8.74965270266163,-21.6546509866725,18.));
#32532=CARTESIAN_POINT('Ctrl Pts',(8.77162723103298,-21.5680245138584,0.));
#32533=CARTESIAN_POINT('Ctrl Pts',(8.77162723103298,-21.5680245138584,18.));
#32534=CARTESIAN_POINT('Ctrl Pts',(8.79299691277858,-21.481425822209,0.));
#32535=CARTESIAN_POINT('Ctrl Pts',(8.79299691277858,-21.481425822209,18.));
#32536=CARTESIAN_POINT('Ctrl Pts',(8.81375890120581,-21.3948590173441,0.));
#32537=CARTESIAN_POINT('Ctrl Pts',(8.81375890120581,-21.3948590173441,18.));
#32538=CARTESIAN_POINT('Ctrl Pts',(8.83391042911628,-21.3083278326642,0.));
#32539=CARTESIAN_POINT('Ctrl Pts',(8.83391042911628,-21.3083278326642,18.));
#32540=CARTESIAN_POINT('Ctrl Pts',(8.85344872418155,-21.2218358113425,0.));
#32541=CARTESIAN_POINT('Ctrl Pts',(8.85344872418155,-21.2218358113425,18.));
#32542=CARTESIAN_POINT('Ctrl Pts',(8.87237094640748,-21.1353864352374,0.));
#32543=CARTESIAN_POINT('Ctrl Pts',(8.87237094640748,-21.1353864352374,18.));
#32544=CARTESIAN_POINT('Ctrl Pts',(8.89067412773385,-21.0489832630915,0.));
#32545=CARTESIAN_POINT('Ctrl Pts',(8.89067412773385,-21.0489832630915,18.));
#32546=CARTESIAN_POINT('Ctrl Pts',(8.90835509843284,-20.9626300944902,0.));
#32547=CARTESIAN_POINT('Ctrl Pts',(8.90835509843284,-20.9626300944902,18.));
#32548=CARTESIAN_POINT('Ctrl Pts',(8.92541048738648,-20.8763310073304,0.));
#32549=CARTESIAN_POINT('Ctrl Pts',(8.92541048738648,-20.8763310073304,18.));
#32550=CARTESIAN_POINT('Ctrl Pts',(8.94183680111377,-20.7900902537083,0.));
#32551=CARTESIAN_POINT('Ctrl Pts',(8.94183680111377,-20.7900902537083,18.));
#32552=CARTESIAN_POINT('Ctrl Pts',(8.95763049112623,-20.7039121898975,0.));
#32553=CARTESIAN_POINT('Ctrl Pts',(8.95763049112623,-20.7039121898975,18.));
#32554=CARTESIAN_POINT('Ctrl Pts',(8.97278801890467,-20.6178012000199,0.));
#32555=CARTESIAN_POINT('Ctrl Pts',(8.97278801890467,-20.6178012000199,18.));
#32556=CARTESIAN_POINT('Ctrl Pts',(8.98730595457659,-20.5317616031369,0.));
#32557=CARTESIAN_POINT('Ctrl Pts',(8.98730595457659,-20.5317616031369,18.));
#32558=CARTESIAN_POINT('Ctrl Pts',(9.00118097039516,-20.4457976315472,0.));
#32559=CARTESIAN_POINT('Ctrl Pts',(9.00118097039516,-20.4457976315472,18.));
#32560=CARTESIAN_POINT('Ctrl Pts',(9.01440965049155,-20.3599135373691,0.));
#32561=CARTESIAN_POINT('Ctrl Pts',(9.01440965049155,-20.3599135373691,18.));
#32562=CARTESIAN_POINT('Ctrl Pts',(9.02698833758324,-20.2741136736186,0.));
#32563=CARTESIAN_POINT('Ctrl Pts',(9.02698833758324,-20.2741136736186,18.));
#32564=CARTESIAN_POINT('Ctrl Pts',(9.03891298737031,-20.1884025764493,0.));
#32565=CARTESIAN_POINT('Ctrl Pts',(9.03891298737031,-20.1884025764493,18.));
#32566=CARTESIAN_POINT('Ctrl Pts',(9.0501789809071,-20.1027850670435,0.));
#32567=CARTESIAN_POINT('Ctrl Pts',(9.0501789809071,-20.1027850670435,18.));
#32568=CARTESIAN_POINT('Ctrl Pts',(9.0607810967537,-20.0172662790811,0.));
#32569=CARTESIAN_POINT('Ctrl Pts',(9.0607810967537,-20.0172662790811,18.));
#32570=CARTESIAN_POINT('Ctrl Pts',(9.0707138821585,-19.9318514954605,0.));
#32571=CARTESIAN_POINT('Ctrl Pts',(9.0707138821585,-19.9318514954605,18.));
#32572=CARTESIAN_POINT('Ctrl Pts',(9.07997196979668,-19.846546013708,0.));
#32573=CARTESIAN_POINT('Ctrl Pts',(9.07997196979668,-19.846546013708,18.));
#32574=CARTESIAN_POINT('Ctrl Pts',(9.08855038355401,-19.7613550146978,0.));
#32575=CARTESIAN_POINT('Ctrl Pts',(9.08855038355401,-19.7613550146978,18.));
#32576=CARTESIAN_POINT('Ctrl Pts',(9.0964449428387,-19.6762833927168,0.));
#32577=CARTESIAN_POINT('Ctrl Pts',(9.0964449428387,-19.6762833927168,18.));
#32578=CARTESIAN_POINT('Ctrl Pts',(9.10365235736464,-19.5913357132276,0.));
#32579=CARTESIAN_POINT('Ctrl Pts',(9.10365235736464,-19.5913357132276,18.));
#32580=CARTESIAN_POINT('Ctrl Pts',(9.11016929611335,-19.5065165934577,0.));
#32581=CARTESIAN_POINT('Ctrl Pts',(9.11016929611335,-19.5065165934577,18.));
#32582=CARTESIAN_POINT('Ctrl Pts',(9.11599159243919,-19.4218310275711,0.));
#32583=CARTESIAN_POINT('Ctrl Pts',(9.11599159243919,-19.4218310275711,18.));
#32584=CARTESIAN_POINT('Ctrl Pts',(9.12111347941199,-19.3372847008483,0.));
#32585=CARTESIAN_POINT('Ctrl Pts',(9.12111347941199,-19.3372847008483,18.));
#32586=CARTESIAN_POINT('Ctrl Pts',(9.12552662785599,-19.2528843844341,0.));
#32587=CARTESIAN_POINT('Ctrl Pts',(9.12552662785599,-19.2528843844341,18.));
#32588=CARTESIAN_POINT('Ctrl Pts',(9.12921984349375,-19.1686380639041,0.));
#32589=CARTESIAN_POINT('Ctrl Pts',(9.12921984349375,-19.1686380639041,18.));
#32590=CARTESIAN_POINT('Ctrl Pts',(9.13218114462419,-19.0845541036965,0.));
#32591=CARTESIAN_POINT('Ctrl Pts',(9.13218114462419,-19.0845541036965,18.));
#32592=CARTESIAN_POINT('Ctrl Pts',(9.13439956903532,-19.0006405223697,0.));
#32593=CARTESIAN_POINT('Ctrl Pts',(9.13439956903532,-19.0006405223697,18.));
#32594=CARTESIAN_POINT('Ctrl Pts',(9.13586688858168,-18.9169043053388,0.));
#32595=CARTESIAN_POINT('Ctrl Pts',(9.13586688858168,-18.9169043053388,18.));
#32596=CARTESIAN_POINT('Ctrl Pts',(9.13657985367153,-18.8333505052874,0.));
#32597=CARTESIAN_POINT('Ctrl Pts',(9.13657985367153,-18.8333505052874,18.));
#32598=CARTESIAN_POINT('Ctrl Pts',(9.13654074021147,-18.7499820263476,0.));
#32599=CARTESIAN_POINT('Ctrl Pts',(9.13654074021147,-18.7499820263476,18.));
#32600=CARTESIAN_POINT('Ctrl Pts',(9.13575227582418,-18.6668016710749,0.));
#32601=CARTESIAN_POINT('Ctrl Pts',(9.13575227582418,-18.6668016710749,18.));
#32602=CARTESIAN_POINT('Ctrl Pts',(9.13421321934922,-18.5838139250423,0.));
#32603=CARTESIAN_POINT('Ctrl Pts',(9.13421321934922,-18.5838139250423,18.));
#32604=CARTESIAN_POINT('Ctrl Pts',(9.13191425549883,-18.5010266156389,0.));
#32605=CARTESIAN_POINT('Ctrl Pts',(9.13191425549883,-18.5010266156389,18.));
#32606=CARTESIAN_POINT('Ctrl Pts',(9.12883240135631,-18.4184531695731,0.));
#32607=CARTESIAN_POINT('Ctrl Pts',(9.12883240135631,-18.4184531695731,18.));
#32608=CARTESIAN_POINT('Ctrl Pts',(9.12493031448671,-18.3361129010289,0.));
#32609=CARTESIAN_POINT('Ctrl Pts',(9.12493031448671,-18.3361129010289,18.));
#32610=CARTESIAN_POINT('Ctrl Pts',(9.12016808144599,-18.2540262849075,0.));
#32611=CARTESIAN_POINT('Ctrl Pts',(9.12016808144599,-18.2540262849075,18.));
#32612=CARTESIAN_POINT('Ctrl Pts',(9.11451347590539,-18.1722108451637,0.));
#32613=CARTESIAN_POINT('Ctrl Pts',(9.11451347590539,-18.1722108451637,18.));
#32614=CARTESIAN_POINT('Ctrl Pts',(9.10795114540259,-18.0906774757189,0.));
#32615=CARTESIAN_POINT('Ctrl Pts',(9.10795114540259,-18.0906774757189,18.));
#32616=CARTESIAN_POINT('Ctrl Pts',(9.10049631917583,-18.0094249416472,0.));
#32617=CARTESIAN_POINT('Ctrl Pts',(9.10049631917583,-18.0094249416472,18.));
#32618=CARTESIAN_POINT('Ctrl Pts',(9.09219303320079,-17.9284406141976,0.));
#32619=CARTESIAN_POINT('Ctrl Pts',(9.09219303320079,-17.9284406141976,18.));
#32620=CARTESIAN_POINT('Ctrl Pts',(9.08308548608349,-17.8477120247758,0.));
#32621=CARTESIAN_POINT('Ctrl Pts',(9.08308548608349,-17.8477120247758,18.));
#32622=CARTESIAN_POINT('Ctrl Pts',(9.07319314215026,-17.7672369091005,0.));
#32623=CARTESIAN_POINT('Ctrl Pts',(9.07319314215026,-17.7672369091005,18.));
#32624=CARTESIAN_POINT('Ctrl Pts',(9.06248904941394,-17.6870319618808,0.));
#32625=CARTESIAN_POINT('Ctrl Pts',(9.06248904941394,-17.6870319618808,18.));
#32626=CARTESIAN_POINT('Ctrl Pts',(9.05086524971401,-17.6071467783263,0.));
#32627=CARTESIAN_POINT('Ctrl Pts',(9.05086524971401,-17.6071467783263,18.));
#32628=CARTESIAN_POINT('Ctrl Pts',(9.03814678971601,-17.5276582702181,0.));
#32629=CARTESIAN_POINT('Ctrl Pts',(9.03814678971601,-17.5276582702181,18.));
#32630=CARTESIAN_POINT('Ctrl Pts',(9.0241575097608,-17.4486443043185,0.));
#32631=CARTESIAN_POINT('Ctrl Pts',(9.0241575097608,-17.4486443043185,18.));
#32632=CARTESIAN_POINT('Ctrl Pts',(9.00877780436036,-17.3701605263553,0.));
#32633=CARTESIAN_POINT('Ctrl Pts',(9.00877780436036,-17.3701605263553,18.));
#32634=CARTESIAN_POINT('Ctrl Pts',(8.99199362652256,-17.2922207948279,0.));
#32635=CARTESIAN_POINT('Ctrl Pts',(8.99199362652256,-17.2922207948279,18.));
#32636=CARTESIAN_POINT('Ctrl Pts',(8.97397941759265,-17.2147637614528,0.));
#32637=CARTESIAN_POINT('Ctrl Pts',(8.97397941759265,-17.2147637614528,18.));
#32638=CARTESIAN_POINT('Ctrl Pts',(8.95502702208203,-17.1376822726252,0.));
#32639=CARTESIAN_POINT('Ctrl Pts',(8.95502702208203,-17.1376822726252,18.));
#32640=CARTESIAN_POINT('Ctrl Pts',(8.93538377395243,-17.0608897634975,0.));
#32641=CARTESIAN_POINT('Ctrl Pts',(8.93538377395243,-17.0608897634975,18.));
#32642=CARTESIAN_POINT('Ctrl Pts',(8.91510993758932,-16.9843788566346,0.));
#32643=CARTESIAN_POINT('Ctrl Pts',(8.91510993758932,-16.9843788566346,18.));
#32644=CARTESIAN_POINT('Ctrl Pts',(8.89394614661328,-16.908275670167,0.));
#32645=CARTESIAN_POINT('Ctrl Pts',(8.89394614661328,-16.908275670167,18.));
#32646=CARTESIAN_POINT('Ctrl Pts',(8.87112909692392,-16.8329157811062,0.));
#32647=CARTESIAN_POINT('Ctrl Pts',(8.87112909692392,-16.8329157811062,18.));
#32648=CARTESIAN_POINT('Ctrl Pts',(8.84558256033742,-16.7587634618101,0.));
#32649=CARTESIAN_POINT('Ctrl Pts',(8.84558256033742,-16.7587634618101,18.));
#32650=CARTESIAN_POINT('Ctrl Pts',(8.82207984677446,-16.7007854423938,0.));
#32651=CARTESIAN_POINT('Ctrl Pts',(8.82207984677446,-16.7007854423938,18.));
#32652=CARTESIAN_POINT('Ctrl Pts',(8.8023348179895,-16.6582257921024,0.));
#32653=CARTESIAN_POINT('Ctrl Pts',(8.8023348179895,-16.6582257921024,18.));
#32654=CARTESIAN_POINT('Ctrl Pts',(8.78817964150685,-16.6302847808193,0.));
#32655=CARTESIAN_POINT('Ctrl Pts',(8.78817964150685,-16.6302847808193,18.));
#32656=CARTESIAN_POINT('Ctrl Pts',(8.78085409196639,-16.6164222996225,0.));
#32657=CARTESIAN_POINT('Ctrl Pts',(8.78085409196639,-16.6164222996225,18.));
#32658=CARTESIAN_POINT('',(8.52496423935279,-22.4349054983023,0.));
#32659=CARTESIAN_POINT('Ctrl Pts',(8.78085409196639,-16.6164222996225,0.));
#32660=CARTESIAN_POINT('Ctrl Pts',(8.78817964150685,-16.6302847808193,0.));
#32661=CARTESIAN_POINT('Ctrl Pts',(8.8023348179895,-16.6582257921024,0.));
#32662=CARTESIAN_POINT('Ctrl Pts',(8.82207984677446,-16.7007854423938,0.));
#32663=CARTESIAN_POINT('Ctrl Pts',(8.84558256033742,-16.7587634618101,0.));
#32664=CARTESIAN_POINT('Ctrl Pts',(8.87112909692392,-16.8329157811062,0.));
#32665=CARTESIAN_POINT('Ctrl Pts',(8.89394614661328,-16.908275670167,0.));
#32666=CARTESIAN_POINT('Ctrl Pts',(8.91510993758932,-16.9843788566346,0.));
#32667=CARTESIAN_POINT('Ctrl Pts',(8.93538377395243,-17.0608897634975,0.));
#32668=CARTESIAN_POINT('Ctrl Pts',(8.95502702208203,-17.1376822726252,0.));
#32669=CARTESIAN_POINT('Ctrl Pts',(8.97397941759265,-17.2147637614528,0.));
#32670=CARTESIAN_POINT('Ctrl Pts',(8.99199362652256,-17.2922207948279,0.));
#32671=CARTESIAN_POINT('Ctrl Pts',(9.00877780436036,-17.3701605263553,0.));
#32672=CARTESIAN_POINT('Ctrl Pts',(9.0241575097608,-17.4486443043185,0.));
#32673=CARTESIAN_POINT('Ctrl Pts',(9.03814678971601,-17.5276582702181,0.));
#32674=CARTESIAN_POINT('Ctrl Pts',(9.05086524971401,-17.6071467783263,0.));
#32675=CARTESIAN_POINT('Ctrl Pts',(9.06248904941394,-17.6870319618808,0.));
#32676=CARTESIAN_POINT('Ctrl Pts',(9.07319314215026,-17.7672369091005,0.));
#32677=CARTESIAN_POINT('Ctrl Pts',(9.08308548608349,-17.8477120247758,0.));
#32678=CARTESIAN_POINT('Ctrl Pts',(9.09219303320079,-17.9284406141976,0.));
#32679=CARTESIAN_POINT('Ctrl Pts',(9.10049631917583,-18.0094249416472,0.));
#32680=CARTESIAN_POINT('Ctrl Pts',(9.10795114540259,-18.0906774757189,0.));
#32681=CARTESIAN_POINT('Ctrl Pts',(9.11451347590539,-18.1722108451637,0.));
#32682=CARTESIAN_POINT('Ctrl Pts',(9.12016808144599,-18.2540262849075,0.));
#32683=CARTESIAN_POINT('Ctrl Pts',(9.12493031448671,-18.3361129010289,0.));
#32684=CARTESIAN_POINT('Ctrl Pts',(9.12883240135631,-18.4184531695731,0.));
#32685=CARTESIAN_POINT('Ctrl Pts',(9.13191425549883,-18.5010266156389,0.));
#32686=CARTESIAN_POINT('Ctrl Pts',(9.13421321934922,-18.5838139250423,0.));
#32687=CARTESIAN_POINT('Ctrl Pts',(9.13575227582418,-18.6668016710749,0.));
#32688=CARTESIAN_POINT('Ctrl Pts',(9.13654074021147,-18.7499820263476,0.));
#32689=CARTESIAN_POINT('Ctrl Pts',(9.13657985367153,-18.8333505052874,0.));
#32690=CARTESIAN_POINT('Ctrl Pts',(9.13586688858168,-18.9169043053388,0.));
#32691=CARTESIAN_POINT('Ctrl Pts',(9.13439956903532,-19.0006405223697,0.));
#32692=CARTESIAN_POINT('Ctrl Pts',(9.13218114462419,-19.0845541036965,0.));
#32693=CARTESIAN_POINT('Ctrl Pts',(9.12921984349375,-19.1686380639041,0.));
#32694=CARTESIAN_POINT('Ctrl Pts',(9.12552662785599,-19.2528843844341,0.));
#32695=CARTESIAN_POINT('Ctrl Pts',(9.12111347941199,-19.3372847008483,0.));
#32696=CARTESIAN_POINT('Ctrl Pts',(9.11599159243919,-19.4218310275711,0.));
#32697=CARTESIAN_POINT('Ctrl Pts',(9.11016929611335,-19.5065165934577,0.));
#32698=CARTESIAN_POINT('Ctrl Pts',(9.10365235736464,-19.5913357132276,0.));
#32699=CARTESIAN_POINT('Ctrl Pts',(9.0964449428387,-19.6762833927168,0.));
#32700=CARTESIAN_POINT('Ctrl Pts',(9.08855038355401,-19.7613550146978,0.));
#32701=CARTESIAN_POINT('Ctrl Pts',(9.07997196979668,-19.846546013708,0.));
#32702=CARTESIAN_POINT('Ctrl Pts',(9.0707138821585,-19.9318514954605,0.));
#32703=CARTESIAN_POINT('Ctrl Pts',(9.0607810967537,-20.0172662790811,0.));
#32704=CARTESIAN_POINT('Ctrl Pts',(9.0501789809071,-20.1027850670435,0.));
#32705=CARTESIAN_POINT('Ctrl Pts',(9.03891298737031,-20.1884025764493,0.));
#32706=CARTESIAN_POINT('Ctrl Pts',(9.02698833758324,-20.2741136736186,0.));
#32707=CARTESIAN_POINT('Ctrl Pts',(9.01440965049155,-20.3599135373691,0.));
#32708=CARTESIAN_POINT('Ctrl Pts',(9.00118097039516,-20.4457976315472,0.));
#32709=CARTESIAN_POINT('Ctrl Pts',(8.98730595457659,-20.5317616031369,0.));
#32710=CARTESIAN_POINT('Ctrl Pts',(8.97278801890467,-20.6178012000199,0.));
#32711=CARTESIAN_POINT('Ctrl Pts',(8.95763049112623,-20.7039121898975,0.));
#32712=CARTESIAN_POINT('Ctrl Pts',(8.94183680111377,-20.7900902537083,0.));
#32713=CARTESIAN_POINT('Ctrl Pts',(8.92541048738648,-20.8763310073304,0.));
#32714=CARTESIAN_POINT('Ctrl Pts',(8.90835509843284,-20.9626300944902,0.));
#32715=CARTESIAN_POINT('Ctrl Pts',(8.89067412773385,-21.0489832630915,0.));
#32716=CARTESIAN_POINT('Ctrl Pts',(8.87237094640748,-21.1353864352374,0.));
#32717=CARTESIAN_POINT('Ctrl Pts',(8.85344872418155,-21.2218358113425,0.));
#32718=CARTESIAN_POINT('Ctrl Pts',(8.83391042911628,-21.3083278326642,0.));
#32719=CARTESIAN_POINT('Ctrl Pts',(8.81375890120581,-21.3948590173441,0.));
#32720=CARTESIAN_POINT('Ctrl Pts',(8.79299691277858,-21.481425822209,0.));
#32721=CARTESIAN_POINT('Ctrl Pts',(8.77162723103298,-21.5680245138584,0.));
#32722=CARTESIAN_POINT('Ctrl Pts',(8.74965270266163,-21.6546509866725,0.));
#32723=CARTESIAN_POINT('Ctrl Pts',(8.72707626956921,-21.7413007707864,0.));
#32724=CARTESIAN_POINT('Ctrl Pts',(8.70390086252202,-21.8279693631274,0.));
#32725=CARTESIAN_POINT('Ctrl Pts',(8.68012932645739,-21.9146524902336,0.));
#32726=CARTESIAN_POINT('Ctrl Pts',(8.6557643376698,-22.0013463859623,0.));
#32727=CARTESIAN_POINT('Ctrl Pts',(8.63080832792612,-22.0880480931906,0.));
#32728=CARTESIAN_POINT('Ctrl Pts',(8.60015442890613,-22.1920971794848,0.));
#32729=CARTESIAN_POINT('Ctrl Pts',(8.57387555634004,-22.2788106077806,0.));
#32730=CARTESIAN_POINT('Ctrl Pts',(8.55238412336293,-22.3481844703457,0.));
#32731=CARTESIAN_POINT('Ctrl Pts',(8.53600237317212,-22.400216619619,0.));
#32732=CARTESIAN_POINT('Ctrl Pts',(8.52496423935284,-22.4349054983023,0.));
#32733=CARTESIAN_POINT('',(8.52496423935279,-22.4349054983023,15.));
#32734=CARTESIAN_POINT('Ctrl Pts',(8.52496423935284,-22.4349054983023,15.));
#32735=CARTESIAN_POINT('Ctrl Pts',(8.53048330625154,-22.4175610589877,15.));
#32736=CARTESIAN_POINT('Ctrl Pts',(8.54146295656906,-22.3828725698612,15.));
#32737=CARTESIAN_POINT('Ctrl Pts',(8.55775698160721,-22.3308410047044,15.));
#32738=CARTESIAN_POINT('Ctrl Pts',(8.57913133085326,-22.2614679221214,15.));
#32739=CARTESIAN_POINT('Ctrl Pts',(8.60526341207613,-22.1747556651024,15.));
#32740=CARTESIAN_POINT('Ctrl Pts',(8.63080832792612,-22.0880480931906,15.));
#32741=CARTESIAN_POINT('Ctrl Pts',(8.6557643376698,-22.0013463859623,15.));
#32742=CARTESIAN_POINT('Ctrl Pts',(8.68012932645739,-21.9146524902336,15.));
#32743=CARTESIAN_POINT('Ctrl Pts',(8.70390086252202,-21.8279693631274,15.));
#32744=CARTESIAN_POINT('Ctrl Pts',(8.72707626956921,-21.7413007707864,15.));
#32745=CARTESIAN_POINT('Ctrl Pts',(8.74965270266163,-21.6546509866725,15.));
#32746=CARTESIAN_POINT('Ctrl Pts',(8.77162723103298,-21.5680245138584,15.));
#32747=CARTESIAN_POINT('Ctrl Pts',(8.79299691277858,-21.481425822209,15.));
#32748=CARTESIAN_POINT('Ctrl Pts',(8.81375890120581,-21.3948590173441,15.));
#32749=CARTESIAN_POINT('Ctrl Pts',(8.83391042911628,-21.3083278326642,15.));
#32750=CARTESIAN_POINT('Ctrl Pts',(8.85344872418155,-21.2218358113425,15.));
#32751=CARTESIAN_POINT('Ctrl Pts',(8.87237094640748,-21.1353864352374,15.));
#32752=CARTESIAN_POINT('Ctrl Pts',(8.89067412773385,-21.0489832630915,15.));
#32753=CARTESIAN_POINT('Ctrl Pts',(8.90835509843284,-20.9626300944902,15.));
#32754=CARTESIAN_POINT('Ctrl Pts',(8.92541048738648,-20.8763310073304,15.));
#32755=CARTESIAN_POINT('Ctrl Pts',(8.94183680111377,-20.7900902537083,15.));
#32756=CARTESIAN_POINT('Ctrl Pts',(8.95763049112623,-20.7039121898975,15.));
#32757=CARTESIAN_POINT('Ctrl Pts',(8.97278801890467,-20.6178012000199,15.));
#32758=CARTESIAN_POINT('Ctrl Pts',(8.98730595457659,-20.5317616031369,15.));
#32759=CARTESIAN_POINT('Ctrl Pts',(9.00118097039516,-20.4457976315472,15.));
#32760=CARTESIAN_POINT('Ctrl Pts',(9.01440965049155,-20.3599135373691,15.));
#32761=CARTESIAN_POINT('Ctrl Pts',(9.02698833758324,-20.2741136736186,15.));
#32762=CARTESIAN_POINT('Ctrl Pts',(9.03891298737031,-20.1884025764493,15.));
#32763=CARTESIAN_POINT('Ctrl Pts',(9.0501789809071,-20.1027850670435,15.));
#32764=CARTESIAN_POINT('Ctrl Pts',(9.0607810967537,-20.0172662790811,15.));
#32765=CARTESIAN_POINT('Ctrl Pts',(9.0707138821585,-19.9318514954605,15.));
#32766=CARTESIAN_POINT('Ctrl Pts',(9.07997196979668,-19.846546013708,15.));
#32767=CARTESIAN_POINT('Ctrl Pts',(9.08855038355401,-19.7613550146978,15.));
#32768=CARTESIAN_POINT('Ctrl Pts',(9.0964449428387,-19.6762833927168,15.));
#32769=CARTESIAN_POINT('Ctrl Pts',(9.10365235736464,-19.5913357132276,15.));
#32770=CARTESIAN_POINT('Ctrl Pts',(9.11016929611335,-19.5065165934577,15.));
#32771=CARTESIAN_POINT('Ctrl Pts',(9.11599159243919,-19.4218310275711,15.));
#32772=CARTESIAN_POINT('Ctrl Pts',(9.12111347941199,-19.3372847008483,15.));
#32773=CARTESIAN_POINT('Ctrl Pts',(9.12552662785599,-19.2528843844341,15.));
#32774=CARTESIAN_POINT('Ctrl Pts',(9.12921984349375,-19.1686380639041,15.));
#32775=CARTESIAN_POINT('Ctrl Pts',(9.13218114462419,-19.0845541036965,15.));
#32776=CARTESIAN_POINT('Ctrl Pts',(9.13439956903532,-19.0006405223697,15.));
#32777=CARTESIAN_POINT('Ctrl Pts',(9.13586688858168,-18.9169043053388,15.));
#32778=CARTESIAN_POINT('Ctrl Pts',(9.13657985367153,-18.8333505052874,15.));
#32779=CARTESIAN_POINT('Ctrl Pts',(9.13654074021147,-18.7499820263476,15.));
#32780=CARTESIAN_POINT('Ctrl Pts',(9.13575227582418,-18.6668016710749,15.));
#32781=CARTESIAN_POINT('Ctrl Pts',(9.13421321934922,-18.5838139250423,15.));
#32782=CARTESIAN_POINT('Ctrl Pts',(9.13191425549883,-18.5010266156389,15.));
#32783=CARTESIAN_POINT('Ctrl Pts',(9.12883240135631,-18.4184531695731,15.));
#32784=CARTESIAN_POINT('Ctrl Pts',(9.12493031448671,-18.3361129010289,15.));
#32785=CARTESIAN_POINT('Ctrl Pts',(9.12016808144599,-18.2540262849075,15.));
#32786=CARTESIAN_POINT('Ctrl Pts',(9.11451347590539,-18.1722108451637,15.));
#32787=CARTESIAN_POINT('Ctrl Pts',(9.10795114540259,-18.0906774757189,15.));
#32788=CARTESIAN_POINT('Ctrl Pts',(9.10049631917583,-18.0094249416472,15.));
#32789=CARTESIAN_POINT('Ctrl Pts',(9.09219303320079,-17.9284406141976,15.));
#32790=CARTESIAN_POINT('Ctrl Pts',(9.08308548608349,-17.8477120247758,15.));
#32791=CARTESIAN_POINT('Ctrl Pts',(9.07319314215026,-17.7672369091005,15.));
#32792=CARTESIAN_POINT('Ctrl Pts',(9.06248904941394,-17.6870319618808,15.));
#32793=CARTESIAN_POINT('Ctrl Pts',(9.05086524971401,-17.6071467783263,15.));
#32794=CARTESIAN_POINT('Ctrl Pts',(9.03814678971601,-17.5276582702181,15.));
#32795=CARTESIAN_POINT('Ctrl Pts',(9.0241575097608,-17.4486443043185,15.));
#32796=CARTESIAN_POINT('Ctrl Pts',(9.00877780436036,-17.3701605263553,15.));
#32797=CARTESIAN_POINT('Ctrl Pts',(8.99199362652256,-17.2922207948279,15.));
#32798=CARTESIAN_POINT('Ctrl Pts',(8.97397941759265,-17.2147637614528,15.));
#32799=CARTESIAN_POINT('Ctrl Pts',(8.95502702208203,-17.1376822726252,15.));
#32800=CARTESIAN_POINT('Ctrl Pts',(8.93538377395243,-17.0608897634975,15.));
#32801=CARTESIAN_POINT('Ctrl Pts',(8.91510993758932,-16.9843788566346,15.));
#32802=CARTESIAN_POINT('Ctrl Pts',(8.89394614661328,-16.908275670167,15.));
#32803=CARTESIAN_POINT('Ctrl Pts',(8.87112909692392,-16.8329157811062,15.));
#32804=CARTESIAN_POINT('Ctrl Pts',(8.84558256033742,-16.7587634618101,15.));
#32805=CARTESIAN_POINT('Ctrl Pts',(8.82207984677446,-16.7007854423938,15.));
#32806=CARTESIAN_POINT('Ctrl Pts',(8.8023348179895,-16.6582257921024,15.));
#32807=CARTESIAN_POINT('Ctrl Pts',(8.78817964150685,-16.6302847808193,15.));
#32808=CARTESIAN_POINT('Ctrl Pts',(8.78085409196639,-16.6164222996225,15.));
#32809=CARTESIAN_POINT('',(8.52496423935279,-22.4349054983023,0.));
#32810=CARTESIAN_POINT('Origin',(3.56140965415431E-14,-1.09833465940894E-13,
0.));
#32811=CARTESIAN_POINT('',(6.29006564240226,-23.1610680715348,0.));
#32812=CARTESIAN_POINT('Origin',(3.56140965415431E-14,-1.09833465940894E-13,
0.));
#32813=CARTESIAN_POINT('',(6.29006564240226,-23.1610680715348,15.));
#32814=CARTESIAN_POINT('Origin',(3.56140965415431E-14,-1.09833465940894E-13,
15.));
#32815=CARTESIAN_POINT('',(6.29006564240226,-23.1610680715348,0.));
#32816=CARTESIAN_POINT('Ctrl Pts',(2.66302778805429,-18.6042245638953,0.));
#32817=CARTESIAN_POINT('Ctrl Pts',(2.66302778805429,-18.6042245638953,18.));
#32818=CARTESIAN_POINT('Ctrl Pts',(2.66524945599054,-18.6197453967525,0.));
#32819=CARTESIAN_POINT('Ctrl Pts',(2.66524945599054,-18.6197453967525,18.));
#32820=CARTESIAN_POINT('Ctrl Pts',(2.67022099202408,-18.6506703537007,0.));
#32821=CARTESIAN_POINT('Ctrl Pts',(2.67022099202408,-18.6506703537007,18.));
#32822=CARTESIAN_POINT('Ctrl Pts',(2.67926286296661,-18.696707670787,0.));
#32823=CARTESIAN_POINT('Ctrl Pts',(2.67926286296661,-18.696707670787,18.));
#32824=CARTESIAN_POINT('Ctrl Pts',(2.69432739305027,-18.7574274222161,0.));
#32825=CARTESIAN_POINT('Ctrl Pts',(2.69432739305027,-18.7574274222161,18.));
#32826=CARTESIAN_POINT('Ctrl Pts',(2.71724545050994,-18.8324337861517,0.));
#32827=CARTESIAN_POINT('Ctrl Pts',(2.71724545050994,-18.8324337861517,18.));
#32828=CARTESIAN_POINT('Ctrl Pts',(2.74308150095404,-18.9068127424043,0.));
#32829=CARTESIAN_POINT('Ctrl Pts',(2.74308150095404,-18.9068127424043,18.));
#32830=CARTESIAN_POINT('Ctrl Pts',(2.77069196504715,-18.980821277801,0.));
#32831=CARTESIAN_POINT('Ctrl Pts',(2.77069196504715,-18.980821277801,18.));
#32832=CARTESIAN_POINT('Ctrl Pts',(2.79926206958176,-19.0546365637297,0.));
#32833=CARTESIAN_POINT('Ctrl Pts',(2.79926206958176,-19.0546365637297,18.));
#32834=CARTESIAN_POINT('Ctrl Pts',(2.828507852372,-19.1283090202125,0.));
#32835=CARTESIAN_POINT('Ctrl Pts',(2.828507852372,-19.1283090202125,18.));
#32836=CARTESIAN_POINT('Ctrl Pts',(2.85848240467741,-19.2018091932025,0.));
#32837=CARTESIAN_POINT('Ctrl Pts',(2.85848240467741,-19.2018091932025,18.));
#32838=CARTESIAN_POINT('Ctrl Pts',(2.88943670541708,-19.2750617358775,0.));
#32839=CARTESIAN_POINT('Ctrl Pts',(2.88943670541708,-19.2750617358775,18.));
#32840=CARTESIAN_POINT('Ctrl Pts',(2.92166984506915,-19.3479817954251,0.));
#32841=CARTESIAN_POINT('Ctrl Pts',(2.92166984506915,-19.3479817954251,18.));
#32842=CARTESIAN_POINT('Ctrl Pts',(2.95535900926266,-19.420516469599,0.));
#32843=CARTESIAN_POINT('Ctrl Pts',(2.95535900926266,-19.420516469599,18.));
#32844=CARTESIAN_POINT('Ctrl Pts',(2.99048468792079,-19.4926628032527,0.));
#32845=CARTESIAN_POINT('Ctrl Pts',(2.99048468792079,-19.4926628032527,18.));
#32846=CARTESIAN_POINT('Ctrl Pts',(3.02691741043283,-19.5644460803884,0.));
#32847=CARTESIAN_POINT('Ctrl Pts',(3.02691741043283,-19.5644460803884,18.));
#32848=CARTESIAN_POINT('Ctrl Pts',(3.06446889170638,-19.635906849522,0.));
#32849=CARTESIAN_POINT('Ctrl Pts',(3.06446889170638,-19.635906849522,18.));
#32850=CARTESIAN_POINT('Ctrl Pts',(3.10295238390997,-19.7070857227052,0.));
#32851=CARTESIAN_POINT('Ctrl Pts',(3.10295238390997,-19.7070857227052,18.));
#32852=CARTESIAN_POINT('Ctrl Pts',(3.1422513957243,-19.7780060327855,0.));
#32853=CARTESIAN_POINT('Ctrl Pts',(3.1422513957243,-19.7780060327855,18.));
#32854=CARTESIAN_POINT('Ctrl Pts',(3.18233430962982,-19.8486701154397,0.));
#32855=CARTESIAN_POINT('Ctrl Pts',(3.18233430962982,-19.8486701154397,18.));
#32856=CARTESIAN_POINT('Ctrl Pts',(3.22321820350857,-19.9190683616661,0.));
#32857=CARTESIAN_POINT('Ctrl Pts',(3.22321820350857,-19.9190683616661,18.));
#32858=CARTESIAN_POINT('Ctrl Pts',(3.26494616363974,-19.9891848794807,0.));
#32859=CARTESIAN_POINT('Ctrl Pts',(3.26494616363974,-19.9891848794807,18.));
#32860=CARTESIAN_POINT('Ctrl Pts',(3.30756123886962,-20.0590040020604,0.));
#32861=CARTESIAN_POINT('Ctrl Pts',(3.30756123886962,-20.0590040020604,18.));
#32862=CARTESIAN_POINT('Ctrl Pts',(3.351076475782,-20.1285177769596,0.));
#32863=CARTESIAN_POINT('Ctrl Pts',(3.351076475782,-20.1285177769596,18.));
#32864=CARTESIAN_POINT('Ctrl Pts',(3.39547305068767,-20.1977264147619,0.));
#32865=CARTESIAN_POINT('Ctrl Pts',(3.39547305068767,-20.1977264147619,18.));
#32866=CARTESIAN_POINT('Ctrl Pts',(3.44071459161672,-20.2666346804507,0.));
#32867=CARTESIAN_POINT('Ctrl Pts',(3.44071459161672,-20.2666346804507,18.));
#32868=CARTESIAN_POINT('Ctrl Pts',(3.48675677306966,-20.3352494700167,0.));
#32869=CARTESIAN_POINT('Ctrl Pts',(3.48675677306966,-20.3352494700167,18.));
#32870=CARTESIAN_POINT('Ctrl Pts',(3.53355803178954,-20.4035771072894,0.));
#32871=CARTESIAN_POINT('Ctrl Pts',(3.53355803178954,-20.4035771072894,18.));
#32872=CARTESIAN_POINT('Ctrl Pts',(3.58109188218494,-20.4716202388531,0.));
#32873=CARTESIAN_POINT('Ctrl Pts',(3.58109188218494,-20.4716202388531,18.));
#32874=CARTESIAN_POINT('Ctrl Pts',(3.62934618720589,-20.5393780076056,0.));
#32875=CARTESIAN_POINT('Ctrl Pts',(3.62934618720589,-20.5393780076056,18.));
#32876=CARTESIAN_POINT('Ctrl Pts',(3.67831730617887,-20.6068475141781,0.));
#32877=CARTESIAN_POINT('Ctrl Pts',(3.67831730617887,-20.6068475141781,18.));
#32878=CARTESIAN_POINT('Ctrl Pts',(3.72800579849619,-20.6740248879992,0.));
#32879=CARTESIAN_POINT('Ctrl Pts',(3.72800579849619,-20.6740248879992,18.));
#32880=CARTESIAN_POINT('Ctrl Pts',(3.77841179839888,-20.740906441832,0.));
#32881=CARTESIAN_POINT('Ctrl Pts',(3.77841179839888,-20.740906441832,18.));
#32882=CARTESIAN_POINT('Ctrl Pts',(3.82952970701915,-20.8074899980321,0.));
#32883=CARTESIAN_POINT('Ctrl Pts',(3.82952970701915,-20.8074899980321,18.));
#32884=CARTESIAN_POINT('Ctrl Pts',(3.88134876172353,-20.8737747416623,0.));
#32885=CARTESIAN_POINT('Ctrl Pts',(3.88134876172353,-20.8737747416623,18.));
#32886=CARTESIAN_POINT('Ctrl Pts',(3.93385538070582,-20.9397606289993,0.));
#32887=CARTESIAN_POINT('Ctrl Pts',(3.93385538070582,-20.9397606289993,18.));
#32888=CARTESIAN_POINT('Ctrl Pts',(3.98703495407281,-21.0054479357374,0.));
#32889=CARTESIAN_POINT('Ctrl Pts',(3.98703495407281,-21.0054479357374,18.));
#32890=CARTESIAN_POINT('Ctrl Pts',(4.04087373166023,-21.0708367812416,0.));
#32891=CARTESIAN_POINT('Ctrl Pts',(4.04087373166023,-21.0708367812416,18.));
#32892=CARTESIAN_POINT('Ctrl Pts',(4.09536099504429,-21.1359265833073,0.));
#32893=CARTESIAN_POINT('Ctrl Pts',(4.09536099504429,-21.1359265833073,18.));
#32894=CARTESIAN_POINT('Ctrl Pts',(4.15048873695645,-21.2007161321625,0.));
#32895=CARTESIAN_POINT('Ctrl Pts',(4.15048873695645,-21.2007161321625,18.));
#32896=CARTESIAN_POINT('Ctrl Pts',(4.20625065101369,-21.2652038365365,0.));
#32897=CARTESIAN_POINT('Ctrl Pts',(4.20625065101369,-21.2652038365365,18.));
#32898=CARTESIAN_POINT('Ctrl Pts',(4.26264132842711,-21.3293879189372,0.));
#32899=CARTESIAN_POINT('Ctrl Pts',(4.26264132842711,-21.3293879189372,18.));
#32900=CARTESIAN_POINT('Ctrl Pts',(4.31965542378783,-21.3932666198096,0.));
#32901=CARTESIAN_POINT('Ctrl Pts',(4.31965542378783,-21.3932666198096,18.));
#32902=CARTESIAN_POINT('Ctrl Pts',(4.37728667813637,-21.4568384368826,0.));
#32903=CARTESIAN_POINT('Ctrl Pts',(4.37728667813637,-21.4568384368826,18.));
#32904=CARTESIAN_POINT('Ctrl Pts',(4.43552802047029,-21.5201021036274,0.));
#32905=CARTESIAN_POINT('Ctrl Pts',(4.43552802047029,-21.5201021036274,18.));
#32906=CARTESIAN_POINT('Ctrl Pts',(4.49437199472474,-21.5830564890896,0.));
#32907=CARTESIAN_POINT('Ctrl Pts',(4.49437199472474,-21.5830564890896,18.));
#32908=CARTESIAN_POINT('Ctrl Pts',(4.55381108432127,-21.6457005243617,0.));
#32909=CARTESIAN_POINT('Ctrl Pts',(4.55381108432127,-21.6457005243617,18.));
#32910=CARTESIAN_POINT('Ctrl Pts',(4.6138380475249,-21.7080331252945,0.));
#32911=CARTESIAN_POINT('Ctrl Pts',(4.6138380475249,-21.7080331252945,18.));
#32912=CARTESIAN_POINT('Ctrl Pts',(4.67444631371023,-21.770053106418,0.));
#32913=CARTESIAN_POINT('Ctrl Pts',(4.67444631371023,-21.770053106418,18.));
#32914=CARTESIAN_POINT('Ctrl Pts',(4.73562994468575,-21.8317591750867,0.));
#32915=CARTESIAN_POINT('Ctrl Pts',(4.73562994468575,-21.8317591750867,18.));
#32916=CARTESIAN_POINT('Ctrl Pts',(4.7973834230091,-21.8931499593332,0.));
#32917=CARTESIAN_POINT('Ctrl Pts',(4.7973834230091,-21.8931499593332,18.));
#32918=CARTESIAN_POINT('Ctrl Pts',(4.85970148585195,-21.954224026919,0.));
#32919=CARTESIAN_POINT('Ctrl Pts',(4.85970148585195,-21.954224026919,18.));
#32920=CARTESIAN_POINT('Ctrl Pts',(4.92257895332778,-22.0149799098431,0.));
#32921=CARTESIAN_POINT('Ctrl Pts',(4.92257895332778,-22.0149799098431,18.));
#32922=CARTESIAN_POINT('Ctrl Pts',(4.98601051193086,-22.0754161299398,0.));
#32923=CARTESIAN_POINT('Ctrl Pts',(4.98601051193086,-22.0754161299398,18.));
#32924=CARTESIAN_POINT('Ctrl Pts',(5.0499907220168,-22.1355312202693,0.));
#32925=CARTESIAN_POINT('Ctrl Pts',(5.0499907220168,-22.1355312202693,18.));
#32926=CARTESIAN_POINT('Ctrl Pts',(5.11451415224483,-22.1953237422816,0.));
#32927=CARTESIAN_POINT('Ctrl Pts',(5.11451415224483,-22.1953237422816,18.));
#32928=CARTESIAN_POINT('Ctrl Pts',(5.17957547700992,-22.2547923093751,0.));
#32929=CARTESIAN_POINT('Ctrl Pts',(5.17957547700992,-22.2547923093751,18.));
#32930=CARTESIAN_POINT('Ctrl Pts',(5.24516957209272,-22.3139356039553,0.));
#32931=CARTESIAN_POINT('Ctrl Pts',(5.24516957209272,-22.3139356039553,18.));
#32932=CARTESIAN_POINT('Ctrl Pts',(5.31129163978934,-22.3727524152125,0.));
#32933=CARTESIAN_POINT('Ctrl Pts',(5.31129163978934,-22.3727524152125,18.));
#32934=CARTESIAN_POINT('Ctrl Pts',(5.37793718711213,-22.4312416086453,0.));
#32935=CARTESIAN_POINT('Ctrl Pts',(5.37793718711213,-22.4312416086453,18.));
#32936=CARTESIAN_POINT('Ctrl Pts',(5.44510186987254,-22.4894020366778,0.));
#32937=CARTESIAN_POINT('Ctrl Pts',(5.44510186987254,-22.4894020366778,18.));
#32938=CARTESIAN_POINT('Ctrl Pts',(5.51278136258485,-22.5472324623564,0.));
#32939=CARTESIAN_POINT('Ctrl Pts',(5.51278136258485,-22.5472324623564,18.));
#32940=CARTESIAN_POINT('Ctrl Pts',(5.58097123210075,-22.6047314918151,0.));
#32941=CARTESIAN_POINT('Ctrl Pts',(5.58097123210075,-22.6047314918151,18.));
#32942=CARTESIAN_POINT('Ctrl Pts',(5.64966676217478,-22.6618974767817,0.));
#32943=CARTESIAN_POINT('Ctrl Pts',(5.64966676217478,-22.6618974767817,18.));
#32944=CARTESIAN_POINT('Ctrl Pts',(5.71886294543539,-22.7187285302677,0.));
#32945=CARTESIAN_POINT('Ctrl Pts',(5.71886294543539,-22.7187285302677,18.));
#32946=CARTESIAN_POINT('Ctrl Pts',(5.7885547640031,-22.7752227318719,0.));
#32947=CARTESIAN_POINT('Ctrl Pts',(5.7885547640031,-22.7752227318719,18.));
#32948=CARTESIAN_POINT('Ctrl Pts',(5.85873740439746,-22.8313782965033,0.));
#32949=CARTESIAN_POINT('Ctrl Pts',(5.85873740439746,-22.8313782965033,18.));
#32950=CARTESIAN_POINT('Ctrl Pts',(5.92940648776744,-22.8871937503747,0.));
#32951=CARTESIAN_POINT('Ctrl Pts',(5.92940648776744,-22.8871937503747,18.));
#32952=CARTESIAN_POINT('Ctrl Pts',(6.00055830861927,-22.9426681304804,0.));
#32953=CARTESIAN_POINT('Ctrl Pts',(6.00055830861927,-22.9426681304804,18.));
#32954=CARTESIAN_POINT('Ctrl Pts',(6.07219001169362,-22.9978011048904,0.));
#32955=CARTESIAN_POINT('Ctrl Pts',(6.07219001169362,-22.9978011048904,18.));
#32956=CARTESIAN_POINT('Ctrl Pts',(6.14429949537005,-23.0525927424848,0.));
#32957=CARTESIAN_POINT('Ctrl Pts',(6.14429949537005,-23.0525927424848,18.));
#32958=CARTESIAN_POINT('Ctrl Pts',(6.20236818200218,-23.0961532179825,0.));
#32959=CARTESIAN_POINT('Ctrl Pts',(6.20236818200218,-23.0961532179825,18.));
#32960=CARTESIAN_POINT('Ctrl Pts',(6.24613371181766,-23.1286702508203,0.));
#32961=CARTESIAN_POINT('Ctrl Pts',(6.24613371181766,-23.1286702508203,18.));
#32962=CARTESIAN_POINT('Ctrl Pts',(6.27540581784971,-23.1502801515009,0.));
#32963=CARTESIAN_POINT('Ctrl Pts',(6.27540581784971,-23.1502801515009,18.));
#32964=CARTESIAN_POINT('Ctrl Pts',(6.29006564240226,-23.1610680715348,0.));
#32965=CARTESIAN_POINT('Ctrl Pts',(6.29006564240226,-23.1610680715348,18.));
#32966=CARTESIAN_POINT('Ctrl Pts',(2.66302778805429,-18.6042245638953,0.));
#32967=CARTESIAN_POINT('Ctrl Pts',(2.66524945599054,-18.6197453967525,0.));
#32968=CARTESIAN_POINT('Ctrl Pts',(2.67022099202408,-18.6506703537007,0.));
#32969=CARTESIAN_POINT('Ctrl Pts',(2.67926286296661,-18.696707670787,0.));
#32970=CARTESIAN_POINT('Ctrl Pts',(2.69432739305027,-18.7574274222161,0.));
#32971=CARTESIAN_POINT('Ctrl Pts',(2.71724545050994,-18.8324337861517,0.));
#32972=CARTESIAN_POINT('Ctrl Pts',(2.74308150095404,-18.9068127424043,0.));
#32973=CARTESIAN_POINT('Ctrl Pts',(2.77069196504715,-18.980821277801,0.));
#32974=CARTESIAN_POINT('Ctrl Pts',(2.79926206958176,-19.0546365637297,0.));
#32975=CARTESIAN_POINT('Ctrl Pts',(2.828507852372,-19.1283090202125,0.));
#32976=CARTESIAN_POINT('Ctrl Pts',(2.85848240467741,-19.2018091932025,0.));
#32977=CARTESIAN_POINT('Ctrl Pts',(2.88943670541708,-19.2750617358775,0.));
#32978=CARTESIAN_POINT('Ctrl Pts',(2.92166984506915,-19.3479817954251,0.));
#32979=CARTESIAN_POINT('Ctrl Pts',(2.95535900926266,-19.420516469599,0.));
#32980=CARTESIAN_POINT('Ctrl Pts',(2.99048468792079,-19.4926628032527,0.));
#32981=CARTESIAN_POINT('Ctrl Pts',(3.02691741043283,-19.5644460803884,0.));
#32982=CARTESIAN_POINT('Ctrl Pts',(3.06446889170638,-19.635906849522,0.));
#32983=CARTESIAN_POINT('Ctrl Pts',(3.10295238390997,-19.7070857227052,0.));
#32984=CARTESIAN_POINT('Ctrl Pts',(3.1422513957243,-19.7780060327855,0.));
#32985=CARTESIAN_POINT('Ctrl Pts',(3.18233430962982,-19.8486701154397,0.));
#32986=CARTESIAN_POINT('Ctrl Pts',(3.22321820350857,-19.9190683616661,0.));
#32987=CARTESIAN_POINT('Ctrl Pts',(3.26494616363974,-19.9891848794807,0.));
#32988=CARTESIAN_POINT('Ctrl Pts',(3.30756123886962,-20.0590040020604,0.));
#32989=CARTESIAN_POINT('Ctrl Pts',(3.351076475782,-20.1285177769596,0.));
#32990=CARTESIAN_POINT('Ctrl Pts',(3.39547305068767,-20.1977264147619,0.));
#32991=CARTESIAN_POINT('Ctrl Pts',(3.44071459161672,-20.2666346804507,0.));
#32992=CARTESIAN_POINT('Ctrl Pts',(3.48675677306966,-20.3352494700167,0.));
#32993=CARTESIAN_POINT('Ctrl Pts',(3.53355803178954,-20.4035771072894,0.));
#32994=CARTESIAN_POINT('Ctrl Pts',(3.58109188218494,-20.4716202388531,0.));
#32995=CARTESIAN_POINT('Ctrl Pts',(3.62934618720589,-20.5393780076056,0.));
#32996=CARTESIAN_POINT('Ctrl Pts',(3.67831730617887,-20.6068475141781,0.));
#32997=CARTESIAN_POINT('Ctrl Pts',(3.72800579849619,-20.6740248879992,0.));
#32998=CARTESIAN_POINT('Ctrl Pts',(3.77841179839888,-20.740906441832,0.));
#32999=CARTESIAN_POINT('Ctrl Pts',(3.82952970701915,-20.8074899980321,0.));
#33000=CARTESIAN_POINT('Ctrl Pts',(3.88134876172353,-20.8737747416623,0.));
#33001=CARTESIAN_POINT('Ctrl Pts',(3.93385538070582,-20.9397606289993,0.));
#33002=CARTESIAN_POINT('Ctrl Pts',(3.98703495407281,-21.0054479357374,0.));
#33003=CARTESIAN_POINT('Ctrl Pts',(4.04087373166023,-21.0708367812416,0.));
#33004=CARTESIAN_POINT('Ctrl Pts',(4.09536099504429,-21.1359265833073,0.));
#33005=CARTESIAN_POINT('Ctrl Pts',(4.15048873695645,-21.2007161321625,0.));
#33006=CARTESIAN_POINT('Ctrl Pts',(4.20625065101369,-21.2652038365365,0.));
#33007=CARTESIAN_POINT('Ctrl Pts',(4.26264132842711,-21.3293879189372,0.));
#33008=CARTESIAN_POINT('Ctrl Pts',(4.31965542378783,-21.3932666198096,0.));
#33009=CARTESIAN_POINT('Ctrl Pts',(4.37728667813637,-21.4568384368826,0.));
#33010=CARTESIAN_POINT('Ctrl Pts',(4.43552802047029,-21.5201021036274,0.));
#33011=CARTESIAN_POINT('Ctrl Pts',(4.49437199472474,-21.5830564890896,0.));
#33012=CARTESIAN_POINT('Ctrl Pts',(4.55381108432127,-21.6457005243617,0.));
#33013=CARTESIAN_POINT('Ctrl Pts',(4.6138380475249,-21.7080331252945,0.));
#33014=CARTESIAN_POINT('Ctrl Pts',(4.67444631371023,-21.770053106418,0.));
#33015=CARTESIAN_POINT('Ctrl Pts',(4.73562994468575,-21.8317591750867,0.));
#33016=CARTESIAN_POINT('Ctrl Pts',(4.7973834230091,-21.8931499593332,0.));
#33017=CARTESIAN_POINT('Ctrl Pts',(4.85970148585195,-21.954224026919,0.));
#33018=CARTESIAN_POINT('Ctrl Pts',(4.92257895332778,-22.0149799098431,0.));
#33019=CARTESIAN_POINT('Ctrl Pts',(4.98601051193086,-22.0754161299398,0.));
#33020=CARTESIAN_POINT('Ctrl Pts',(5.0499907220168,-22.1355312202693,0.));
#33021=CARTESIAN_POINT('Ctrl Pts',(5.11451415224483,-22.1953237422816,0.));
#33022=CARTESIAN_POINT('Ctrl Pts',(5.17957547700992,-22.2547923093751,0.));
#33023=CARTESIAN_POINT('Ctrl Pts',(5.24516957209272,-22.3139356039553,0.));
#33024=CARTESIAN_POINT('Ctrl Pts',(5.31129163978934,-22.3727524152125,0.));
#33025=CARTESIAN_POINT('Ctrl Pts',(5.37793718711213,-22.4312416086453,0.));
#33026=CARTESIAN_POINT('Ctrl Pts',(5.44510186987254,-22.4894020366778,0.));
#33027=CARTESIAN_POINT('Ctrl Pts',(5.51278136258485,-22.5472324623564,0.));
#33028=CARTESIAN_POINT('Ctrl Pts',(5.58097123210075,-22.6047314918151,0.));
#33029=CARTESIAN_POINT('Ctrl Pts',(5.64966676217478,-22.6618974767817,0.));
#33030=CARTESIAN_POINT('Ctrl Pts',(5.71886294543539,-22.7187285302677,0.));
#33031=CARTESIAN_POINT('Ctrl Pts',(5.7885547640031,-22.7752227318719,0.));
#33032=CARTESIAN_POINT('Ctrl Pts',(5.85873740439746,-22.8313782965033,0.));
#33033=CARTESIAN_POINT('Ctrl Pts',(5.92940648776744,-22.8871937503747,0.));
#33034=CARTESIAN_POINT('Ctrl Pts',(6.00055830861927,-22.9426681304804,0.));
#33035=CARTESIAN_POINT('Ctrl Pts',(6.08651635230849,-23.0088276997724,0.));
#33036=CARTESIAN_POINT('Ctrl Pts',(6.15874528113544,-23.0635340031629,0.));
#33037=CARTESIAN_POINT('Ctrl Pts',(6.21690914895776,-23.107026289589,0.));
#33038=CARTESIAN_POINT('Ctrl Pts',(6.26074599324761,-23.1394922314359,0.));
#33039=CARTESIAN_POINT('Ctrl Pts',(6.29006564240226,-23.1610680715348,0.));
#33040=CARTESIAN_POINT('Ctrl Pts',(2.66302778805429,-18.6042245638953,15.));
#33041=CARTESIAN_POINT('Ctrl Pts',(2.66524945599054,-18.6197453967525,15.));
#33042=CARTESIAN_POINT('Ctrl Pts',(2.67022099202408,-18.6506703537007,15.));
#33043=CARTESIAN_POINT('Ctrl Pts',(2.67926286296661,-18.696707670787,15.));
#33044=CARTESIAN_POINT('Ctrl Pts',(2.69432739305027,-18.7574274222161,15.));
#33045=CARTESIAN_POINT('Ctrl Pts',(2.71724545050994,-18.8324337861517,15.));
#33046=CARTESIAN_POINT('Ctrl Pts',(2.74308150095404,-18.9068127424043,15.));
#33047=CARTESIAN_POINT('Ctrl Pts',(2.77069196504715,-18.980821277801,15.));
#33048=CARTESIAN_POINT('Ctrl Pts',(2.79926206958176,-19.0546365637297,15.));
#33049=CARTESIAN_POINT('Ctrl Pts',(2.828507852372,-19.1283090202125,15.));
#33050=CARTESIAN_POINT('Ctrl Pts',(2.85848240467741,-19.2018091932025,15.));
#33051=CARTESIAN_POINT('Ctrl Pts',(2.88943670541708,-19.2750617358775,15.));
#33052=CARTESIAN_POINT('Ctrl Pts',(2.92166984506915,-19.3479817954251,15.));
#33053=CARTESIAN_POINT('Ctrl Pts',(2.95535900926266,-19.420516469599,15.));
#33054=CARTESIAN_POINT('Ctrl Pts',(2.99048468792079,-19.4926628032527,15.));
#33055=CARTESIAN_POINT('Ctrl Pts',(3.02691741043283,-19.5644460803884,15.));
#33056=CARTESIAN_POINT('Ctrl Pts',(3.06446889170638,-19.635906849522,15.));
#33057=CARTESIAN_POINT('Ctrl Pts',(3.10295238390997,-19.7070857227052,15.));
#33058=CARTESIAN_POINT('Ctrl Pts',(3.1422513957243,-19.7780060327855,15.));
#33059=CARTESIAN_POINT('Ctrl Pts',(3.18233430962982,-19.8486701154397,15.));
#33060=CARTESIAN_POINT('Ctrl Pts',(3.22321820350857,-19.9190683616661,15.));
#33061=CARTESIAN_POINT('Ctrl Pts',(3.26494616363974,-19.9891848794807,15.));
#33062=CARTESIAN_POINT('Ctrl Pts',(3.30756123886962,-20.0590040020604,15.));
#33063=CARTESIAN_POINT('Ctrl Pts',(3.351076475782,-20.1285177769596,15.));
#33064=CARTESIAN_POINT('Ctrl Pts',(3.39547305068767,-20.1977264147619,15.));
#33065=CARTESIAN_POINT('Ctrl Pts',(3.44071459161672,-20.2666346804507,15.));
#33066=CARTESIAN_POINT('Ctrl Pts',(3.48675677306966,-20.3352494700167,15.));
#33067=CARTESIAN_POINT('Ctrl Pts',(3.53355803178954,-20.4035771072894,15.));
#33068=CARTESIAN_POINT('Ctrl Pts',(3.58109188218494,-20.4716202388531,15.));
#33069=CARTESIAN_POINT('Ctrl Pts',(3.62934618720589,-20.5393780076056,15.));
#33070=CARTESIAN_POINT('Ctrl Pts',(3.67831730617887,-20.6068475141781,15.));
#33071=CARTESIAN_POINT('Ctrl Pts',(3.72800579849619,-20.6740248879992,15.));
#33072=CARTESIAN_POINT('Ctrl Pts',(3.77841179839888,-20.740906441832,15.));
#33073=CARTESIAN_POINT('Ctrl Pts',(3.82952970701915,-20.8074899980321,15.));
#33074=CARTESIAN_POINT('Ctrl Pts',(3.88134876172353,-20.8737747416623,15.));
#33075=CARTESIAN_POINT('Ctrl Pts',(3.93385538070582,-20.9397606289993,15.));
#33076=CARTESIAN_POINT('Ctrl Pts',(3.98703495407281,-21.0054479357374,15.));
#33077=CARTESIAN_POINT('Ctrl Pts',(4.04087373166023,-21.0708367812416,15.));
#33078=CARTESIAN_POINT('Ctrl Pts',(4.09536099504429,-21.1359265833073,15.));
#33079=CARTESIAN_POINT('Ctrl Pts',(4.15048873695645,-21.2007161321625,15.));
#33080=CARTESIAN_POINT('Ctrl Pts',(4.20625065101369,-21.2652038365365,15.));
#33081=CARTESIAN_POINT('Ctrl Pts',(4.26264132842711,-21.3293879189372,15.));
#33082=CARTESIAN_POINT('Ctrl Pts',(4.31965542378783,-21.3932666198096,15.));
#33083=CARTESIAN_POINT('Ctrl Pts',(4.37728667813637,-21.4568384368826,15.));
#33084=CARTESIAN_POINT('Ctrl Pts',(4.43552802047029,-21.5201021036274,15.));
#33085=CARTESIAN_POINT('Ctrl Pts',(4.49437199472474,-21.5830564890896,15.));
#33086=CARTESIAN_POINT('Ctrl Pts',(4.55381108432127,-21.6457005243617,15.));
#33087=CARTESIAN_POINT('Ctrl Pts',(4.6138380475249,-21.7080331252945,15.));
#33088=CARTESIAN_POINT('Ctrl Pts',(4.67444631371023,-21.770053106418,15.));
#33089=CARTESIAN_POINT('Ctrl Pts',(4.73562994468575,-21.8317591750867,15.));
#33090=CARTESIAN_POINT('Ctrl Pts',(4.7973834230091,-21.8931499593332,15.));
#33091=CARTESIAN_POINT('Ctrl Pts',(4.85970148585195,-21.954224026919,15.));
#33092=CARTESIAN_POINT('Ctrl Pts',(4.92257895332778,-22.0149799098431,15.));
#33093=CARTESIAN_POINT('Ctrl Pts',(4.98601051193086,-22.0754161299398,15.));
#33094=CARTESIAN_POINT('Ctrl Pts',(5.0499907220168,-22.1355312202693,15.));
#33095=CARTESIAN_POINT('Ctrl Pts',(5.11451415224483,-22.1953237422816,15.));
#33096=CARTESIAN_POINT('Ctrl Pts',(5.17957547700992,-22.2547923093751,15.));
#33097=CARTESIAN_POINT('Ctrl Pts',(5.24516957209272,-22.3139356039553,15.));
#33098=CARTESIAN_POINT('Ctrl Pts',(5.31129163978934,-22.3727524152125,15.));
#33099=CARTESIAN_POINT('Ctrl Pts',(5.37793718711213,-22.4312416086453,15.));
#33100=CARTESIAN_POINT('Ctrl Pts',(5.44510186987254,-22.4894020366778,15.));
#33101=CARTESIAN_POINT('Ctrl Pts',(5.51278136258485,-22.5472324623564,15.));
#33102=CARTESIAN_POINT('Ctrl Pts',(5.58097123210075,-22.6047314918151,15.));
#33103=CARTESIAN_POINT('Ctrl Pts',(5.64966676217478,-22.6618974767817,15.));
#33104=CARTESIAN_POINT('Ctrl Pts',(5.71886294543539,-22.7187285302677,15.));
#33105=CARTESIAN_POINT('Ctrl Pts',(5.7885547640031,-22.7752227318719,15.));
#33106=CARTESIAN_POINT('Ctrl Pts',(5.85873740439746,-22.8313782965033,15.));
#33107=CARTESIAN_POINT('Ctrl Pts',(5.92940648776744,-22.8871937503747,15.));
#33108=CARTESIAN_POINT('Ctrl Pts',(6.00055830861927,-22.9426681304804,15.));
#33109=CARTESIAN_POINT('Ctrl Pts',(6.08651635230849,-23.0088276997724,15.));
#33110=CARTESIAN_POINT('Ctrl Pts',(6.15874528113544,-23.0635340031629,15.));
#33111=CARTESIAN_POINT('Ctrl Pts',(6.21690914895776,-23.107026289589,15.));
#33112=CARTESIAN_POINT('Ctrl Pts',(6.26074599324761,-23.1394922314359,15.));
#33113=CARTESIAN_POINT('Ctrl Pts',(6.29006564240226,-23.1610680715348,15.));
#33114=CARTESIAN_POINT('Ctrl Pts',(-6.29006564240227,-23.1610680715348,
0.));
#33115=CARTESIAN_POINT('Ctrl Pts',(-6.29006564240227,-23.1610680715348,
18.));
#33116=CARTESIAN_POINT('Ctrl Pts',(-6.27540581784972,-23.1502801515009,
0.));
#33117=CARTESIAN_POINT('Ctrl Pts',(-6.27540581784972,-23.1502801515009,
18.));
#33118=CARTESIAN_POINT('Ctrl Pts',(-6.24613371181767,-23.1286702508203,
0.));
#33119=CARTESIAN_POINT('Ctrl Pts',(-6.24613371181767,-23.1286702508203,
18.));
#33120=CARTESIAN_POINT('Ctrl Pts',(-6.20236818200219,-23.0961532179825,
0.));
#33121=CARTESIAN_POINT('Ctrl Pts',(-6.20236818200219,-23.0961532179825,
18.));
#33122=CARTESIAN_POINT('Ctrl Pts',(-6.14429949537005,-23.0525927424848,
0.));
#33123=CARTESIAN_POINT('Ctrl Pts',(-6.14429949537005,-23.0525927424848,
18.));
#33124=CARTESIAN_POINT('Ctrl Pts',(-6.07219001169363,-22.9978011048904,
0.));
#33125=CARTESIAN_POINT('Ctrl Pts',(-6.07219001169363,-22.9978011048904,
18.));
#33126=CARTESIAN_POINT('Ctrl Pts',(-6.00055830861928,-22.9426681304804,
0.));
#33127=CARTESIAN_POINT('Ctrl Pts',(-6.00055830861928,-22.9426681304804,
18.));
#33128=CARTESIAN_POINT('Ctrl Pts',(-5.92940648776744,-22.8871937503747,
0.));
#33129=CARTESIAN_POINT('Ctrl Pts',(-5.92940648776744,-22.8871937503747,
18.));
#33130=CARTESIAN_POINT('Ctrl Pts',(-5.85873740439747,-22.8313782965033,
0.));
#33131=CARTESIAN_POINT('Ctrl Pts',(-5.85873740439747,-22.8313782965033,
18.));
#33132=CARTESIAN_POINT('Ctrl Pts',(-5.78855476400311,-22.7752227318719,
0.));
#33133=CARTESIAN_POINT('Ctrl Pts',(-5.78855476400311,-22.7752227318719,
18.));
#33134=CARTESIAN_POINT('Ctrl Pts',(-5.71886294543539,-22.7187285302677,
0.));
#33135=CARTESIAN_POINT('Ctrl Pts',(-5.71886294543539,-22.7187285302677,
18.));
#33136=CARTESIAN_POINT('Ctrl Pts',(-5.64966676217478,-22.6618974767817,
0.));
#33137=CARTESIAN_POINT('Ctrl Pts',(-5.64966676217478,-22.6618974767817,
18.));
#33138=CARTESIAN_POINT('Ctrl Pts',(-5.58097123210075,-22.6047314918152,
0.));
#33139=CARTESIAN_POINT('Ctrl Pts',(-5.58097123210075,-22.6047314918152,
18.));
#33140=CARTESIAN_POINT('Ctrl Pts',(-5.51278136258486,-22.5472324623564,
0.));
#33141=CARTESIAN_POINT('Ctrl Pts',(-5.51278136258486,-22.5472324623564,
18.));
#33142=CARTESIAN_POINT('Ctrl Pts',(-5.44510186987254,-22.4894020366778,
0.));
#33143=CARTESIAN_POINT('Ctrl Pts',(-5.44510186987254,-22.4894020366778,
18.));
#33144=CARTESIAN_POINT('Ctrl Pts',(-5.37793718711213,-22.4312416086453,
0.));
#33145=CARTESIAN_POINT('Ctrl Pts',(-5.37793718711213,-22.4312416086453,
18.));
#33146=CARTESIAN_POINT('Ctrl Pts',(-5.31129163978934,-22.3727524152125,
0.));
#33147=CARTESIAN_POINT('Ctrl Pts',(-5.31129163978934,-22.3727524152125,
18.));
#33148=CARTESIAN_POINT('Ctrl Pts',(-5.24516957209273,-22.3139356039553,
0.));
#33149=CARTESIAN_POINT('Ctrl Pts',(-5.24516957209273,-22.3139356039553,
18.));
#33150=CARTESIAN_POINT('Ctrl Pts',(-5.17957547700993,-22.2547923093751,
0.));
#33151=CARTESIAN_POINT('Ctrl Pts',(-5.17957547700993,-22.2547923093751,
18.));
#33152=CARTESIAN_POINT('Ctrl Pts',(-5.11451415224484,-22.1953237422816,
0.));
#33153=CARTESIAN_POINT('Ctrl Pts',(-5.11451415224484,-22.1953237422816,
18.));
#33154=CARTESIAN_POINT('Ctrl Pts',(-5.04999072201681,-22.1355312202693,
0.));
#33155=CARTESIAN_POINT('Ctrl Pts',(-5.04999072201681,-22.1355312202693,
18.));
#33156=CARTESIAN_POINT('Ctrl Pts',(-4.98601051193087,-22.0754161299398,
0.));
#33157=CARTESIAN_POINT('Ctrl Pts',(-4.98601051193087,-22.0754161299398,
18.));
#33158=CARTESIAN_POINT('Ctrl Pts',(-4.92257895332779,-22.0149799098431,
0.));
#33159=CARTESIAN_POINT('Ctrl Pts',(-4.92257895332779,-22.0149799098431,
18.));
#33160=CARTESIAN_POINT('Ctrl Pts',(-4.85970148585196,-21.9542240269191,
0.));
#33161=CARTESIAN_POINT('Ctrl Pts',(-4.85970148585196,-21.9542240269191,
18.));
#33162=CARTESIAN_POINT('Ctrl Pts',(-4.7973834230091,-21.8931499593332,0.));
#33163=CARTESIAN_POINT('Ctrl Pts',(-4.7973834230091,-21.8931499593332,18.));
#33164=CARTESIAN_POINT('Ctrl Pts',(-4.73562994468575,-21.8317591750867,
0.));
#33165=CARTESIAN_POINT('Ctrl Pts',(-4.73562994468575,-21.8317591750867,
18.));
#33166=CARTESIAN_POINT('Ctrl Pts',(-4.67444631371023,-21.770053106418,0.));
#33167=CARTESIAN_POINT('Ctrl Pts',(-4.67444631371023,-21.770053106418,18.));
#33168=CARTESIAN_POINT('Ctrl Pts',(-4.6138380475249,-21.7080331252945,0.));
#33169=CARTESIAN_POINT('Ctrl Pts',(-4.6138380475249,-21.7080331252945,18.));
#33170=CARTESIAN_POINT('Ctrl Pts',(-4.55381108432127,-21.6457005243617,
0.));
#33171=CARTESIAN_POINT('Ctrl Pts',(-4.55381108432127,-21.6457005243617,
18.));
#33172=CARTESIAN_POINT('Ctrl Pts',(-4.49437199472475,-21.5830564890896,
0.));
#33173=CARTESIAN_POINT('Ctrl Pts',(-4.49437199472475,-21.5830564890896,
18.));
#33174=CARTESIAN_POINT('Ctrl Pts',(-4.4355280204703,-21.5201021036274,0.));
#33175=CARTESIAN_POINT('Ctrl Pts',(-4.4355280204703,-21.5201021036274,18.));
#33176=CARTESIAN_POINT('Ctrl Pts',(-4.37728667813637,-21.4568384368826,
0.));
#33177=CARTESIAN_POINT('Ctrl Pts',(-4.37728667813637,-21.4568384368826,
18.));
#33178=CARTESIAN_POINT('Ctrl Pts',(-4.31965542378783,-21.3932666198096,
0.));
#33179=CARTESIAN_POINT('Ctrl Pts',(-4.31965542378783,-21.3932666198096,
18.));
#33180=CARTESIAN_POINT('Ctrl Pts',(-4.26264132842712,-21.3293879189372,
0.));
#33181=CARTESIAN_POINT('Ctrl Pts',(-4.26264132842712,-21.3293879189372,
18.));
#33182=CARTESIAN_POINT('Ctrl Pts',(-4.20625065101369,-21.2652038365365,
0.));
#33183=CARTESIAN_POINT('Ctrl Pts',(-4.20625065101369,-21.2652038365365,
18.));
#33184=CARTESIAN_POINT('Ctrl Pts',(-4.15048873695646,-21.2007161321625,
0.));
#33185=CARTESIAN_POINT('Ctrl Pts',(-4.15048873695646,-21.2007161321625,
18.));
#33186=CARTESIAN_POINT('Ctrl Pts',(-4.09536099504429,-21.1359265833073,
0.));
#33187=CARTESIAN_POINT('Ctrl Pts',(-4.09536099504429,-21.1359265833073,
18.));
#33188=CARTESIAN_POINT('Ctrl Pts',(-4.04087373166023,-21.0708367812416,
0.));
#33189=CARTESIAN_POINT('Ctrl Pts',(-4.04087373166023,-21.0708367812416,
18.));
#33190=CARTESIAN_POINT('Ctrl Pts',(-3.98703495407281,-21.0054479357374,
0.));
#33191=CARTESIAN_POINT('Ctrl Pts',(-3.98703495407281,-21.0054479357374,
18.));
#33192=CARTESIAN_POINT('Ctrl Pts',(-3.93385538070582,-20.9397606289993,
0.));
#33193=CARTESIAN_POINT('Ctrl Pts',(-3.93385538070582,-20.9397606289993,
18.));
#33194=CARTESIAN_POINT('Ctrl Pts',(-3.88134876172354,-20.8737747416623,
0.));
#33195=CARTESIAN_POINT('Ctrl Pts',(-3.88134876172354,-20.8737747416623,
18.));
#33196=CARTESIAN_POINT('Ctrl Pts',(-3.82952970701916,-20.8074899980321,
0.));
#33197=CARTESIAN_POINT('Ctrl Pts',(-3.82952970701916,-20.8074899980321,
18.));
#33198=CARTESIAN_POINT('Ctrl Pts',(-3.77841179839888,-20.740906441832,0.));
#33199=CARTESIAN_POINT('Ctrl Pts',(-3.77841179839888,-20.740906441832,18.));
#33200=CARTESIAN_POINT('Ctrl Pts',(-3.7280057984962,-20.6740248879992,0.));
#33201=CARTESIAN_POINT('Ctrl Pts',(-3.7280057984962,-20.6740248879992,18.));
#33202=CARTESIAN_POINT('Ctrl Pts',(-3.67831730617888,-20.6068475141781,
0.));
#33203=CARTESIAN_POINT('Ctrl Pts',(-3.67831730617888,-20.6068475141781,
18.));
#33204=CARTESIAN_POINT('Ctrl Pts',(-3.6293461872059,-20.5393780076057,0.));
#33205=CARTESIAN_POINT('Ctrl Pts',(-3.6293461872059,-20.5393780076057,18.));
#33206=CARTESIAN_POINT('Ctrl Pts',(-3.58109188218494,-20.4716202388531,
0.));
#33207=CARTESIAN_POINT('Ctrl Pts',(-3.58109188218494,-20.4716202388531,
18.));
#33208=CARTESIAN_POINT('Ctrl Pts',(-3.53355803178955,-20.4035771072894,
0.));
#33209=CARTESIAN_POINT('Ctrl Pts',(-3.53355803178955,-20.4035771072894,
18.));
#33210=CARTESIAN_POINT('Ctrl Pts',(-3.48675677306967,-20.3352494700167,
0.));
#33211=CARTESIAN_POINT('Ctrl Pts',(-3.48675677306967,-20.3352494700167,
18.));
#33212=CARTESIAN_POINT('Ctrl Pts',(-3.44071459161672,-20.2666346804507,
0.));
#33213=CARTESIAN_POINT('Ctrl Pts',(-3.44071459161672,-20.2666346804507,
18.));
#33214=CARTESIAN_POINT('Ctrl Pts',(-3.39547305068768,-20.1977264147619,
0.));
#33215=CARTESIAN_POINT('Ctrl Pts',(-3.39547305068768,-20.1977264147619,
18.));
#33216=CARTESIAN_POINT('Ctrl Pts',(-3.35107647578201,-20.1285177769596,
0.));
#33217=CARTESIAN_POINT('Ctrl Pts',(-3.35107647578201,-20.1285177769596,
18.));
#33218=CARTESIAN_POINT('Ctrl Pts',(-3.30756123886962,-20.0590040020604,
0.));
#33219=CARTESIAN_POINT('Ctrl Pts',(-3.30756123886962,-20.0590040020604,
18.));
#33220=CARTESIAN_POINT('Ctrl Pts',(-3.26494616363974,-19.9891848794807,
0.));
#33221=CARTESIAN_POINT('Ctrl Pts',(-3.26494616363974,-19.9891848794807,
18.));
#33222=CARTESIAN_POINT('Ctrl Pts',(-3.22321820350857,-19.9190683616661,
0.));
#33223=CARTESIAN_POINT('Ctrl Pts',(-3.22321820350857,-19.9190683616661,
18.));
#33224=CARTESIAN_POINT('Ctrl Pts',(-3.18233430962982,-19.8486701154397,
0.));
#33225=CARTESIAN_POINT('Ctrl Pts',(-3.18233430962982,-19.8486701154397,
18.));
#33226=CARTESIAN_POINT('Ctrl Pts',(-3.14225139572431,-19.7780060327855,
0.));
#33227=CARTESIAN_POINT('Ctrl Pts',(-3.14225139572431,-19.7780060327855,
18.));
#33228=CARTESIAN_POINT('Ctrl Pts',(-3.10295238390997,-19.7070857227052,
0.));
#33229=CARTESIAN_POINT('Ctrl Pts',(-3.10295238390997,-19.7070857227052,
18.));
#33230=CARTESIAN_POINT('Ctrl Pts',(-3.06446889170638,-19.635906849522,0.));
#33231=CARTESIAN_POINT('Ctrl Pts',(-3.06446889170638,-19.635906849522,18.));
#33232=CARTESIAN_POINT('Ctrl Pts',(-3.02691741043284,-19.5644460803884,
0.));
#33233=CARTESIAN_POINT('Ctrl Pts',(-3.02691741043284,-19.5644460803884,
18.));
#33234=CARTESIAN_POINT('Ctrl Pts',(-2.99048468792079,-19.4926628032527,
0.));
#33235=CARTESIAN_POINT('Ctrl Pts',(-2.99048468792079,-19.4926628032527,
18.));
#33236=CARTESIAN_POINT('Ctrl Pts',(-2.95535900926266,-19.420516469599,0.));
#33237=CARTESIAN_POINT('Ctrl Pts',(-2.95535900926266,-19.420516469599,18.));
#33238=CARTESIAN_POINT('Ctrl Pts',(-2.92166984506916,-19.3479817954251,
0.));
#33239=CARTESIAN_POINT('Ctrl Pts',(-2.92166984506916,-19.3479817954251,
18.));
#33240=CARTESIAN_POINT('Ctrl Pts',(-2.88943670541709,-19.2750617358775,
0.));
#33241=CARTESIAN_POINT('Ctrl Pts',(-2.88943670541709,-19.2750617358775,
18.));
#33242=CARTESIAN_POINT('Ctrl Pts',(-2.85848240467742,-19.2018091932025,
0.));
#33243=CARTESIAN_POINT('Ctrl Pts',(-2.85848240467742,-19.2018091932025,
18.));
#33244=CARTESIAN_POINT('Ctrl Pts',(-2.828507852372,-19.1283090202125,0.));
#33245=CARTESIAN_POINT('Ctrl Pts',(-2.828507852372,-19.1283090202125,18.));
#33246=CARTESIAN_POINT('Ctrl Pts',(-2.79926206958176,-19.0546365637297,
0.));
#33247=CARTESIAN_POINT('Ctrl Pts',(-2.79926206958176,-19.0546365637297,
18.));
#33248=CARTESIAN_POINT('Ctrl Pts',(-2.77069196504715,-18.980821277801,0.));
#33249=CARTESIAN_POINT('Ctrl Pts',(-2.77069196504715,-18.980821277801,18.));
#33250=CARTESIAN_POINT('Ctrl Pts',(-2.74308150095405,-18.9068127424043,
0.));
#33251=CARTESIAN_POINT('Ctrl Pts',(-2.74308150095405,-18.9068127424043,
18.));
#33252=CARTESIAN_POINT('Ctrl Pts',(-2.71724545050995,-18.8324337861517,
0.));
#33253=CARTESIAN_POINT('Ctrl Pts',(-2.71724545050995,-18.8324337861517,
18.));
#33254=CARTESIAN_POINT('Ctrl Pts',(-2.69432739305028,-18.7574274222161,
0.));
#33255=CARTESIAN_POINT('Ctrl Pts',(-2.69432739305028,-18.7574274222161,
18.));
#33256=CARTESIAN_POINT('Ctrl Pts',(-2.67926286296662,-18.696707670787,0.));
#33257=CARTESIAN_POINT('Ctrl Pts',(-2.67926286296662,-18.696707670787,18.));
#33258=CARTESIAN_POINT('Ctrl Pts',(-2.67022099202409,-18.6506703537007,
0.));
#33259=CARTESIAN_POINT('Ctrl Pts',(-2.67022099202409,-18.6506703537007,
18.));
#33260=CARTESIAN_POINT('Ctrl Pts',(-2.66524945599055,-18.6197453967525,
0.));
#33261=CARTESIAN_POINT('Ctrl Pts',(-2.66524945599055,-18.6197453967525,
18.));
#33262=CARTESIAN_POINT('Ctrl Pts',(-2.6630277880543,-18.6042245638953,0.));
#33263=CARTESIAN_POINT('Ctrl Pts',(-2.6630277880543,-18.6042245638953,18.));
#33264=CARTESIAN_POINT('',(-6.29006564240232,-23.1610680715348,0.));
#33265=CARTESIAN_POINT('Ctrl Pts',(-2.6630277880543,-18.6042245638953,0.));
#33266=CARTESIAN_POINT('Ctrl Pts',(-2.66524945599055,-18.6197453967525,
0.));
#33267=CARTESIAN_POINT('Ctrl Pts',(-2.67022099202409,-18.6506703537007,
0.));
#33268=CARTESIAN_POINT('Ctrl Pts',(-2.67926286296662,-18.696707670787,0.));
#33269=CARTESIAN_POINT('Ctrl Pts',(-2.69432739305028,-18.7574274222161,
0.));
#33270=CARTESIAN_POINT('Ctrl Pts',(-2.71724545050995,-18.8324337861517,
0.));
#33271=CARTESIAN_POINT('Ctrl Pts',(-2.74308150095405,-18.9068127424043,
0.));
#33272=CARTESIAN_POINT('Ctrl Pts',(-2.77069196504715,-18.980821277801,0.));
#33273=CARTESIAN_POINT('Ctrl Pts',(-2.79926206958176,-19.0546365637297,
0.));
#33274=CARTESIAN_POINT('Ctrl Pts',(-2.828507852372,-19.1283090202125,0.));
#33275=CARTESIAN_POINT('Ctrl Pts',(-2.85848240467742,-19.2018091932025,
0.));
#33276=CARTESIAN_POINT('Ctrl Pts',(-2.88943670541709,-19.2750617358775,
0.));
#33277=CARTESIAN_POINT('Ctrl Pts',(-2.92166984506916,-19.3479817954251,
0.));
#33278=CARTESIAN_POINT('Ctrl Pts',(-2.95535900926266,-19.420516469599,0.));
#33279=CARTESIAN_POINT('Ctrl Pts',(-2.99048468792079,-19.4926628032527,
0.));
#33280=CARTESIAN_POINT('Ctrl Pts',(-3.02691741043284,-19.5644460803884,
0.));
#33281=CARTESIAN_POINT('Ctrl Pts',(-3.06446889170638,-19.635906849522,0.));
#33282=CARTESIAN_POINT('Ctrl Pts',(-3.10295238390997,-19.7070857227052,
0.));
#33283=CARTESIAN_POINT('Ctrl Pts',(-3.14225139572431,-19.7780060327855,
0.));
#33284=CARTESIAN_POINT('Ctrl Pts',(-3.18233430962982,-19.8486701154397,
0.));
#33285=CARTESIAN_POINT('Ctrl Pts',(-3.22321820350857,-19.9190683616661,
0.));
#33286=CARTESIAN_POINT('Ctrl Pts',(-3.26494616363974,-19.9891848794807,
0.));
#33287=CARTESIAN_POINT('Ctrl Pts',(-3.30756123886962,-20.0590040020604,
0.));
#33288=CARTESIAN_POINT('Ctrl Pts',(-3.35107647578201,-20.1285177769596,
0.));
#33289=CARTESIAN_POINT('Ctrl Pts',(-3.39547305068768,-20.1977264147619,
0.));
#33290=CARTESIAN_POINT('Ctrl Pts',(-3.44071459161672,-20.2666346804507,
0.));
#33291=CARTESIAN_POINT('Ctrl Pts',(-3.48675677306967,-20.3352494700167,
0.));
#33292=CARTESIAN_POINT('Ctrl Pts',(-3.53355803178955,-20.4035771072894,
0.));
#33293=CARTESIAN_POINT('Ctrl Pts',(-3.58109188218494,-20.4716202388531,
0.));
#33294=CARTESIAN_POINT('Ctrl Pts',(-3.6293461872059,-20.5393780076057,0.));
#33295=CARTESIAN_POINT('Ctrl Pts',(-3.67831730617888,-20.6068475141781,
0.));
#33296=CARTESIAN_POINT('Ctrl Pts',(-3.7280057984962,-20.6740248879992,0.));
#33297=CARTESIAN_POINT('Ctrl Pts',(-3.77841179839888,-20.740906441832,0.));
#33298=CARTESIAN_POINT('Ctrl Pts',(-3.82952970701916,-20.8074899980321,
0.));
#33299=CARTESIAN_POINT('Ctrl Pts',(-3.88134876172354,-20.8737747416623,
0.));
#33300=CARTESIAN_POINT('Ctrl Pts',(-3.93385538070582,-20.9397606289993,
0.));
#33301=CARTESIAN_POINT('Ctrl Pts',(-3.98703495407281,-21.0054479357374,
0.));
#33302=CARTESIAN_POINT('Ctrl Pts',(-4.04087373166023,-21.0708367812416,
0.));
#33303=CARTESIAN_POINT('Ctrl Pts',(-4.09536099504429,-21.1359265833073,
0.));
#33304=CARTESIAN_POINT('Ctrl Pts',(-4.15048873695646,-21.2007161321625,
0.));
#33305=CARTESIAN_POINT('Ctrl Pts',(-4.20625065101369,-21.2652038365365,
0.));
#33306=CARTESIAN_POINT('Ctrl Pts',(-4.26264132842712,-21.3293879189372,
0.));
#33307=CARTESIAN_POINT('Ctrl Pts',(-4.31965542378783,-21.3932666198096,
0.));
#33308=CARTESIAN_POINT('Ctrl Pts',(-4.37728667813637,-21.4568384368826,
0.));
#33309=CARTESIAN_POINT('Ctrl Pts',(-4.4355280204703,-21.5201021036274,0.));
#33310=CARTESIAN_POINT('Ctrl Pts',(-4.49437199472475,-21.5830564890896,
0.));
#33311=CARTESIAN_POINT('Ctrl Pts',(-4.55381108432127,-21.6457005243617,
0.));
#33312=CARTESIAN_POINT('Ctrl Pts',(-4.6138380475249,-21.7080331252945,0.));
#33313=CARTESIAN_POINT('Ctrl Pts',(-4.67444631371023,-21.770053106418,0.));
#33314=CARTESIAN_POINT('Ctrl Pts',(-4.73562994468575,-21.8317591750867,
0.));
#33315=CARTESIAN_POINT('Ctrl Pts',(-4.7973834230091,-21.8931499593332,0.));
#33316=CARTESIAN_POINT('Ctrl Pts',(-4.85970148585196,-21.9542240269191,
0.));
#33317=CARTESIAN_POINT('Ctrl Pts',(-4.92257895332779,-22.0149799098431,
0.));
#33318=CARTESIAN_POINT('Ctrl Pts',(-4.98601051193087,-22.0754161299398,
0.));
#33319=CARTESIAN_POINT('Ctrl Pts',(-5.04999072201681,-22.1355312202693,
0.));
#33320=CARTESIAN_POINT('Ctrl Pts',(-5.11451415224484,-22.1953237422816,
0.));
#33321=CARTESIAN_POINT('Ctrl Pts',(-5.17957547700993,-22.2547923093751,
0.));
#33322=CARTESIAN_POINT('Ctrl Pts',(-5.24516957209273,-22.3139356039553,
0.));
#33323=CARTESIAN_POINT('Ctrl Pts',(-5.31129163978934,-22.3727524152125,
0.));
#33324=CARTESIAN_POINT('Ctrl Pts',(-5.37793718711213,-22.4312416086453,
0.));
#33325=CARTESIAN_POINT('Ctrl Pts',(-5.44510186987254,-22.4894020366778,
0.));
#33326=CARTESIAN_POINT('Ctrl Pts',(-5.51278136258486,-22.5472324623564,
0.));
#33327=CARTESIAN_POINT('Ctrl Pts',(-5.58097123210075,-22.6047314918152,
0.));
#33328=CARTESIAN_POINT('Ctrl Pts',(-5.64966676217478,-22.6618974767817,
0.));
#33329=CARTESIAN_POINT('Ctrl Pts',(-5.71886294543539,-22.7187285302677,
0.));
#33330=CARTESIAN_POINT('Ctrl Pts',(-5.78855476400311,-22.7752227318719,
0.));
#33331=CARTESIAN_POINT('Ctrl Pts',(-5.85873740439747,-22.8313782965033,
0.));
#33332=CARTESIAN_POINT('Ctrl Pts',(-5.92940648776744,-22.8871937503747,
0.));
#33333=CARTESIAN_POINT('Ctrl Pts',(-6.00055830861928,-22.9426681304804,
0.));
#33334=CARTESIAN_POINT('Ctrl Pts',(-6.0865163523085,-23.0088276997724,0.));
#33335=CARTESIAN_POINT('Ctrl Pts',(-6.15874528113544,-23.0635340031629,
0.));
#33336=CARTESIAN_POINT('Ctrl Pts',(-6.21690914895778,-23.107026289589,0.));
#33337=CARTESIAN_POINT('Ctrl Pts',(-6.26074599324762,-23.1394922314359,
0.));
#33338=CARTESIAN_POINT('Ctrl Pts',(-6.29006564240227,-23.1610680715348,
0.));
#33339=CARTESIAN_POINT('',(-6.29006564240232,-23.1610680715348,15.));
#33340=CARTESIAN_POINT('Ctrl Pts',(-6.29006564240227,-23.1610680715348,
15.));
#33341=CARTESIAN_POINT('Ctrl Pts',(-6.27540581784972,-23.1502801515009,
15.));
#33342=CARTESIAN_POINT('Ctrl Pts',(-6.24613371181767,-23.1286702508203,
15.));
#33343=CARTESIAN_POINT('Ctrl Pts',(-6.20236818200219,-23.0961532179825,
15.));
#33344=CARTESIAN_POINT('Ctrl Pts',(-6.14429949537005,-23.0525927424848,
15.));
#33345=CARTESIAN_POINT('Ctrl Pts',(-6.07219001169363,-22.9978011048904,
15.));
#33346=CARTESIAN_POINT('Ctrl Pts',(-6.00055830861928,-22.9426681304804,
15.));
#33347=CARTESIAN_POINT('Ctrl Pts',(-5.92940648776744,-22.8871937503747,
15.));
#33348=CARTESIAN_POINT('Ctrl Pts',(-5.85873740439747,-22.8313782965033,
15.));
#33349=CARTESIAN_POINT('Ctrl Pts',(-5.78855476400311,-22.7752227318719,
15.));
#33350=CARTESIAN_POINT('Ctrl Pts',(-5.71886294543539,-22.7187285302677,
15.));
#33351=CARTESIAN_POINT('Ctrl Pts',(-5.64966676217478,-22.6618974767817,
15.));
#33352=CARTESIAN_POINT('Ctrl Pts',(-5.58097123210075,-22.6047314918152,
15.));
#33353=CARTESIAN_POINT('Ctrl Pts',(-5.51278136258486,-22.5472324623564,
15.));
#33354=CARTESIAN_POINT('Ctrl Pts',(-5.44510186987254,-22.4894020366778,
15.));
#33355=CARTESIAN_POINT('Ctrl Pts',(-5.37793718711213,-22.4312416086453,
15.));
#33356=CARTESIAN_POINT('Ctrl Pts',(-5.31129163978934,-22.3727524152125,
15.));
#33357=CARTESIAN_POINT('Ctrl Pts',(-5.24516957209273,-22.3139356039553,
15.));
#33358=CARTESIAN_POINT('Ctrl Pts',(-5.17957547700993,-22.2547923093751,
15.));
#33359=CARTESIAN_POINT('Ctrl Pts',(-5.11451415224484,-22.1953237422816,
15.));
#33360=CARTESIAN_POINT('Ctrl Pts',(-5.04999072201681,-22.1355312202693,
15.));
#33361=CARTESIAN_POINT('Ctrl Pts',(-4.98601051193087,-22.0754161299398,
15.));
#33362=CARTESIAN_POINT('Ctrl Pts',(-4.92257895332779,-22.0149799098431,
15.));
#33363=CARTESIAN_POINT('Ctrl Pts',(-4.85970148585196,-21.9542240269191,
15.));
#33364=CARTESIAN_POINT('Ctrl Pts',(-4.7973834230091,-21.8931499593332,15.));
#33365=CARTESIAN_POINT('Ctrl Pts',(-4.73562994468575,-21.8317591750867,
15.));
#33366=CARTESIAN_POINT('Ctrl Pts',(-4.67444631371023,-21.770053106418,15.));
#33367=CARTESIAN_POINT('Ctrl Pts',(-4.6138380475249,-21.7080331252945,15.));
#33368=CARTESIAN_POINT('Ctrl Pts',(-4.55381108432127,-21.6457005243617,
15.));
#33369=CARTESIAN_POINT('Ctrl Pts',(-4.49437199472475,-21.5830564890896,
15.));
#33370=CARTESIAN_POINT('Ctrl Pts',(-4.4355280204703,-21.5201021036274,15.));
#33371=CARTESIAN_POINT('Ctrl Pts',(-4.37728667813637,-21.4568384368826,
15.));
#33372=CARTESIAN_POINT('Ctrl Pts',(-4.31965542378783,-21.3932666198096,
15.));
#33373=CARTESIAN_POINT('Ctrl Pts',(-4.26264132842712,-21.3293879189372,
15.));
#33374=CARTESIAN_POINT('Ctrl Pts',(-4.20625065101369,-21.2652038365365,
15.));
#33375=CARTESIAN_POINT('Ctrl Pts',(-4.15048873695646,-21.2007161321625,
15.));
#33376=CARTESIAN_POINT('Ctrl Pts',(-4.09536099504429,-21.1359265833073,
15.));
#33377=CARTESIAN_POINT('Ctrl Pts',(-4.04087373166023,-21.0708367812416,
15.));
#33378=CARTESIAN_POINT('Ctrl Pts',(-3.98703495407281,-21.0054479357374,
15.));
#33379=CARTESIAN_POINT('Ctrl Pts',(-3.93385538070582,-20.9397606289993,
15.));
#33380=CARTESIAN_POINT('Ctrl Pts',(-3.88134876172354,-20.8737747416623,
15.));
#33381=CARTESIAN_POINT('Ctrl Pts',(-3.82952970701916,-20.8074899980321,
15.));
#33382=CARTESIAN_POINT('Ctrl Pts',(-3.77841179839888,-20.740906441832,15.));
#33383=CARTESIAN_POINT('Ctrl Pts',(-3.7280057984962,-20.6740248879992,15.));
#33384=CARTESIAN_POINT('Ctrl Pts',(-3.67831730617888,-20.6068475141781,
15.));
#33385=CARTESIAN_POINT('Ctrl Pts',(-3.6293461872059,-20.5393780076057,15.));
#33386=CARTESIAN_POINT('Ctrl Pts',(-3.58109188218494,-20.4716202388531,
15.));
#33387=CARTESIAN_POINT('Ctrl Pts',(-3.53355803178955,-20.4035771072894,
15.));
#33388=CARTESIAN_POINT('Ctrl Pts',(-3.48675677306967,-20.3352494700167,
15.));
#33389=CARTESIAN_POINT('Ctrl Pts',(-3.44071459161672,-20.2666346804507,
15.));
#33390=CARTESIAN_POINT('Ctrl Pts',(-3.39547305068768,-20.1977264147619,
15.));
#33391=CARTESIAN_POINT('Ctrl Pts',(-3.35107647578201,-20.1285177769596,
15.));
#33392=CARTESIAN_POINT('Ctrl Pts',(-3.30756123886962,-20.0590040020604,
15.));
#33393=CARTESIAN_POINT('Ctrl Pts',(-3.26494616363974,-19.9891848794807,
15.));
#33394=CARTESIAN_POINT('Ctrl Pts',(-3.22321820350857,-19.9190683616661,
15.));
#33395=CARTESIAN_POINT('Ctrl Pts',(-3.18233430962982,-19.8486701154397,
15.));
#33396=CARTESIAN_POINT('Ctrl Pts',(-3.14225139572431,-19.7780060327855,
15.));
#33397=CARTESIAN_POINT('Ctrl Pts',(-3.10295238390997,-19.7070857227052,
15.));
#33398=CARTESIAN_POINT('Ctrl Pts',(-3.06446889170638,-19.635906849522,15.));
#33399=CARTESIAN_POINT('Ctrl Pts',(-3.02691741043284,-19.5644460803884,
15.));
#33400=CARTESIAN_POINT('Ctrl Pts',(-2.99048468792079,-19.4926628032527,
15.));
#33401=CARTESIAN_POINT('Ctrl Pts',(-2.95535900926266,-19.420516469599,15.));
#33402=CARTESIAN_POINT('Ctrl Pts',(-2.92166984506916,-19.3479817954251,
15.));
#33403=CARTESIAN_POINT('Ctrl Pts',(-2.88943670541709,-19.2750617358775,
15.));
#33404=CARTESIAN_POINT('Ctrl Pts',(-2.85848240467742,-19.2018091932025,
15.));
#33405=CARTESIAN_POINT('Ctrl Pts',(-2.828507852372,-19.1283090202125,15.));
#33406=CARTESIAN_POINT('Ctrl Pts',(-2.79926206958176,-19.0546365637297,
15.));
#33407=CARTESIAN_POINT('Ctrl Pts',(-2.77069196504715,-18.980821277801,15.));
#33408=CARTESIAN_POINT('Ctrl Pts',(-2.74308150095405,-18.9068127424043,
15.));
#33409=CARTESIAN_POINT('Ctrl Pts',(-2.71724545050995,-18.8324337861517,
15.));
#33410=CARTESIAN_POINT('Ctrl Pts',(-2.69432739305028,-18.7574274222161,
15.));
#33411=CARTESIAN_POINT('Ctrl Pts',(-2.67926286296662,-18.696707670787,15.));
#33412=CARTESIAN_POINT('Ctrl Pts',(-2.67022099202409,-18.6506703537007,
15.));
#33413=CARTESIAN_POINT('Ctrl Pts',(-2.66524945599055,-18.6197453967525,
15.));
#33414=CARTESIAN_POINT('Ctrl Pts',(-2.6630277880543,-18.6042245638953,15.));
#33415=CARTESIAN_POINT('',(-6.29006564240232,-23.1610680715348,0.));
#33416=CARTESIAN_POINT('Origin',(-3.5746082146807E-14,-1.09790581218125E-13,
0.));
#33417=CARTESIAN_POINT('',(-8.52496423935285,-22.4349054983023,0.));
#33418=CARTESIAN_POINT('Origin',(-3.5746082146807E-14,-1.09790581218125E-13,
0.));
#33419=CARTESIAN_POINT('',(-8.52496423935285,-22.4349054983023,15.));
#33420=CARTESIAN_POINT('Origin',(-3.5746082146807E-14,-1.09790581218125E-13,
15.));
#33421=CARTESIAN_POINT('',(-8.52496423935285,-22.4349054983023,0.));
#33422=CARTESIAN_POINT('Ctrl Pts',(-8.7808540919664,-16.6164222996225,0.));
#33423=CARTESIAN_POINT('Ctrl Pts',(-8.7808540919664,-16.6164222996225,18.));
#33424=CARTESIAN_POINT('Ctrl Pts',(-8.78817964150686,-16.6302847808193,
0.));
#33425=CARTESIAN_POINT('Ctrl Pts',(-8.78817964150686,-16.6302847808193,
18.));
#33426=CARTESIAN_POINT('Ctrl Pts',(-8.80233481798951,-16.6582257921024,
0.));
#33427=CARTESIAN_POINT('Ctrl Pts',(-8.80233481798951,-16.6582257921024,
18.));
#33428=CARTESIAN_POINT('Ctrl Pts',(-8.82207984677447,-16.7007854423938,
0.));
#33429=CARTESIAN_POINT('Ctrl Pts',(-8.82207984677447,-16.7007854423938,
18.));
#33430=CARTESIAN_POINT('Ctrl Pts',(-8.84558256033742,-16.7587634618101,
0.));
#33431=CARTESIAN_POINT('Ctrl Pts',(-8.84558256033742,-16.7587634618101,
18.));
#33432=CARTESIAN_POINT('Ctrl Pts',(-8.87112909692392,-16.8329157811062,
0.));
#33433=CARTESIAN_POINT('Ctrl Pts',(-8.87112909692392,-16.8329157811062,
18.));
#33434=CARTESIAN_POINT('Ctrl Pts',(-8.89394614661329,-16.908275670167,0.));
#33435=CARTESIAN_POINT('Ctrl Pts',(-8.89394614661329,-16.908275670167,18.));
#33436=CARTESIAN_POINT('Ctrl Pts',(-8.91510993758933,-16.9843788566346,
0.));
#33437=CARTESIAN_POINT('Ctrl Pts',(-8.91510993758933,-16.9843788566346,
18.));
#33438=CARTESIAN_POINT('Ctrl Pts',(-8.93538377395244,-17.0608897634975,
0.));
#33439=CARTESIAN_POINT('Ctrl Pts',(-8.93538377395244,-17.0608897634975,
18.));
#33440=CARTESIAN_POINT('Ctrl Pts',(-8.95502702208204,-17.1376822726252,
0.));
#33441=CARTESIAN_POINT('Ctrl Pts',(-8.95502702208204,-17.1376822726252,
18.));
#33442=CARTESIAN_POINT('Ctrl Pts',(-8.97397941759265,-17.2147637614528,
0.));
#33443=CARTESIAN_POINT('Ctrl Pts',(-8.97397941759265,-17.2147637614528,
18.));
#33444=CARTESIAN_POINT('Ctrl Pts',(-8.99199362652257,-17.2922207948279,
0.));
#33445=CARTESIAN_POINT('Ctrl Pts',(-8.99199362652257,-17.2922207948279,
18.));
#33446=CARTESIAN_POINT('Ctrl Pts',(-9.00877780436037,-17.3701605263553,
0.));
#33447=CARTESIAN_POINT('Ctrl Pts',(-9.00877780436037,-17.3701605263553,
18.));
#33448=CARTESIAN_POINT('Ctrl Pts',(-9.0241575097608,-17.4486443043185,0.));
#33449=CARTESIAN_POINT('Ctrl Pts',(-9.0241575097608,-17.4486443043185,18.));
#33450=CARTESIAN_POINT('Ctrl Pts',(-9.03814678971601,-17.5276582702181,
0.));
#33451=CARTESIAN_POINT('Ctrl Pts',(-9.03814678971601,-17.5276582702181,
18.));
#33452=CARTESIAN_POINT('Ctrl Pts',(-9.05086524971401,-17.6071467783263,
0.));
#33453=CARTESIAN_POINT('Ctrl Pts',(-9.05086524971401,-17.6071467783263,
18.));
#33454=CARTESIAN_POINT('Ctrl Pts',(-9.06248904941395,-17.6870319618808,
0.));
#33455=CARTESIAN_POINT('Ctrl Pts',(-9.06248904941395,-17.6870319618808,
18.));
#33456=CARTESIAN_POINT('Ctrl Pts',(-9.07319314215027,-17.7672369091005,
0.));
#33457=CARTESIAN_POINT('Ctrl Pts',(-9.07319314215027,-17.7672369091005,
18.));
#33458=CARTESIAN_POINT('Ctrl Pts',(-9.08308548608349,-17.8477120247758,
0.));
#33459=CARTESIAN_POINT('Ctrl Pts',(-9.08308548608349,-17.8477120247758,
18.));
#33460=CARTESIAN_POINT('Ctrl Pts',(-9.09219303320079,-17.9284406141976,
0.));
#33461=CARTESIAN_POINT('Ctrl Pts',(-9.09219303320079,-17.9284406141976,
18.));
#33462=CARTESIAN_POINT('Ctrl Pts',(-9.10049631917583,-18.0094249416472,
0.));
#33463=CARTESIAN_POINT('Ctrl Pts',(-9.10049631917583,-18.0094249416472,
18.));
#33464=CARTESIAN_POINT('Ctrl Pts',(-9.10795114540259,-18.0906774757189,
0.));
#33465=CARTESIAN_POINT('Ctrl Pts',(-9.10795114540259,-18.0906774757189,
18.));
#33466=CARTESIAN_POINT('Ctrl Pts',(-9.1145134759054,-18.1722108451637,0.));
#33467=CARTESIAN_POINT('Ctrl Pts',(-9.1145134759054,-18.1722108451637,18.));
#33468=CARTESIAN_POINT('Ctrl Pts',(-9.12016808144599,-18.2540262849075,
0.));
#33469=CARTESIAN_POINT('Ctrl Pts',(-9.12016808144599,-18.2540262849075,
18.));
#33470=CARTESIAN_POINT('Ctrl Pts',(-9.12493031448672,-18.3361129010289,
0.));
#33471=CARTESIAN_POINT('Ctrl Pts',(-9.12493031448672,-18.3361129010289,
18.));
#33472=CARTESIAN_POINT('Ctrl Pts',(-9.12883240135631,-18.4184531695731,
0.));
#33473=CARTESIAN_POINT('Ctrl Pts',(-9.12883240135631,-18.4184531695731,
18.));
#33474=CARTESIAN_POINT('Ctrl Pts',(-9.13191425549883,-18.5010266156389,
0.));
#33475=CARTESIAN_POINT('Ctrl Pts',(-9.13191425549883,-18.5010266156389,
18.));
#33476=CARTESIAN_POINT('Ctrl Pts',(-9.13421321934922,-18.5838139250423,
0.));
#33477=CARTESIAN_POINT('Ctrl Pts',(-9.13421321934922,-18.5838139250423,
18.));
#33478=CARTESIAN_POINT('Ctrl Pts',(-9.13575227582419,-18.6668016710749,
0.));
#33479=CARTESIAN_POINT('Ctrl Pts',(-9.13575227582419,-18.6668016710749,
18.));
#33480=CARTESIAN_POINT('Ctrl Pts',(-9.13654074021147,-18.7499820263476,
0.));
#33481=CARTESIAN_POINT('Ctrl Pts',(-9.13654074021147,-18.7499820263476,
18.));
#33482=CARTESIAN_POINT('Ctrl Pts',(-9.13657985367154,-18.8333505052874,
0.));
#33483=CARTESIAN_POINT('Ctrl Pts',(-9.13657985367154,-18.8333505052874,
18.));
#33484=CARTESIAN_POINT('Ctrl Pts',(-9.13586688858169,-18.9169043053388,
0.));
#33485=CARTESIAN_POINT('Ctrl Pts',(-9.13586688858169,-18.9169043053388,
18.));
#33486=CARTESIAN_POINT('Ctrl Pts',(-9.13439956903533,-19.0006405223697,
0.));
#33487=CARTESIAN_POINT('Ctrl Pts',(-9.13439956903533,-19.0006405223697,
18.));
#33488=CARTESIAN_POINT('Ctrl Pts',(-9.13218114462419,-19.0845541036965,
0.));
#33489=CARTESIAN_POINT('Ctrl Pts',(-9.13218114462419,-19.0845541036965,
18.));
#33490=CARTESIAN_POINT('Ctrl Pts',(-9.12921984349375,-19.1686380639041,
0.));
#33491=CARTESIAN_POINT('Ctrl Pts',(-9.12921984349375,-19.1686380639041,
18.));
#33492=CARTESIAN_POINT('Ctrl Pts',(-9.125526627856,-19.2528843844341,0.));
#33493=CARTESIAN_POINT('Ctrl Pts',(-9.125526627856,-19.2528843844341,18.));
#33494=CARTESIAN_POINT('Ctrl Pts',(-9.121113479412,-19.3372847008483,0.));
#33495=CARTESIAN_POINT('Ctrl Pts',(-9.121113479412,-19.3372847008483,18.));
#33496=CARTESIAN_POINT('Ctrl Pts',(-9.1159915924392,-19.4218310275711,0.));
#33497=CARTESIAN_POINT('Ctrl Pts',(-9.1159915924392,-19.4218310275711,18.));
#33498=CARTESIAN_POINT('Ctrl Pts',(-9.11016929611336,-19.5065165934577,
0.));
#33499=CARTESIAN_POINT('Ctrl Pts',(-9.11016929611336,-19.5065165934577,
18.));
#33500=CARTESIAN_POINT('Ctrl Pts',(-9.10365235736465,-19.5913357132276,
0.));
#33501=CARTESIAN_POINT('Ctrl Pts',(-9.10365235736465,-19.5913357132276,
18.));
#33502=CARTESIAN_POINT('Ctrl Pts',(-9.0964449428387,-19.6762833927168,0.));
#33503=CARTESIAN_POINT('Ctrl Pts',(-9.0964449428387,-19.6762833927168,18.));
#33504=CARTESIAN_POINT('Ctrl Pts',(-9.08855038355402,-19.7613550146978,
0.));
#33505=CARTESIAN_POINT('Ctrl Pts',(-9.08855038355402,-19.7613550146978,
18.));
#33506=CARTESIAN_POINT('Ctrl Pts',(-9.07997196979668,-19.846546013708,0.));
#33507=CARTESIAN_POINT('Ctrl Pts',(-9.07997196979668,-19.846546013708,18.));
#33508=CARTESIAN_POINT('Ctrl Pts',(-9.0707138821585,-19.9318514954605,0.));
#33509=CARTESIAN_POINT('Ctrl Pts',(-9.0707138821585,-19.9318514954605,18.));
#33510=CARTESIAN_POINT('Ctrl Pts',(-9.0607810967537,-20.0172662790811,0.));
#33511=CARTESIAN_POINT('Ctrl Pts',(-9.0607810967537,-20.0172662790811,18.));
#33512=CARTESIAN_POINT('Ctrl Pts',(-9.05017898090711,-20.1027850670435,
0.));
#33513=CARTESIAN_POINT('Ctrl Pts',(-9.05017898090711,-20.1027850670435,
18.));
#33514=CARTESIAN_POINT('Ctrl Pts',(-9.03891298737032,-20.1884025764493,
0.));
#33515=CARTESIAN_POINT('Ctrl Pts',(-9.03891298737032,-20.1884025764493,
18.));
#33516=CARTESIAN_POINT('Ctrl Pts',(-9.02698833758324,-20.2741136736186,
0.));
#33517=CARTESIAN_POINT('Ctrl Pts',(-9.02698833758324,-20.2741136736186,
18.));
#33518=CARTESIAN_POINT('Ctrl Pts',(-9.01440965049155,-20.3599135373691,
0.));
#33519=CARTESIAN_POINT('Ctrl Pts',(-9.01440965049155,-20.3599135373691,
18.));
#33520=CARTESIAN_POINT('Ctrl Pts',(-9.00118097039517,-20.4457976315472,
0.));
#33521=CARTESIAN_POINT('Ctrl Pts',(-9.00118097039517,-20.4457976315472,
18.));
#33522=CARTESIAN_POINT('Ctrl Pts',(-8.98730595457659,-20.5317616031369,
0.));
#33523=CARTESIAN_POINT('Ctrl Pts',(-8.98730595457659,-20.5317616031369,
18.));
#33524=CARTESIAN_POINT('Ctrl Pts',(-8.97278801890468,-20.6178012000199,
0.));
#33525=CARTESIAN_POINT('Ctrl Pts',(-8.97278801890468,-20.6178012000199,
18.));
#33526=CARTESIAN_POINT('Ctrl Pts',(-8.95763049112623,-20.7039121898975,
0.));
#33527=CARTESIAN_POINT('Ctrl Pts',(-8.95763049112623,-20.7039121898975,
18.));
#33528=CARTESIAN_POINT('Ctrl Pts',(-8.94183680111377,-20.7900902537083,
0.));
#33529=CARTESIAN_POINT('Ctrl Pts',(-8.94183680111377,-20.7900902537083,
18.));
#33530=CARTESIAN_POINT('Ctrl Pts',(-8.92541048738649,-20.8763310073304,
0.));
#33531=CARTESIAN_POINT('Ctrl Pts',(-8.92541048738649,-20.8763310073304,
18.));
#33532=CARTESIAN_POINT('Ctrl Pts',(-8.90835509843285,-20.9626300944902,
0.));
#33533=CARTESIAN_POINT('Ctrl Pts',(-8.90835509843285,-20.9626300944902,
18.));
#33534=CARTESIAN_POINT('Ctrl Pts',(-8.89067412773386,-21.0489832630915,
0.));
#33535=CARTESIAN_POINT('Ctrl Pts',(-8.89067412773386,-21.0489832630915,
18.));
#33536=CARTESIAN_POINT('Ctrl Pts',(-8.87237094640749,-21.1353864352374,
0.));
#33537=CARTESIAN_POINT('Ctrl Pts',(-8.87237094640749,-21.1353864352374,
18.));
#33538=CARTESIAN_POINT('Ctrl Pts',(-8.85344872418156,-21.2218358113425,
0.));
#33539=CARTESIAN_POINT('Ctrl Pts',(-8.85344872418156,-21.2218358113425,
18.));
#33540=CARTESIAN_POINT('Ctrl Pts',(-8.83391042911629,-21.3083278326642,
0.));
#33541=CARTESIAN_POINT('Ctrl Pts',(-8.83391042911629,-21.3083278326642,
18.));
#33542=CARTESIAN_POINT('Ctrl Pts',(-8.81375890120582,-21.3948590173441,
0.));
#33543=CARTESIAN_POINT('Ctrl Pts',(-8.81375890120582,-21.3948590173441,
18.));
#33544=CARTESIAN_POINT('Ctrl Pts',(-8.79299691277858,-21.481425822209,0.));
#33545=CARTESIAN_POINT('Ctrl Pts',(-8.79299691277858,-21.481425822209,18.));
#33546=CARTESIAN_POINT('Ctrl Pts',(-8.77162723103299,-21.5680245138584,
0.));
#33547=CARTESIAN_POINT('Ctrl Pts',(-8.77162723103299,-21.5680245138584,
18.));
#33548=CARTESIAN_POINT('Ctrl Pts',(-8.74965270266163,-21.6546509866725,
0.));
#33549=CARTESIAN_POINT('Ctrl Pts',(-8.74965270266163,-21.6546509866725,
18.));
#33550=CARTESIAN_POINT('Ctrl Pts',(-8.72707626956922,-21.7413007707864,
0.));
#33551=CARTESIAN_POINT('Ctrl Pts',(-8.72707626956922,-21.7413007707864,
18.));
#33552=CARTESIAN_POINT('Ctrl Pts',(-8.70390086252203,-21.8279693631274,
0.));
#33553=CARTESIAN_POINT('Ctrl Pts',(-8.70390086252203,-21.8279693631274,
18.));
#33554=CARTESIAN_POINT('Ctrl Pts',(-8.68012932645739,-21.9146524902336,
0.));
#33555=CARTESIAN_POINT('Ctrl Pts',(-8.68012932645739,-21.9146524902336,
18.));
#33556=CARTESIAN_POINT('Ctrl Pts',(-8.6557643376698,-22.0013463859623,0.));
#33557=CARTESIAN_POINT('Ctrl Pts',(-8.6557643376698,-22.0013463859623,18.));
#33558=CARTESIAN_POINT('Ctrl Pts',(-8.63080832792612,-22.0880480931906,
0.));
#33559=CARTESIAN_POINT('Ctrl Pts',(-8.63080832792612,-22.0880480931906,
18.));
#33560=CARTESIAN_POINT('Ctrl Pts',(-8.60526341207614,-22.1747556651024,
0.));
#33561=CARTESIAN_POINT('Ctrl Pts',(-8.60526341207614,-22.1747556651024,
18.));
#33562=CARTESIAN_POINT('Ctrl Pts',(-8.57913133085326,-22.2614679221213,
0.));
#33563=CARTESIAN_POINT('Ctrl Pts',(-8.57913133085326,-22.2614679221213,
18.));
#33564=CARTESIAN_POINT('Ctrl Pts',(-8.55775698160722,-22.3308410047044,
0.));
#33565=CARTESIAN_POINT('Ctrl Pts',(-8.55775698160722,-22.3308410047044,
18.));
#33566=CARTESIAN_POINT('Ctrl Pts',(-8.54146295656907,-22.3828725698612,
0.));
#33567=CARTESIAN_POINT('Ctrl Pts',(-8.54146295656907,-22.3828725698612,
18.));
#33568=CARTESIAN_POINT('Ctrl Pts',(-8.53048330625155,-22.4175610589877,
0.));
#33569=CARTESIAN_POINT('Ctrl Pts',(-8.53048330625155,-22.4175610589877,
18.));
#33570=CARTESIAN_POINT('Ctrl Pts',(-8.52496423935285,-22.4349054983023,
0.));
#33571=CARTESIAN_POINT('Ctrl Pts',(-8.52496423935285,-22.4349054983023,
18.));
#33572=CARTESIAN_POINT('Ctrl Pts',(-8.7808540919664,-16.6164222996225,0.));
#33573=CARTESIAN_POINT('Ctrl Pts',(-8.78817964150686,-16.6302847808193,
0.));
#33574=CARTESIAN_POINT('Ctrl Pts',(-8.80233481798951,-16.6582257921024,
0.));
#33575=CARTESIAN_POINT('Ctrl Pts',(-8.82207984677447,-16.7007854423938,
0.));
#33576=CARTESIAN_POINT('Ctrl Pts',(-8.84558256033742,-16.7587634618101,
0.));
#33577=CARTESIAN_POINT('Ctrl Pts',(-8.87112909692392,-16.8329157811062,
0.));
#33578=CARTESIAN_POINT('Ctrl Pts',(-8.89394614661329,-16.908275670167,0.));
#33579=CARTESIAN_POINT('Ctrl Pts',(-8.91510993758933,-16.9843788566346,
0.));
#33580=CARTESIAN_POINT('Ctrl Pts',(-8.93538377395244,-17.0608897634975,
0.));
#33581=CARTESIAN_POINT('Ctrl Pts',(-8.95502702208204,-17.1376822726252,
0.));
#33582=CARTESIAN_POINT('Ctrl Pts',(-8.97397941759265,-17.2147637614528,
0.));
#33583=CARTESIAN_POINT('Ctrl Pts',(-8.99199362652257,-17.2922207948279,
0.));
#33584=CARTESIAN_POINT('Ctrl Pts',(-9.00877780436037,-17.3701605263553,
0.));
#33585=CARTESIAN_POINT('Ctrl Pts',(-9.0241575097608,-17.4486443043185,0.));
#33586=CARTESIAN_POINT('Ctrl Pts',(-9.03814678971601,-17.5276582702181,
0.));
#33587=CARTESIAN_POINT('Ctrl Pts',(-9.05086524971401,-17.6071467783263,
0.));
#33588=CARTESIAN_POINT('Ctrl Pts',(-9.06248904941395,-17.6870319618808,
0.));
#33589=CARTESIAN_POINT('Ctrl Pts',(-9.07319314215027,-17.7672369091005,
0.));
#33590=CARTESIAN_POINT('Ctrl Pts',(-9.08308548608349,-17.8477120247758,
0.));
#33591=CARTESIAN_POINT('Ctrl Pts',(-9.09219303320079,-17.9284406141976,
0.));
#33592=CARTESIAN_POINT('Ctrl Pts',(-9.10049631917583,-18.0094249416472,
0.));
#33593=CARTESIAN_POINT('Ctrl Pts',(-9.10795114540259,-18.0906774757189,
0.));
#33594=CARTESIAN_POINT('Ctrl Pts',(-9.1145134759054,-18.1722108451637,0.));
#33595=CARTESIAN_POINT('Ctrl Pts',(-9.12016808144599,-18.2540262849075,
0.));
#33596=CARTESIAN_POINT('Ctrl Pts',(-9.12493031448672,-18.3361129010289,
0.));
#33597=CARTESIAN_POINT('Ctrl Pts',(-9.12883240135631,-18.4184531695731,
0.));
#33598=CARTESIAN_POINT('Ctrl Pts',(-9.13191425549883,-18.5010266156389,
0.));
#33599=CARTESIAN_POINT('Ctrl Pts',(-9.13421321934922,-18.5838139250423,
0.));
#33600=CARTESIAN_POINT('Ctrl Pts',(-9.13575227582419,-18.6668016710749,
0.));
#33601=CARTESIAN_POINT('Ctrl Pts',(-9.13654074021147,-18.7499820263476,
0.));
#33602=CARTESIAN_POINT('Ctrl Pts',(-9.13657985367154,-18.8333505052874,
0.));
#33603=CARTESIAN_POINT('Ctrl Pts',(-9.13586688858169,-18.9169043053388,
0.));
#33604=CARTESIAN_POINT('Ctrl Pts',(-9.13439956903533,-19.0006405223697,
0.));
#33605=CARTESIAN_POINT('Ctrl Pts',(-9.13218114462419,-19.0845541036965,
0.));
#33606=CARTESIAN_POINT('Ctrl Pts',(-9.12921984349375,-19.1686380639041,
0.));
#33607=CARTESIAN_POINT('Ctrl Pts',(-9.125526627856,-19.2528843844341,0.));
#33608=CARTESIAN_POINT('Ctrl Pts',(-9.121113479412,-19.3372847008483,0.));
#33609=CARTESIAN_POINT('Ctrl Pts',(-9.1159915924392,-19.4218310275711,0.));
#33610=CARTESIAN_POINT('Ctrl Pts',(-9.11016929611336,-19.5065165934577,
0.));
#33611=CARTESIAN_POINT('Ctrl Pts',(-9.10365235736465,-19.5913357132276,
0.));
#33612=CARTESIAN_POINT('Ctrl Pts',(-9.0964449428387,-19.6762833927168,0.));
#33613=CARTESIAN_POINT('Ctrl Pts',(-9.08855038355402,-19.7613550146978,
0.));
#33614=CARTESIAN_POINT('Ctrl Pts',(-9.07997196979668,-19.846546013708,0.));
#33615=CARTESIAN_POINT('Ctrl Pts',(-9.0707138821585,-19.9318514954605,0.));
#33616=CARTESIAN_POINT('Ctrl Pts',(-9.0607810967537,-20.0172662790811,0.));
#33617=CARTESIAN_POINT('Ctrl Pts',(-9.05017898090711,-20.1027850670435,
0.));
#33618=CARTESIAN_POINT('Ctrl Pts',(-9.03891298737032,-20.1884025764493,
0.));
#33619=CARTESIAN_POINT('Ctrl Pts',(-9.02698833758324,-20.2741136736186,
0.));
#33620=CARTESIAN_POINT('Ctrl Pts',(-9.01440965049155,-20.3599135373691,
0.));
#33621=CARTESIAN_POINT('Ctrl Pts',(-9.00118097039517,-20.4457976315472,
0.));
#33622=CARTESIAN_POINT('Ctrl Pts',(-8.98730595457659,-20.5317616031369,
0.));
#33623=CARTESIAN_POINT('Ctrl Pts',(-8.97278801890468,-20.6178012000199,
0.));
#33624=CARTESIAN_POINT('Ctrl Pts',(-8.95763049112623,-20.7039121898975,
0.));
#33625=CARTESIAN_POINT('Ctrl Pts',(-8.94183680111377,-20.7900902537083,
0.));
#33626=CARTESIAN_POINT('Ctrl Pts',(-8.92541048738649,-20.8763310073304,
0.));
#33627=CARTESIAN_POINT('Ctrl Pts',(-8.90835509843285,-20.9626300944902,
0.));
#33628=CARTESIAN_POINT('Ctrl Pts',(-8.89067412773386,-21.0489832630915,
0.));
#33629=CARTESIAN_POINT('Ctrl Pts',(-8.87237094640749,-21.1353864352374,
0.));
#33630=CARTESIAN_POINT('Ctrl Pts',(-8.85344872418156,-21.2218358113425,
0.));
#33631=CARTESIAN_POINT('Ctrl Pts',(-8.83391042911629,-21.3083278326642,
0.));
#33632=CARTESIAN_POINT('Ctrl Pts',(-8.81375890120582,-21.3948590173441,
0.));
#33633=CARTESIAN_POINT('Ctrl Pts',(-8.79299691277858,-21.481425822209,0.));
#33634=CARTESIAN_POINT('Ctrl Pts',(-8.77162723103299,-21.5680245138584,
0.));
#33635=CARTESIAN_POINT('Ctrl Pts',(-8.74965270266163,-21.6546509866725,
0.));
#33636=CARTESIAN_POINT('Ctrl Pts',(-8.72707626956922,-21.7413007707864,
0.));
#33637=CARTESIAN_POINT('Ctrl Pts',(-8.70390086252203,-21.8279693631274,
0.));
#33638=CARTESIAN_POINT('Ctrl Pts',(-8.68012932645739,-21.9146524902336,
0.));
#33639=CARTESIAN_POINT('Ctrl Pts',(-8.6557643376698,-22.0013463859623,0.));
#33640=CARTESIAN_POINT('Ctrl Pts',(-8.63080832792612,-22.0880480931906,
0.));
#33641=CARTESIAN_POINT('Ctrl Pts',(-8.60015442890614,-22.1920971794848,
0.));
#33642=CARTESIAN_POINT('Ctrl Pts',(-8.57387555634004,-22.2788106077804,
0.));
#33643=CARTESIAN_POINT('Ctrl Pts',(-8.55238412336295,-22.3481844703457,
0.));
#33644=CARTESIAN_POINT('Ctrl Pts',(-8.53600237317213,-22.4002166196189,
0.));
#33645=CARTESIAN_POINT('Ctrl Pts',(-8.52496423935285,-22.4349054983023,
0.));
#33646=CARTESIAN_POINT('Ctrl Pts',(-8.7808540919664,-16.6164222996225,15.));
#33647=CARTESIAN_POINT('Ctrl Pts',(-8.78817964150686,-16.6302847808193,
15.));
#33648=CARTESIAN_POINT('Ctrl Pts',(-8.80233481798951,-16.6582257921024,
15.));
#33649=CARTESIAN_POINT('Ctrl Pts',(-8.82207984677447,-16.7007854423938,
15.));
#33650=CARTESIAN_POINT('Ctrl Pts',(-8.84558256033742,-16.7587634618101,
15.));
#33651=CARTESIAN_POINT('Ctrl Pts',(-8.87112909692392,-16.8329157811062,
15.));
#33652=CARTESIAN_POINT('Ctrl Pts',(-8.89394614661329,-16.908275670167,15.));
#33653=CARTESIAN_POINT('Ctrl Pts',(-8.91510993758933,-16.9843788566346,
15.));
#33654=CARTESIAN_POINT('Ctrl Pts',(-8.93538377395244,-17.0608897634975,
15.));
#33655=CARTESIAN_POINT('Ctrl Pts',(-8.95502702208204,-17.1376822726252,
15.));
#33656=CARTESIAN_POINT('Ctrl Pts',(-8.97397941759265,-17.2147637614528,
15.));
#33657=CARTESIAN_POINT('Ctrl Pts',(-8.99199362652257,-17.2922207948279,
15.));
#33658=CARTESIAN_POINT('Ctrl Pts',(-9.00877780436037,-17.3701605263553,
15.));
#33659=CARTESIAN_POINT('Ctrl Pts',(-9.0241575097608,-17.4486443043185,15.));
#33660=CARTESIAN_POINT('Ctrl Pts',(-9.03814678971601,-17.5276582702181,
15.));
#33661=CARTESIAN_POINT('Ctrl Pts',(-9.05086524971401,-17.6071467783263,
15.));
#33662=CARTESIAN_POINT('Ctrl Pts',(-9.06248904941395,-17.6870319618808,
15.));
#33663=CARTESIAN_POINT('Ctrl Pts',(-9.07319314215027,-17.7672369091005,
15.));
#33664=CARTESIAN_POINT('Ctrl Pts',(-9.08308548608349,-17.8477120247758,
15.));
#33665=CARTESIAN_POINT('Ctrl Pts',(-9.09219303320079,-17.9284406141976,
15.));
#33666=CARTESIAN_POINT('Ctrl Pts',(-9.10049631917583,-18.0094249416472,
15.));
#33667=CARTESIAN_POINT('Ctrl Pts',(-9.10795114540259,-18.0906774757189,
15.));
#33668=CARTESIAN_POINT('Ctrl Pts',(-9.1145134759054,-18.1722108451637,15.));
#33669=CARTESIAN_POINT('Ctrl Pts',(-9.12016808144599,-18.2540262849075,
15.));
#33670=CARTESIAN_POINT('Ctrl Pts',(-9.12493031448672,-18.3361129010289,
15.));
#33671=CARTESIAN_POINT('Ctrl Pts',(-9.12883240135631,-18.4184531695731,
15.));
#33672=CARTESIAN_POINT('Ctrl Pts',(-9.13191425549883,-18.5010266156389,
15.));
#33673=CARTESIAN_POINT('Ctrl Pts',(-9.13421321934922,-18.5838139250423,
15.));
#33674=CARTESIAN_POINT('Ctrl Pts',(-9.13575227582419,-18.6668016710749,
15.));
#33675=CARTESIAN_POINT('Ctrl Pts',(-9.13654074021147,-18.7499820263476,
15.));
#33676=CARTESIAN_POINT('Ctrl Pts',(-9.13657985367154,-18.8333505052874,
15.));
#33677=CARTESIAN_POINT('Ctrl Pts',(-9.13586688858169,-18.9169043053388,
15.));
#33678=CARTESIAN_POINT('Ctrl Pts',(-9.13439956903533,-19.0006405223697,
15.));
#33679=CARTESIAN_POINT('Ctrl Pts',(-9.13218114462419,-19.0845541036965,
15.));
#33680=CARTESIAN_POINT('Ctrl Pts',(-9.12921984349375,-19.1686380639041,
15.));
#33681=CARTESIAN_POINT('Ctrl Pts',(-9.125526627856,-19.2528843844341,15.));
#33682=CARTESIAN_POINT('Ctrl Pts',(-9.121113479412,-19.3372847008483,15.));
#33683=CARTESIAN_POINT('Ctrl Pts',(-9.1159915924392,-19.4218310275711,15.));
#33684=CARTESIAN_POINT('Ctrl Pts',(-9.11016929611336,-19.5065165934577,
15.));
#33685=CARTESIAN_POINT('Ctrl Pts',(-9.10365235736465,-19.5913357132276,
15.));
#33686=CARTESIAN_POINT('Ctrl Pts',(-9.0964449428387,-19.6762833927168,15.));
#33687=CARTESIAN_POINT('Ctrl Pts',(-9.08855038355402,-19.7613550146978,
15.));
#33688=CARTESIAN_POINT('Ctrl Pts',(-9.07997196979668,-19.846546013708,15.));
#33689=CARTESIAN_POINT('Ctrl Pts',(-9.0707138821585,-19.9318514954605,15.));
#33690=CARTESIAN_POINT('Ctrl Pts',(-9.0607810967537,-20.0172662790811,15.));
#33691=CARTESIAN_POINT('Ctrl Pts',(-9.05017898090711,-20.1027850670435,
15.));
#33692=CARTESIAN_POINT('Ctrl Pts',(-9.03891298737032,-20.1884025764493,
15.));
#33693=CARTESIAN_POINT('Ctrl Pts',(-9.02698833758324,-20.2741136736186,
15.));
#33694=CARTESIAN_POINT('Ctrl Pts',(-9.01440965049155,-20.3599135373691,
15.));
#33695=CARTESIAN_POINT('Ctrl Pts',(-9.00118097039517,-20.4457976315472,
15.));
#33696=CARTESIAN_POINT('Ctrl Pts',(-8.98730595457659,-20.5317616031369,
15.));
#33697=CARTESIAN_POINT('Ctrl Pts',(-8.97278801890468,-20.6178012000199,
15.));
#33698=CARTESIAN_POINT('Ctrl Pts',(-8.95763049112623,-20.7039121898975,
15.));
#33699=CARTESIAN_POINT('Ctrl Pts',(-8.94183680111377,-20.7900902537083,
15.));
#33700=CARTESIAN_POINT('Ctrl Pts',(-8.92541048738649,-20.8763310073304,
15.));
#33701=CARTESIAN_POINT('Ctrl Pts',(-8.90835509843285,-20.9626300944902,
15.));
#33702=CARTESIAN_POINT('Ctrl Pts',(-8.89067412773386,-21.0489832630915,
15.));
#33703=CARTESIAN_POINT('Ctrl Pts',(-8.87237094640749,-21.1353864352374,
15.));
#33704=CARTESIAN_POINT('Ctrl Pts',(-8.85344872418156,-21.2218358113425,
15.));
#33705=CARTESIAN_POINT('Ctrl Pts',(-8.83391042911629,-21.3083278326642,
15.));
#33706=CARTESIAN_POINT('Ctrl Pts',(-8.81375890120582,-21.3948590173441,
15.));
#33707=CARTESIAN_POINT('Ctrl Pts',(-8.79299691277858,-21.481425822209,15.));
#33708=CARTESIAN_POINT('Ctrl Pts',(-8.77162723103299,-21.5680245138584,
15.));
#33709=CARTESIAN_POINT('Ctrl Pts',(-8.74965270266163,-21.6546509866725,
15.));
#33710=CARTESIAN_POINT('Ctrl Pts',(-8.72707626956922,-21.7413007707864,
15.));
#33711=CARTESIAN_POINT('Ctrl Pts',(-8.70390086252203,-21.8279693631274,
15.));
#33712=CARTESIAN_POINT('Ctrl Pts',(-8.68012932645739,-21.9146524902336,
15.));
#33713=CARTESIAN_POINT('Ctrl Pts',(-8.6557643376698,-22.0013463859623,15.));
#33714=CARTESIAN_POINT('Ctrl Pts',(-8.63080832792612,-22.0880480931906,
15.));
#33715=CARTESIAN_POINT('Ctrl Pts',(-8.60015442890614,-22.1920971794848,
15.));
#33716=CARTESIAN_POINT('Ctrl Pts',(-8.57387555634004,-22.2788106077804,
15.));
#33717=CARTESIAN_POINT('Ctrl Pts',(-8.55238412336295,-22.3481844703457,
15.));
#33718=CARTESIAN_POINT('Ctrl Pts',(-8.53600237317213,-22.4002166196189,
15.));
#33719=CARTESIAN_POINT('Ctrl Pts',(-8.52496423935285,-22.4349054983023,
15.));
#33720=CARTESIAN_POINT('Ctrl Pts',(-18.7025042402277,-15.040489857191,0.));
#33721=CARTESIAN_POINT('Ctrl Pts',(-18.7025042402277,-15.040489857191,18.));
#33722=CARTESIAN_POINT('Ctrl Pts',(-18.6843032127312,-15.0403790752228,
0.));
#33723=CARTESIAN_POINT('Ctrl Pts',(-18.6843032127312,-15.0403790752228,
18.));
#33724=CARTESIAN_POINT('Ctrl Pts',(-18.6479196005666,-15.0401020105546,
0.));
#33725=CARTESIAN_POINT('Ctrl Pts',(-18.6479196005666,-15.0401020105546,
18.));
#33726=CARTESIAN_POINT('Ctrl Pts',(-18.5933995108277,-15.0395199113665,
0.));
#33727=CARTESIAN_POINT('Ctrl Pts',(-18.5933995108277,-15.0395199113665,
18.));
#33728=CARTESIAN_POINT('Ctrl Pts',(-18.5208167514208,-15.0384106640281,
0.));
#33729=CARTESIAN_POINT('Ctrl Pts',(-18.5208167514208,-15.0384106640281,
18.));
#33730=CARTESIAN_POINT('Ctrl Pts',(-18.4302732371441,-15.0364681891201,
0.));
#33731=CARTESIAN_POINT('Ctrl Pts',(-18.4302732371441,-15.0364681891201,
18.));
#33732=CARTESIAN_POINT('Ctrl Pts',(-18.3399156227477,-15.0339687345357,
0.));
#33733=CARTESIAN_POINT('Ctrl Pts',(-18.3399156227477,-15.0339687345357,
18.));
#33734=CARTESIAN_POINT('Ctrl Pts',(-18.2497455679917,-15.0309110092482,
0.));
#33735=CARTESIAN_POINT('Ctrl Pts',(-18.2497455679917,-15.0309110092482,
18.));
#33736=CARTESIAN_POINT('Ctrl Pts',(-18.1597655779328,-15.0272936035154,
0.));
#33737=CARTESIAN_POINT('Ctrl Pts',(-18.1597655779328,-15.0272936035154,
18.));
#33738=CARTESIAN_POINT('Ctrl Pts',(-18.0699792164192,-15.0231151183906,
0.));
#33739=CARTESIAN_POINT('Ctrl Pts',(-18.0699792164192,-15.0231151183906,
18.));
#33740=CARTESIAN_POINT('Ctrl Pts',(-17.980390892286,-15.0183741723687,0.));
#33741=CARTESIAN_POINT('Ctrl Pts',(-17.980390892286,-15.0183741723687,18.));
#33742=CARTESIAN_POINT('Ctrl Pts',(-17.891005548971,-15.0130693803259,0.));
#33743=CARTESIAN_POINT('Ctrl Pts',(-17.891005548971,-15.0130693803259,18.));
#33744=CARTESIAN_POINT('Ctrl Pts',(-17.8018283748074,-15.0071993464636,
0.));
#33745=CARTESIAN_POINT('Ctrl Pts',(-17.8018283748074,-15.0071993464636,
18.));
#33746=CARTESIAN_POINT('Ctrl Pts',(-17.7128645299878,-15.0007626541286,
0.));
#33747=CARTESIAN_POINT('Ctrl Pts',(-17.7128645299878,-15.0007626541286,
18.));
#33748=CARTESIAN_POINT('Ctrl Pts',(-17.6241187988652,-14.9937578646616,
0.));
#33749=CARTESIAN_POINT('Ctrl Pts',(-17.6241187988652,-14.9937578646616,
18.));
#33750=CARTESIAN_POINT('Ctrl Pts',(-17.5355955872257,-14.9861834999847,
0.));
#33751=CARTESIAN_POINT('Ctrl Pts',(-17.5355955872257,-14.9861834999847,
18.));
#33752=CARTESIAN_POINT('Ctrl Pts',(-17.4472991215239,-14.9780380183576,
0.));
#33753=CARTESIAN_POINT('Ctrl Pts',(-17.4472991215239,-14.9780380183576,
18.));
#33754=CARTESIAN_POINT('Ctrl Pts',(-17.3592335908103,-14.9693197947387,
0.));
#33755=CARTESIAN_POINT('Ctrl Pts',(-17.3592335908103,-14.9693197947387,
18.));
#33756=CARTESIAN_POINT('Ctrl Pts',(-17.2714032968314,-14.9600271060471,
0.));
#33757=CARTESIAN_POINT('Ctrl Pts',(-17.2714032968314,-14.9600271060471,
18.));
#33758=CARTESIAN_POINT('Ctrl Pts',(-17.1838128327073,-14.9501581118289,
0.));
#33759=CARTESIAN_POINT('Ctrl Pts',(-17.1838128327073,-14.9501581118289,
18.));
#33760=CARTESIAN_POINT('Ctrl Pts',(-17.0964671184813,-14.9397108660998,
0.));
#33761=CARTESIAN_POINT('Ctrl Pts',(-17.0964671184813,-14.9397108660998,
18.));
#33762=CARTESIAN_POINT('Ctrl Pts',(-17.0093712776822,-14.9286833603319,
0.));
#33763=CARTESIAN_POINT('Ctrl Pts',(-17.0093712776822,-14.9286833603319,
18.));
#33764=CARTESIAN_POINT('Ctrl Pts',(-16.9225305499155,-14.9170735658747,
0.));
#33765=CARTESIAN_POINT('Ctrl Pts',(-16.9225305499155,-14.9170735658747,
18.));
#33766=CARTESIAN_POINT('Ctrl Pts',(-16.8359501981915,-14.9048794721647,
0.));
#33767=CARTESIAN_POINT('Ctrl Pts',(-16.8359501981915,-14.9048794721647,
18.));
#33768=CARTESIAN_POINT('Ctrl Pts',(-16.7496353900706,-14.8920991518626,
0.));
#33769=CARTESIAN_POINT('Ctrl Pts',(-16.7496353900706,-14.8920991518626,
18.));
#33770=CARTESIAN_POINT('Ctrl Pts',(-16.6635911790385,-14.8787307479454,
0.));
#33771=CARTESIAN_POINT('Ctrl Pts',(-16.6635911790385,-14.8787307479454,
18.));
#33772=CARTESIAN_POINT('Ctrl Pts',(-16.5778226646614,-14.8647723257055,
0.));
#33773=CARTESIAN_POINT('Ctrl Pts',(-16.5778226646614,-14.8647723257055,
18.));
#33774=CARTESIAN_POINT('Ctrl Pts',(-16.492335117066,-14.8502217520165,0.));
#33775=CARTESIAN_POINT('Ctrl Pts',(-16.492335117066,-14.8502217520165,18.));
#33776=CARTESIAN_POINT('Ctrl Pts',(-16.4071341001481,-14.8350765822692,
0.));
#33777=CARTESIAN_POINT('Ctrl Pts',(-16.4071341001481,-14.8350765822692,
18.));
#33778=CARTESIAN_POINT('Ctrl Pts',(-16.3222256264574,-14.8193339134125,
0.));
#33779=CARTESIAN_POINT('Ctrl Pts',(-16.3222256264574,-14.8193339134125,
18.));
#33780=CARTESIAN_POINT('Ctrl Pts',(-16.2376161919272,-14.8029903659562,
0.));
#33781=CARTESIAN_POINT('Ctrl Pts',(-16.2376161919272,-14.8029903659562,
18.));
#33782=CARTESIAN_POINT('Ctrl Pts',(-16.1533125058853,-14.7860423865308,
0.));
#33783=CARTESIAN_POINT('Ctrl Pts',(-16.1533125058853,-14.7860423865308,
18.));
#33784=CARTESIAN_POINT('Ctrl Pts',(-16.0693212651732,-14.7684865075326,
0.));
#33785=CARTESIAN_POINT('Ctrl Pts',(-16.0693212651732,-14.7684865075326,
18.));
#33786=CARTESIAN_POINT('Ctrl Pts',(-15.9856489347991,-14.7503195973741,
0.));
#33787=CARTESIAN_POINT('Ctrl Pts',(-15.9856489347991,-14.7503195973741,
18.));
#33788=CARTESIAN_POINT('Ctrl Pts',(-15.9023014613802,-14.7315391924939,
0.));
#33789=CARTESIAN_POINT('Ctrl Pts',(-15.9023014613802,-14.7315391924939,
18.));
#33790=CARTESIAN_POINT('Ctrl Pts',(-15.8192842036838,-14.7121435744495,
0.));
#33791=CARTESIAN_POINT('Ctrl Pts',(-15.8192842036838,-14.7121435744495,
18.));
#33792=CARTESIAN_POINT('Ctrl Pts',(-15.7366025822956,-14.692131002056,0.));
#33793=CARTESIAN_POINT('Ctrl Pts',(-15.7366025822956,-14.692131002056,18.));
#33794=CARTESIAN_POINT('Ctrl Pts',(-15.6542626345121,-14.6714990558793,
0.));
#33795=CARTESIAN_POINT('Ctrl Pts',(-15.6542626345121,-14.6714990558793,
18.));
#33796=CARTESIAN_POINT('Ctrl Pts',(-15.5722715494357,-14.6502440080911,
0.));
#33797=CARTESIAN_POINT('Ctrl Pts',(-15.5722715494357,-14.6502440080911,
18.));
#33798=CARTESIAN_POINT('Ctrl Pts',(-15.4906383406647,-14.6283600295736,
0.));
#33799=CARTESIAN_POINT('Ctrl Pts',(-15.4906383406647,-14.6283600295736,
18.));
#33800=CARTESIAN_POINT('Ctrl Pts',(-15.4093740621548,-14.6058389416146,
0.));
#33801=CARTESIAN_POINT('Ctrl Pts',(-15.4093740621548,-14.6058389416146,
18.));
#33802=CARTESIAN_POINT('Ctrl Pts',(-15.3284903715086,-14.5826719336929,
0.));
#33803=CARTESIAN_POINT('Ctrl Pts',(-15.3284903715086,-14.5826719336929,
18.));
#33804=CARTESIAN_POINT('Ctrl Pts',(-15.2479982823383,-14.5588510579962,
0.));
#33805=CARTESIAN_POINT('Ctrl Pts',(-15.2479982823383,-14.5588510579962,
18.));
#33806=CARTESIAN_POINT('Ctrl Pts',(-15.1679069808052,-14.534370647705,0.));
#33807=CARTESIAN_POINT('Ctrl Pts',(-15.1679069808052,-14.534370647705,18.));
#33808=CARTESIAN_POINT('Ctrl Pts',(-15.0882222764759,-14.5092291736391,
0.));
#33809=CARTESIAN_POINT('Ctrl Pts',(-15.0882222764759,-14.5092291736391,
18.));
#33810=CARTESIAN_POINT('Ctrl Pts',(-15.0089462280505,-14.4834296977405,
0.));
#33811=CARTESIAN_POINT('Ctrl Pts',(-15.0089462280505,-14.4834296977405,
18.));
#33812=CARTESIAN_POINT('Ctrl Pts',(-14.9300806580357,-14.4569756801697,
0.));
#33813=CARTESIAN_POINT('Ctrl Pts',(-14.9300806580357,-14.4569756801697,
18.));
#33814=CARTESIAN_POINT('Ctrl Pts',(-14.8516302160049,-14.4298673266313,
0.));
#33815=CARTESIAN_POINT('Ctrl Pts',(-14.8516302160049,-14.4298673266313,
18.));
#33816=CARTESIAN_POINT('Ctrl Pts',(-14.7736052248294,-14.4020981965564,
0.));
#33817=CARTESIAN_POINT('Ctrl Pts',(-14.7736052248294,-14.4020981965564,
18.));
#33818=CARTESIAN_POINT('Ctrl Pts',(-14.6960255561799,-14.3736505809735,
0.));
#33819=CARTESIAN_POINT('Ctrl Pts',(-14.6960255561799,-14.3736505809735,
18.));
#33820=CARTESIAN_POINT('Ctrl Pts',(-14.6189211183837,-14.3444949335274,
0.));
#33821=CARTESIAN_POINT('Ctrl Pts',(-14.6189211183837,-14.3444949335274,
18.));
#33822=CARTESIAN_POINT('Ctrl Pts',(-14.5423237181615,-14.3145996213697,
0.));
#33823=CARTESIAN_POINT('Ctrl Pts',(-14.5423237181615,-14.3145996213697,
18.));
#33824=CARTESIAN_POINT('Ctrl Pts',(-14.4662599802682,-14.2839394106401,
0.));
#33825=CARTESIAN_POINT('Ctrl Pts',(-14.4662599802682,-14.2839394106401,
18.));
#33826=CARTESIAN_POINT('Ctrl Pts',(-14.3907450096103,-14.2525030666863,
0.));
#33827=CARTESIAN_POINT('Ctrl Pts',(-14.3907450096103,-14.2525030666863,
18.));
#33828=CARTESIAN_POINT('Ctrl Pts',(-14.3157729256101,-14.2203046917613,
0.));
#33829=CARTESIAN_POINT('Ctrl Pts',(-14.3157729256101,-14.2203046917613,
18.));
#33830=CARTESIAN_POINT('Ctrl Pts',(-14.2413181097468,-14.1873822640681,
0.));
#33831=CARTESIAN_POINT('Ctrl Pts',(-14.2413181097468,-14.1873822640681,
18.));
#33832=CARTESIAN_POINT('Ctrl Pts',(-14.1673550455622,-14.1537739659715,
0.));
#33833=CARTESIAN_POINT('Ctrl Pts',(-14.1673550455622,-14.1537739659715,
18.));
#33834=CARTESIAN_POINT('Ctrl Pts',(-14.0938755647891,-14.1194976094444,
0.));
#33835=CARTESIAN_POINT('Ctrl Pts',(-14.0938755647891,-14.1194976094444,
18.));
#33836=CARTESIAN_POINT('Ctrl Pts',(-14.0209038736616,-14.0845327205726,
0.));
#33837=CARTESIAN_POINT('Ctrl Pts',(-14.0209038736616,-14.0845327205726,
18.));
#33838=CARTESIAN_POINT('Ctrl Pts',(-13.9485205009332,-14.0487919508068,
0.));
#33839=CARTESIAN_POINT('Ctrl Pts',(-13.9485205009332,-14.0487919508068,
18.));
#33840=CARTESIAN_POINT('Ctrl Pts',(-13.876852657608,-14.0121326766855,0.));
#33841=CARTESIAN_POINT('Ctrl Pts',(-13.876852657608,-14.0121326766855,18.));
#33842=CARTESIAN_POINT('Ctrl Pts',(-13.806028835706,-13.9744114225699,0.));
#33843=CARTESIAN_POINT('Ctrl Pts',(-13.806028835706,-13.9744114225699,18.));
#33844=CARTESIAN_POINT('Ctrl Pts',(-13.7361389175879,-13.9355316323567,
0.));
#33845=CARTESIAN_POINT('Ctrl Pts',(-13.7361389175879,-13.9355316323567,
18.));
#33846=CARTESIAN_POINT('Ctrl Pts',(-13.6672004242289,-13.8954842290745,
0.));
#33847=CARTESIAN_POINT('Ctrl Pts',(-13.6672004242289,-13.8954842290745,
18.));
#33848=CARTESIAN_POINT('Ctrl Pts',(-13.5991011046042,-13.854416158639,0.));
#33849=CARTESIAN_POINT('Ctrl Pts',(-13.5991011046042,-13.854416158639,18.));
#33850=CARTESIAN_POINT('Ctrl Pts',(-13.5316488646659,-13.8125718693898,
0.));
#33851=CARTESIAN_POINT('Ctrl Pts',(-13.5316488646659,-13.8125718693898,
18.));
#33852=CARTESIAN_POINT('Ctrl Pts',(-13.4646849459541,-13.7701598398937,
0.));
#33853=CARTESIAN_POINT('Ctrl Pts',(-13.4646849459541,-13.7701598398937,
18.));
#33854=CARTESIAN_POINT('Ctrl Pts',(-13.3981837093919,-13.7272351052346,
0.));
#33855=CARTESIAN_POINT('Ctrl Pts',(-13.3981837093919,-13.7272351052346,
18.));
#33856=CARTESIAN_POINT('Ctrl Pts',(-13.332345249068,-13.6835899659728,0.));
#33857=CARTESIAN_POINT('Ctrl Pts',(-13.332345249068,-13.6835899659728,18.));
#33858=CARTESIAN_POINT('Ctrl Pts',(-13.267724591625,-13.6386021757691,0.));
#33859=CARTESIAN_POINT('Ctrl Pts',(-13.267724591625,-13.6386021757691,18.));
#33860=CARTESIAN_POINT('Ctrl Pts',(-13.2050958591127,-13.5913916488449,
0.));
#33861=CARTESIAN_POINT('Ctrl Pts',(-13.2050958591127,-13.5913916488449,
18.));
#33862=CARTESIAN_POINT('Ctrl Pts',(-13.1572182238498,-13.5511230466604,
0.));
#33863=CARTESIAN_POINT('Ctrl Pts',(-13.1572182238498,-13.5511230466604,
18.));
#33864=CARTESIAN_POINT('Ctrl Pts',(-13.1228431405579,-13.5191927531554,
0.));
#33865=CARTESIAN_POINT('Ctrl Pts',(-13.1228431405579,-13.5191927531554,
18.));
#33866=CARTESIAN_POINT('Ctrl Pts',(-13.1006438497967,-13.4970961329957,
0.));
#33867=CARTESIAN_POINT('Ctrl Pts',(-13.1006438497967,-13.4970961329957,
18.));
#33868=CARTESIAN_POINT('Ctrl Pts',(-13.0897235660237,-13.4858453790958,
0.));
#33869=CARTESIAN_POINT('Ctrl Pts',(-13.0897235660237,-13.4858453790958,
18.));
#33870=CARTESIAN_POINT('',(-18.7025042402277,-15.040489857191,0.));
#33871=CARTESIAN_POINT('Ctrl Pts',(-13.0897235660237,-13.4858453790958,
0.));
#33872=CARTESIAN_POINT('Ctrl Pts',(-13.1006438497967,-13.4970961329957,
0.));
#33873=CARTESIAN_POINT('Ctrl Pts',(-13.1228431405579,-13.5191927531554,
0.));
#33874=CARTESIAN_POINT('Ctrl Pts',(-13.1572182238498,-13.5511230466604,
0.));
#33875=CARTESIAN_POINT('Ctrl Pts',(-13.2050958591127,-13.5913916488449,
0.));
#33876=CARTESIAN_POINT('Ctrl Pts',(-13.267724591625,-13.6386021757691,0.));
#33877=CARTESIAN_POINT('Ctrl Pts',(-13.332345249068,-13.6835899659728,0.));
#33878=CARTESIAN_POINT('Ctrl Pts',(-13.3981837093919,-13.7272351052346,
0.));
#33879=CARTESIAN_POINT('Ctrl Pts',(-13.4646849459541,-13.7701598398937,
0.));
#33880=CARTESIAN_POINT('Ctrl Pts',(-13.5316488646659,-13.8125718693898,
0.));
#33881=CARTESIAN_POINT('Ctrl Pts',(-13.5991011046042,-13.854416158639,0.));
#33882=CARTESIAN_POINT('Ctrl Pts',(-13.6672004242289,-13.8954842290745,
0.));
#33883=CARTESIAN_POINT('Ctrl Pts',(-13.7361389175879,-13.9355316323567,
0.));
#33884=CARTESIAN_POINT('Ctrl Pts',(-13.806028835706,-13.9744114225699,0.));
#33885=CARTESIAN_POINT('Ctrl Pts',(-13.876852657608,-14.0121326766855,0.));
#33886=CARTESIAN_POINT('Ctrl Pts',(-13.9485205009332,-14.0487919508068,
0.));
#33887=CARTESIAN_POINT('Ctrl Pts',(-14.0209038736616,-14.0845327205726,
0.));
#33888=CARTESIAN_POINT('Ctrl Pts',(-14.0938755647891,-14.1194976094444,
0.));
#33889=CARTESIAN_POINT('Ctrl Pts',(-14.1673550455622,-14.1537739659715,
0.));
#33890=CARTESIAN_POINT('Ctrl Pts',(-14.2413181097468,-14.1873822640681,
0.));
#33891=CARTESIAN_POINT('Ctrl Pts',(-14.3157729256101,-14.2203046917613,
0.));
#33892=CARTESIAN_POINT('Ctrl Pts',(-14.3907450096103,-14.2525030666863,
0.));
#33893=CARTESIAN_POINT('Ctrl Pts',(-14.4662599802682,-14.2839394106401,
0.));
#33894=CARTESIAN_POINT('Ctrl Pts',(-14.5423237181615,-14.3145996213697,
0.));
#33895=CARTESIAN_POINT('Ctrl Pts',(-14.6189211183837,-14.3444949335274,
0.));
#33896=CARTESIAN_POINT('Ctrl Pts',(-14.6960255561799,-14.3736505809735,
0.));
#33897=CARTESIAN_POINT('Ctrl Pts',(-14.7736052248294,-14.4020981965564,
0.));
#33898=CARTESIAN_POINT('Ctrl Pts',(-14.8516302160049,-14.4298673266313,
0.));
#33899=CARTESIAN_POINT('Ctrl Pts',(-14.9300806580357,-14.4569756801697,
0.));
#33900=CARTESIAN_POINT('Ctrl Pts',(-15.0089462280505,-14.4834296977405,
0.));
#33901=CARTESIAN_POINT('Ctrl Pts',(-15.0882222764759,-14.5092291736391,
0.));
#33902=CARTESIAN_POINT('Ctrl Pts',(-15.1679069808052,-14.534370647705,0.));
#33903=CARTESIAN_POINT('Ctrl Pts',(-15.2479982823383,-14.5588510579962,
0.));
#33904=CARTESIAN_POINT('Ctrl Pts',(-15.3284903715086,-14.5826719336929,
0.));
#33905=CARTESIAN_POINT('Ctrl Pts',(-15.4093740621548,-14.6058389416146,
0.));
#33906=CARTESIAN_POINT('Ctrl Pts',(-15.4906383406647,-14.6283600295736,
0.));
#33907=CARTESIAN_POINT('Ctrl Pts',(-15.5722715494357,-14.6502440080911,
0.));
#33908=CARTESIAN_POINT('Ctrl Pts',(-15.6542626345121,-14.6714990558793,
0.));
#33909=CARTESIAN_POINT('Ctrl Pts',(-15.7366025822956,-14.692131002056,0.));
#33910=CARTESIAN_POINT('Ctrl Pts',(-15.8192842036838,-14.7121435744495,
0.));
#33911=CARTESIAN_POINT('Ctrl Pts',(-15.9023014613802,-14.7315391924939,
0.));
#33912=CARTESIAN_POINT('Ctrl Pts',(-15.9856489347991,-14.7503195973741,
0.));
#33913=CARTESIAN_POINT('Ctrl Pts',(-16.0693212651732,-14.7684865075326,
0.));
#33914=CARTESIAN_POINT('Ctrl Pts',(-16.1533125058853,-14.7860423865308,
0.));
#33915=CARTESIAN_POINT('Ctrl Pts',(-16.2376161919272,-14.8029903659562,
0.));
#33916=CARTESIAN_POINT('Ctrl Pts',(-16.3222256264574,-14.8193339134125,
0.));
#33917=CARTESIAN_POINT('Ctrl Pts',(-16.4071341001481,-14.8350765822692,
0.));
#33918=CARTESIAN_POINT('Ctrl Pts',(-16.492335117066,-14.8502217520165,0.));
#33919=CARTESIAN_POINT('Ctrl Pts',(-16.5778226646614,-14.8647723257055,
0.));
#33920=CARTESIAN_POINT('Ctrl Pts',(-16.6635911790385,-14.8787307479454,
0.));
#33921=CARTESIAN_POINT('Ctrl Pts',(-16.7496353900706,-14.8920991518626,
0.));
#33922=CARTESIAN_POINT('Ctrl Pts',(-16.8359501981915,-14.9048794721647,
0.));
#33923=CARTESIAN_POINT('Ctrl Pts',(-16.9225305499155,-14.9170735658747,
0.));
#33924=CARTESIAN_POINT('Ctrl Pts',(-17.0093712776822,-14.9286833603319,
0.));
#33925=CARTESIAN_POINT('Ctrl Pts',(-17.0964671184813,-14.9397108660998,
0.));
#33926=CARTESIAN_POINT('Ctrl Pts',(-17.1838128327073,-14.9501581118289,
0.));
#33927=CARTESIAN_POINT('Ctrl Pts',(-17.2714032968314,-14.9600271060471,
0.));
#33928=CARTESIAN_POINT('Ctrl Pts',(-17.3592335908103,-14.9693197947387,
0.));
#33929=CARTESIAN_POINT('Ctrl Pts',(-17.4472991215239,-14.9780380183576,
0.));
#33930=CARTESIAN_POINT('Ctrl Pts',(-17.5355955872257,-14.9861834999847,
0.));
#33931=CARTESIAN_POINT('Ctrl Pts',(-17.6241187988652,-14.9937578646616,
0.));
#33932=CARTESIAN_POINT('Ctrl Pts',(-17.7128645299878,-15.0007626541286,
0.));
#33933=CARTESIAN_POINT('Ctrl Pts',(-17.8018283748074,-15.0071993464636,
0.));
#33934=CARTESIAN_POINT('Ctrl Pts',(-17.891005548971,-15.0130693803259,0.));
#33935=CARTESIAN_POINT('Ctrl Pts',(-17.980390892286,-15.0183741723687,0.));
#33936=CARTESIAN_POINT('Ctrl Pts',(-18.0699792164192,-15.0231151183906,
0.));
#33937=CARTESIAN_POINT('Ctrl Pts',(-18.1597655779328,-15.0272936035154,
0.));
#33938=CARTESIAN_POINT('Ctrl Pts',(-18.2497455679917,-15.0309110092482,
0.));
#33939=CARTESIAN_POINT('Ctrl Pts',(-18.3399156227477,-15.0339687345357,
0.));
#33940=CARTESIAN_POINT('Ctrl Pts',(-18.4483447600234,-15.036968080037,0.));
#33941=CARTESIAN_POINT('Ctrl Pts',(-18.5389347492702,-15.0387713100259,
0.));
#33942=CARTESIAN_POINT('Ctrl Pts',(-18.6115544313469,-15.0397694451467,
0.));
#33943=CARTESIAN_POINT('Ctrl Pts',(-18.6661021851765,-15.0402682932585,
0.));
#33944=CARTESIAN_POINT('Ctrl Pts',(-18.7025042402277,-15.040489857191,0.));
#33945=CARTESIAN_POINT('',(-18.7025042402277,-15.040489857191,15.));
#33946=CARTESIAN_POINT('Ctrl Pts',(-18.7025042402277,-15.040489857191,15.));
#33947=CARTESIAN_POINT('Ctrl Pts',(-18.6843032127312,-15.0403790752228,
15.));
#33948=CARTESIAN_POINT('Ctrl Pts',(-18.6479196005666,-15.0401020105546,
15.));
#33949=CARTESIAN_POINT('Ctrl Pts',(-18.5933995108277,-15.0395199113665,
15.));
#33950=CARTESIAN_POINT('Ctrl Pts',(-18.5208167514208,-15.0384106640281,
15.));
#33951=CARTESIAN_POINT('Ctrl Pts',(-18.4302732371441,-15.0364681891201,
15.));
#33952=CARTESIAN_POINT('Ctrl Pts',(-18.3399156227477,-15.0339687345357,
15.));
#33953=CARTESIAN_POINT('Ctrl Pts',(-18.2497455679917,-15.0309110092482,
15.));
#33954=CARTESIAN_POINT('Ctrl Pts',(-18.1597655779328,-15.0272936035154,
15.));
#33955=CARTESIAN_POINT('Ctrl Pts',(-18.0699792164192,-15.0231151183906,
15.));
#33956=CARTESIAN_POINT('Ctrl Pts',(-17.980390892286,-15.0183741723687,15.));
#33957=CARTESIAN_POINT('Ctrl Pts',(-17.891005548971,-15.0130693803259,15.));
#33958=CARTESIAN_POINT('Ctrl Pts',(-17.8018283748074,-15.0071993464636,
15.));
#33959=CARTESIAN_POINT('Ctrl Pts',(-17.7128645299878,-15.0007626541286,
15.));
#33960=CARTESIAN_POINT('Ctrl Pts',(-17.6241187988652,-14.9937578646616,
15.));
#33961=CARTESIAN_POINT('Ctrl Pts',(-17.5355955872257,-14.9861834999847,
15.));
#33962=CARTESIAN_POINT('Ctrl Pts',(-17.4472991215239,-14.9780380183576,
15.));
#33963=CARTESIAN_POINT('Ctrl Pts',(-17.3592335908103,-14.9693197947387,
15.));
#33964=CARTESIAN_POINT('Ctrl Pts',(-17.2714032968314,-14.9600271060471,
15.));
#33965=CARTESIAN_POINT('Ctrl Pts',(-17.1838128327073,-14.9501581118289,
15.));
#33966=CARTESIAN_POINT('Ctrl Pts',(-17.0964671184813,-14.9397108660998,
15.));
#33967=CARTESIAN_POINT('Ctrl Pts',(-17.0093712776822,-14.9286833603319,
15.));
#33968=CARTESIAN_POINT('Ctrl Pts',(-16.9225305499155,-14.9170735658747,
15.));
#33969=CARTESIAN_POINT('Ctrl Pts',(-16.8359501981915,-14.9048794721647,
15.));
#33970=CARTESIAN_POINT('Ctrl Pts',(-16.7496353900706,-14.8920991518626,
15.));
#33971=CARTESIAN_POINT('Ctrl Pts',(-16.6635911790385,-14.8787307479454,
15.));
#33972=CARTESIAN_POINT('Ctrl Pts',(-16.5778226646614,-14.8647723257055,
15.));
#33973=CARTESIAN_POINT('Ctrl Pts',(-16.492335117066,-14.8502217520165,15.));
#33974=CARTESIAN_POINT('Ctrl Pts',(-16.4071341001481,-14.8350765822692,
15.));
#33975=CARTESIAN_POINT('Ctrl Pts',(-16.3222256264574,-14.8193339134125,
15.));
#33976=CARTESIAN_POINT('Ctrl Pts',(-16.2376161919272,-14.8029903659562,
15.));
#33977=CARTESIAN_POINT('Ctrl Pts',(-16.1533125058853,-14.7860423865308,
15.));
#33978=CARTESIAN_POINT('Ctrl Pts',(-16.0693212651732,-14.7684865075326,
15.));
#33979=CARTESIAN_POINT('Ctrl Pts',(-15.9856489347991,-14.7503195973741,
15.));
#33980=CARTESIAN_POINT('Ctrl Pts',(-15.9023014613802,-14.7315391924939,
15.));
#33981=CARTESIAN_POINT('Ctrl Pts',(-15.8192842036838,-14.7121435744495,
15.));
#33982=CARTESIAN_POINT('Ctrl Pts',(-15.7366025822956,-14.692131002056,15.));
#33983=CARTESIAN_POINT('Ctrl Pts',(-15.6542626345121,-14.6714990558793,
15.));
#33984=CARTESIAN_POINT('Ctrl Pts',(-15.5722715494357,-14.6502440080911,
15.));
#33985=CARTESIAN_POINT('Ctrl Pts',(-15.4906383406647,-14.6283600295736,
15.));
#33986=CARTESIAN_POINT('Ctrl Pts',(-15.4093740621548,-14.6058389416146,
15.));
#33987=CARTESIAN_POINT('Ctrl Pts',(-15.3284903715086,-14.5826719336929,
15.));
#33988=CARTESIAN_POINT('Ctrl Pts',(-15.2479982823383,-14.5588510579962,
15.));
#33989=CARTESIAN_POINT('Ctrl Pts',(-15.1679069808052,-14.534370647705,15.));
#33990=CARTESIAN_POINT('Ctrl Pts',(-15.0882222764759,-14.5092291736391,
15.));
#33991=CARTESIAN_POINT('Ctrl Pts',(-15.0089462280505,-14.4834296977405,
15.));
#33992=CARTESIAN_POINT('Ctrl Pts',(-14.9300806580357,-14.4569756801697,
15.));
#33993=CARTESIAN_POINT('Ctrl Pts',(-14.8516302160049,-14.4298673266313,
15.));
#33994=CARTESIAN_POINT('Ctrl Pts',(-14.7736052248294,-14.4020981965564,
15.));
#33995=CARTESIAN_POINT('Ctrl Pts',(-14.6960255561799,-14.3736505809735,
15.));
#33996=CARTESIAN_POINT('Ctrl Pts',(-14.6189211183837,-14.3444949335274,
15.));
#33997=CARTESIAN_POINT('Ctrl Pts',(-14.5423237181615,-14.3145996213697,
15.));
#33998=CARTESIAN_POINT('Ctrl Pts',(-14.4662599802682,-14.2839394106401,
15.));
#33999=CARTESIAN_POINT('Ctrl Pts',(-14.3907450096103,-14.2525030666863,
15.));
#34000=CARTESIAN_POINT('Ctrl Pts',(-14.3157729256101,-14.2203046917613,
15.));
#34001=CARTESIAN_POINT('Ctrl Pts',(-14.2413181097468,-14.1873822640681,
15.));
#34002=CARTESIAN_POINT('Ctrl Pts',(-14.1673550455622,-14.1537739659715,
15.));
#34003=CARTESIAN_POINT('Ctrl Pts',(-14.0938755647891,-14.1194976094444,
15.));
#34004=CARTESIAN_POINT('Ctrl Pts',(-14.0209038736616,-14.0845327205726,
15.));
#34005=CARTESIAN_POINT('Ctrl Pts',(-13.9485205009332,-14.0487919508068,
15.));
#34006=CARTESIAN_POINT('Ctrl Pts',(-13.876852657608,-14.0121326766855,15.));
#34007=CARTESIAN_POINT('Ctrl Pts',(-13.806028835706,-13.9744114225699,15.));
#34008=CARTESIAN_POINT('Ctrl Pts',(-13.7361389175879,-13.9355316323567,
15.));
#34009=CARTESIAN_POINT('Ctrl Pts',(-13.6672004242289,-13.8954842290745,
15.));
#34010=CARTESIAN_POINT('Ctrl Pts',(-13.5991011046042,-13.854416158639,15.));
#34011=CARTESIAN_POINT('Ctrl Pts',(-13.5316488646659,-13.8125718693898,
15.));
#34012=CARTESIAN_POINT('Ctrl Pts',(-13.4646849459541,-13.7701598398937,
15.));
#34013=CARTESIAN_POINT('Ctrl Pts',(-13.3981837093919,-13.7272351052346,
15.));
#34014=CARTESIAN_POINT('Ctrl Pts',(-13.332345249068,-13.6835899659728,15.));
#34015=CARTESIAN_POINT('Ctrl Pts',(-13.267724591625,-13.6386021757691,15.));
#34016=CARTESIAN_POINT('Ctrl Pts',(-13.2050958591127,-13.5913916488449,
15.));
#34017=CARTESIAN_POINT('Ctrl Pts',(-13.1572182238498,-13.5511230466604,
15.));
#34018=CARTESIAN_POINT('Ctrl Pts',(-13.1228431405579,-13.5191927531554,
15.));
#34019=CARTESIAN_POINT('Ctrl Pts',(-13.1006438497967,-13.4970961329957,
15.));
#34020=CARTESIAN_POINT('Ctrl Pts',(-13.0897235660237,-13.4858453790958,
15.));
#34021=CARTESIAN_POINT('',(-18.7025042402277,-15.040489857191,0.));
#34022=CARTESIAN_POINT('Origin',(-9.34524724197226E-14,-6.78114261146376E-14,
0.));
#34023=CARTESIAN_POINT('',(-20.0837475345526,-13.1393715591102,0.));
#34024=CARTESIAN_POINT('Origin',(-9.34524724197226E-14,-6.78114261146376E-14,
0.));
#34025=CARTESIAN_POINT('',(-20.0837475345526,-13.1393715591102,15.));
#34026=CARTESIAN_POINT('Origin',(-9.34524724197226E-14,-6.78114261146376E-14,
15.));
#34027=CARTESIAN_POINT('',(-20.0837475345526,-13.1393715591102,0.));
#34028=CARTESIAN_POINT('Ctrl Pts',(-16.8707481591095,-8.28171148831561,
0.));
#34029=CARTESIAN_POINT('Ctrl Pts',(-16.8707481591095,-8.28171148831561,
18.));
#34030=CARTESIAN_POINT('Ctrl Pts',(-16.8848228151885,-8.28862062120314,
0.));
#34031=CARTESIAN_POINT('Ctrl Pts',(-16.8848228151885,-8.28862062120314,
18.));
#34032=CARTESIAN_POINT('Ctrl Pts',(-16.9126979078877,-8.30290517019115,
0.));
#34033=CARTESIAN_POINT('Ctrl Pts',(-16.9126979078877,-8.30290517019115,
18.));
#34034=CARTESIAN_POINT('Ctrl Pts',(-16.9536879065132,-8.32573081382562,
0.));
#34035=CARTESIAN_POINT('Ctrl Pts',(-16.9536879065132,-8.32573081382562,
18.));
#34036=CARTESIAN_POINT('Ctrl Pts',(-17.0067806259695,-8.35882146841243,
0.));
#34037=CARTESIAN_POINT('Ctrl Pts',(-17.0067806259695,-8.35882146841243,
18.));
#34038=CARTESIAN_POINT('Ctrl Pts',(-17.071033847921,-8.40379607744265,0.));
#34039=CARTESIAN_POINT('Ctrl Pts',(-17.071033847921,-8.40379607744265,18.));
#34040=CARTESIAN_POINT('Ctrl Pts',(-17.1337886602855,-8.45135198307876,
0.));
#34041=CARTESIAN_POINT('Ctrl Pts',(-17.1337886602855,-8.45135198307876,
18.));
#34042=CARTESIAN_POINT('Ctrl Pts',(-17.1956428575086,-8.50048099003882,
0.));
#34043=CARTESIAN_POINT('Ctrl Pts',(-17.1956428575086,-8.50048099003882,
18.));
#34044=CARTESIAN_POINT('Ctrl Pts',(-17.2570167183611,-8.55046295192433,
0.));
#34045=CARTESIAN_POINT('Ctrl Pts',(-17.2570167183611,-8.55046295192433,
18.));
#34046=CARTESIAN_POINT('Ctrl Pts',(-17.3180459442745,-8.60104338529165,
0.));
#34047=CARTESIAN_POINT('Ctrl Pts',(-17.3180459442745,-8.60104338529165,
18.));
#34048=CARTESIAN_POINT('Ctrl Pts',(-17.3786861166843,-8.65226368112815,
0.));
#34049=CARTESIAN_POINT('Ctrl Pts',(-17.3786861166843,-8.65226368112815,
18.));
#34050=CARTESIAN_POINT('Ctrl Pts',(-17.438788019753,-8.70433925112174,0.));
#34051=CARTESIAN_POINT('Ctrl Pts',(-17.438788019753,-8.70433925112174,18.));
#34052=CARTESIAN_POINT('Ctrl Pts',(-17.4981785296199,-8.75752832625954,
0.));
#34053=CARTESIAN_POINT('Ctrl Pts',(-17.4981785296199,-8.75752832625954,
18.));
#34054=CARTESIAN_POINT('Ctrl Pts',(-17.5567525798882,-8.8119830723955,0.));
#34055=CARTESIAN_POINT('Ctrl Pts',(-17.5567525798882,-8.8119830723955,18.));
#34056=CARTESIAN_POINT('Ctrl Pts',(-17.614513388992,-8.86768402115343,0.));
#34057=CARTESIAN_POINT('Ctrl Pts',(-17.614513388992,-8.86768402115343,18.));
#34058=CARTESIAN_POINT('Ctrl Pts',(-17.6715250120654,-8.92451585185175,
0.));
#34059=CARTESIAN_POINT('Ctrl Pts',(-17.6715250120654,-8.92451585185175,
18.));
#34060=CARTESIAN_POINT('Ctrl Pts',(-17.7278841963319,-8.98231202490685,
0.));
#34061=CARTESIAN_POINT('Ctrl Pts',(-17.7278841963319,-8.98231202490685,
18.));
#34062=CARTESIAN_POINT('Ctrl Pts',(-17.7836872744016,-9.04090748239097,
0.));
#34063=CARTESIAN_POINT('Ctrl Pts',(-17.7836872744016,-9.04090748239097,
18.));
#34064=CARTESIAN_POINT('Ctrl Pts',(-17.8389924349283,-9.10019864472208,
0.));
#34065=CARTESIAN_POINT('Ctrl Pts',(-17.8389924349283,-9.10019864472208,
18.));
#34066=CARTESIAN_POINT('Ctrl Pts',(-17.8938116696237,-9.16015616361609,
0.));
#34067=CARTESIAN_POINT('Ctrl Pts',(-17.8938116696237,-9.16015616361609,
18.));
#34068=CARTESIAN_POINT('Ctrl Pts',(-17.9481305624284,-9.22079331175917,
0.));
#34069=CARTESIAN_POINT('Ctrl Pts',(-17.9481305624284,-9.22079331175917,
18.));
#34070=CARTESIAN_POINT('Ctrl Pts',(-18.0019206847747,-9.2821461557447,0.));
#34071=CARTESIAN_POINT('Ctrl Pts',(-18.0019206847747,-9.2821461557447,18.));
#34072=CARTESIAN_POINT('Ctrl Pts',(-18.0551538338035,-9.34425079614395,
0.));
#34073=CARTESIAN_POINT('Ctrl Pts',(-18.0551538338035,-9.34425079614395,
18.));
#34074=CARTESIAN_POINT('Ctrl Pts',(-18.1078184146735,-9.40711718355464,
0.));
#34075=CARTESIAN_POINT('Ctrl Pts',(-18.1078184146735,-9.40711718355464,
18.));
#34076=CARTESIAN_POINT('Ctrl Pts',(-18.1599204445014,-9.47072748065831,
0.));
#34077=CARTESIAN_POINT('Ctrl Pts',(-18.1599204445014,-9.47072748065831,
18.));
#34078=CARTESIAN_POINT('Ctrl Pts',(-18.2114756946126,-9.53504856811685,
0.));
#34079=CARTESIAN_POINT('Ctrl Pts',(-18.2114756946126,-9.53504856811685,
18.));
#34080=CARTESIAN_POINT('Ctrl Pts',(-18.2625044208165,-9.60004042085346,
0.));
#34081=CARTESIAN_POINT('Ctrl Pts',(-18.2625044208165,-9.60004042085346,
18.));
#34082=CARTESIAN_POINT('Ctrl Pts',(-18.3130254811852,-9.66566546403259,
0.));
#34083=CARTESIAN_POINT('Ctrl Pts',(-18.3130254811852,-9.66566546403259,
18.));
#34084=CARTESIAN_POINT('Ctrl Pts',(-18.3630495772677,-9.73189932619939,
0.));
#34085=CARTESIAN_POINT('Ctrl Pts',(-18.3630495772677,-9.73189932619939,
18.));
#34086=CARTESIAN_POINT('Ctrl Pts',(-18.4125796444662,-9.79873019947433,
0.));
#34087=CARTESIAN_POINT('Ctrl Pts',(-18.4125796444662,-9.79873019947433,
18.));
#34088=CARTESIAN_POINT('Ctrl Pts',(-18.461614050347,-9.86615372541684,0.));
#34089=CARTESIAN_POINT('Ctrl Pts',(-18.461614050347,-9.86615372541684,18.));
#34090=CARTESIAN_POINT('Ctrl Pts',(-18.5101489409161,-9.93416923996828,
0.));
#34091=CARTESIAN_POINT('Ctrl Pts',(-18.5101489409161,-9.93416923996828,
18.));
#34092=CARTESIAN_POINT('Ctrl Pts',(-18.5581807679204,-10.0027757313807,
0.));
#34093=CARTESIAN_POINT('Ctrl Pts',(-18.5581807679204,-10.0027757313807,
18.));
#34094=CARTESIAN_POINT('Ctrl Pts',(-18.605709190442,-10.0719672018851,0.));
#34095=CARTESIAN_POINT('Ctrl Pts',(-18.605709190442,-10.0719672018851,18.));
#34096=CARTESIAN_POINT('Ctrl Pts',(-18.6527367592664,-10.1417331637795,
0.));
#34097=CARTESIAN_POINT('Ctrl Pts',(-18.6527367592664,-10.1417331637795,
18.));
#34098=CARTESIAN_POINT('Ctrl Pts',(-18.699267629819,-10.2120606864872,0.));
#34099=CARTESIAN_POINT('Ctrl Pts',(-18.699267629819,-10.2120606864872,18.));
#34100=CARTESIAN_POINT('Ctrl Pts',(-18.7453065790062,-10.2829359603685,
0.));
#34101=CARTESIAN_POINT('Ctrl Pts',(-18.7453065790062,-10.2829359603685,
18.));
#34102=CARTESIAN_POINT('Ctrl Pts',(-18.7908579693851,-10.3543459451258,
0.));
#34103=CARTESIAN_POINT('Ctrl Pts',(-18.7908579693851,-10.3543459451258,
18.));
#34104=CARTESIAN_POINT('Ctrl Pts',(-18.8359245594214,-10.4262802670211,
0.));
#34105=CARTESIAN_POINT('Ctrl Pts',(-18.8359245594214,-10.4262802670211,
18.));
#34106=CARTESIAN_POINT('Ctrl Pts',(-18.8805076729356,-10.4987309368494,
0.));
#34107=CARTESIAN_POINT('Ctrl Pts',(-18.8805076729356,-10.4987309368494,
18.));
#34108=CARTESIAN_POINT('Ctrl Pts',(-18.9246077453188,-10.5716914651544,
0.));
#34109=CARTESIAN_POINT('Ctrl Pts',(-18.9246077453188,-10.5716914651544,
18.));
#34110=CARTESIAN_POINT('Ctrl Pts',(-18.9682247574834,-10.6451561585969,
0.));
#34111=CARTESIAN_POINT('Ctrl Pts',(-18.9682247574834,-10.6451561585969,
18.));
#34112=CARTESIAN_POINT('Ctrl Pts',(-19.0113586878152,-10.7191193896586,
0.));
#34113=CARTESIAN_POINT('Ctrl Pts',(-19.0113586878152,-10.7191193896586,
18.));
#34114=CARTESIAN_POINT('Ctrl Pts',(-19.0540100416943,-10.7935747414879,
0.));
#34115=CARTESIAN_POINT('Ctrl Pts',(-19.0540100416943,-10.7935747414879,
18.));
#34116=CARTESIAN_POINT('Ctrl Pts',(-19.0961797996403,-10.868515097783,0.));
#34117=CARTESIAN_POINT('Ctrl Pts',(-19.0961797996403,-10.868515097783,18.));
#34118=CARTESIAN_POINT('Ctrl Pts',(-19.1378691901023,-10.9439330179206,
0.));
#34119=CARTESIAN_POINT('Ctrl Pts',(-19.1378691901023,-10.9439330179206,
18.));
#34120=CARTESIAN_POINT('Ctrl Pts',(-19.1790795192393,-11.0198210228993,
0.));
#34121=CARTESIAN_POINT('Ctrl Pts',(-19.1790795192393,-11.0198210228993,
18.));
#34122=CARTESIAN_POINT('Ctrl Pts',(-19.2198119937835,-11.0961718903994,
0.));
#34123=CARTESIAN_POINT('Ctrl Pts',(-19.2198119937835,-11.0961718903994,
18.));
#34124=CARTESIAN_POINT('Ctrl Pts',(-19.2600675167206,-11.1729790050543,
0.));
#34125=CARTESIAN_POINT('Ctrl Pts',(-19.2600675167206,-11.1729790050543,
18.));
#34126=CARTESIAN_POINT('Ctrl Pts',(-19.2998466936739,-11.2502363198588,
0.));
#34127=CARTESIAN_POINT('Ctrl Pts',(-19.2998466936739,-11.2502363198588,
18.));
#34128=CARTESIAN_POINT('Ctrl Pts',(-19.3391499248083,-11.3279381634523,
0.));
#34129=CARTESIAN_POINT('Ctrl Pts',(-19.3391499248083,-11.3279381634523,
18.));
#34130=CARTESIAN_POINT('Ctrl Pts',(-19.3779774742876,-11.4060790880015,
0.));
#34131=CARTESIAN_POINT('Ctrl Pts',(-19.3779774742876,-11.4060790880015,
18.));
#34132=CARTESIAN_POINT('Ctrl Pts',(-19.4163295466324,-11.4846537135043,
0.));
#34133=CARTESIAN_POINT('Ctrl Pts',(-19.4163295466324,-11.4846537135043,
18.));
#34134=CARTESIAN_POINT('Ctrl Pts',(-19.4542063779876,-11.5636565297382,
0.));
#34135=CARTESIAN_POINT('Ctrl Pts',(-19.4542063779876,-11.5636565297382,
18.));
#34136=CARTESIAN_POINT('Ctrl Pts',(-19.4916082541529,-11.6430819099846,
0.));
#34137=CARTESIAN_POINT('Ctrl Pts',(-19.4916082541529,-11.6430819099846,
18.));
#34138=CARTESIAN_POINT('Ctrl Pts',(-19.5285354853626,-11.722924244195,0.));
#34139=CARTESIAN_POINT('Ctrl Pts',(-19.5285354853626,-11.722924244195,18.));
#34140=CARTESIAN_POINT('Ctrl Pts',(-19.5649883985826,-11.8031780389346,
0.));
#34141=CARTESIAN_POINT('Ctrl Pts',(-19.5649883985826,-11.8031780389346,
18.));
#34142=CARTESIAN_POINT('Ctrl Pts',(-19.6009673241771,-11.8838380136222,
0.));
#34143=CARTESIAN_POINT('Ctrl Pts',(-19.6009673241771,-11.8838380136222,
18.));
#34144=CARTESIAN_POINT('Ctrl Pts',(-19.6364725931695,-11.9648992312094,
0.));
#34145=CARTESIAN_POINT('Ctrl Pts',(-19.6364725931695,-11.9648992312094,
18.));
#34146=CARTESIAN_POINT('Ctrl Pts',(-19.6715045149944,-12.0463570680308,
0.));
#34147=CARTESIAN_POINT('Ctrl Pts',(-19.6715045149944,-12.0463570680308,
18.));
#34148=CARTESIAN_POINT('Ctrl Pts',(-19.7060633406705,-12.1282070378972,
0.));
#34149=CARTESIAN_POINT('Ctrl Pts',(-19.7060633406705,-12.1282070378972,
18.));
#34150=CARTESIAN_POINT('Ctrl Pts',(-19.7401492304335,-12.2104446447874,
0.));
#34151=CARTESIAN_POINT('Ctrl Pts',(-19.7401492304335,-12.2104446447874,
18.));
#34152=CARTESIAN_POINT('Ctrl Pts',(-19.7737622285562,-12.2930652417986,
0.));
#34153=CARTESIAN_POINT('Ctrl Pts',(-19.7737622285562,-12.2930652417986,
18.));
#34154=CARTESIAN_POINT('Ctrl Pts',(-19.8069022248387,-12.3760638341708,
0.));
#34155=CARTESIAN_POINT('Ctrl Pts',(-19.8069022248387,-12.3760638341708,
18.));
#34156=CARTESIAN_POINT('Ctrl Pts',(-19.839568972011,-12.4594350764989,0.));
#34157=CARTESIAN_POINT('Ctrl Pts',(-19.839568972011,-12.4594350764989,18.));
#34158=CARTESIAN_POINT('Ctrl Pts',(-19.8717621942733,-12.5431736030595,
0.));
#34159=CARTESIAN_POINT('Ctrl Pts',(-19.8717621942733,-12.5431736030595,
18.));
#34160=CARTESIAN_POINT('Ctrl Pts',(-19.9034816813503,-12.6272742843372,
0.));
#34161=CARTESIAN_POINT('Ctrl Pts',(-19.9034816813503,-12.6272742843372,
18.));
#34162=CARTESIAN_POINT('Ctrl Pts',(-19.9347273847264,-12.7117325003719,
0.));
#34163=CARTESIAN_POINT('Ctrl Pts',(-19.9347273847264,-12.7117325003719,
18.));
#34164=CARTESIAN_POINT('Ctrl Pts',(-19.9654995335894,-12.7965444294443,
0.));
#34165=CARTESIAN_POINT('Ctrl Pts',(-19.9654995335894,-12.7965444294443,
18.));
#34166=CARTESIAN_POINT('Ctrl Pts',(-19.9957986945787,-12.8817072534696,
0.));
#34167=CARTESIAN_POINT('Ctrl Pts',(-19.9957986945787,-12.8817072534696,
18.));
#34168=CARTESIAN_POINT('Ctrl Pts',(-20.0256255826397,-12.9672189949731,
0.));
#34169=CARTESIAN_POINT('Ctrl Pts',(-20.0256255826397,-12.9672189949731,
18.));
#34170=CARTESIAN_POINT('Ctrl Pts',(-20.0491098457044,-13.0359065249991,
0.));
#34171=CARTESIAN_POINT('Ctrl Pts',(-20.0491098457044,-13.0359065249991,
18.));
#34172=CARTESIAN_POINT('Ctrl Pts',(-20.0665110891946,-13.0875783330728,
0.));
#34173=CARTESIAN_POINT('Ctrl Pts',(-20.0665110891946,-13.0875783330728,
18.));
#34174=CARTESIAN_POINT('Ctrl Pts',(-20.0780177478283,-13.1220955868173,
0.));
#34175=CARTESIAN_POINT('Ctrl Pts',(-20.0780177478283,-13.1220955868173,
18.));
#34176=CARTESIAN_POINT('Ctrl Pts',(-20.0837475345526,-13.1393715591102,
0.));
#34177=CARTESIAN_POINT('Ctrl Pts',(-20.0837475345526,-13.1393715591102,
18.));
#34178=CARTESIAN_POINT('Ctrl Pts',(-16.8707481591095,-8.28171148831561,
0.));
#34179=CARTESIAN_POINT('Ctrl Pts',(-16.8848228151885,-8.28862062120314,
0.));
#34180=CARTESIAN_POINT('Ctrl Pts',(-16.9126979078877,-8.30290517019115,
0.));
#34181=CARTESIAN_POINT('Ctrl Pts',(-16.9536879065132,-8.32573081382562,
0.));
#34182=CARTESIAN_POINT('Ctrl Pts',(-17.0067806259695,-8.35882146841243,
0.));
#34183=CARTESIAN_POINT('Ctrl Pts',(-17.071033847921,-8.40379607744265,0.));
#34184=CARTESIAN_POINT('Ctrl Pts',(-17.1337886602855,-8.45135198307876,
0.));
#34185=CARTESIAN_POINT('Ctrl Pts',(-17.1956428575086,-8.50048099003882,
0.));
#34186=CARTESIAN_POINT('Ctrl Pts',(-17.2570167183611,-8.55046295192433,
0.));
#34187=CARTESIAN_POINT('Ctrl Pts',(-17.3180459442745,-8.60104338529165,
0.));
#34188=CARTESIAN_POINT('Ctrl Pts',(-17.3786861166843,-8.65226368112815,
0.));
#34189=CARTESIAN_POINT('Ctrl Pts',(-17.438788019753,-8.70433925112174,0.));
#34190=CARTESIAN_POINT('Ctrl Pts',(-17.4981785296199,-8.75752832625954,
0.));
#34191=CARTESIAN_POINT('Ctrl Pts',(-17.5567525798882,-8.8119830723955,0.));
#34192=CARTESIAN_POINT('Ctrl Pts',(-17.614513388992,-8.86768402115343,0.));
#34193=CARTESIAN_POINT('Ctrl Pts',(-17.6715250120654,-8.92451585185175,
0.));
#34194=CARTESIAN_POINT('Ctrl Pts',(-17.7278841963319,-8.98231202490685,
0.));
#34195=CARTESIAN_POINT('Ctrl Pts',(-17.7836872744016,-9.04090748239097,
0.));
#34196=CARTESIAN_POINT('Ctrl Pts',(-17.8389924349283,-9.10019864472208,
0.));
#34197=CARTESIAN_POINT('Ctrl Pts',(-17.8938116696237,-9.16015616361609,
0.));
#34198=CARTESIAN_POINT('Ctrl Pts',(-17.9481305624284,-9.22079331175917,
0.));
#34199=CARTESIAN_POINT('Ctrl Pts',(-18.0019206847747,-9.2821461557447,0.));
#34200=CARTESIAN_POINT('Ctrl Pts',(-18.0551538338035,-9.34425079614395,
0.));
#34201=CARTESIAN_POINT('Ctrl Pts',(-18.1078184146735,-9.40711718355464,
0.));
#34202=CARTESIAN_POINT('Ctrl Pts',(-18.1599204445014,-9.47072748065831,
0.));
#34203=CARTESIAN_POINT('Ctrl Pts',(-18.2114756946126,-9.53504856811685,
0.));
#34204=CARTESIAN_POINT('Ctrl Pts',(-18.2625044208165,-9.60004042085346,
0.));
#34205=CARTESIAN_POINT('Ctrl Pts',(-18.3130254811852,-9.66566546403259,
0.));
#34206=CARTESIAN_POINT('Ctrl Pts',(-18.3630495772677,-9.73189932619939,
0.));
#34207=CARTESIAN_POINT('Ctrl Pts',(-18.4125796444662,-9.79873019947433,
0.));
#34208=CARTESIAN_POINT('Ctrl Pts',(-18.461614050347,-9.86615372541684,0.));
#34209=CARTESIAN_POINT('Ctrl Pts',(-18.5101489409161,-9.93416923996828,
0.));
#34210=CARTESIAN_POINT('Ctrl Pts',(-18.5581807679204,-10.0027757313807,
0.));
#34211=CARTESIAN_POINT('Ctrl Pts',(-18.605709190442,-10.0719672018851,0.));
#34212=CARTESIAN_POINT('Ctrl Pts',(-18.6527367592664,-10.1417331637795,
0.));
#34213=CARTESIAN_POINT('Ctrl Pts',(-18.699267629819,-10.2120606864872,0.));
#34214=CARTESIAN_POINT('Ctrl Pts',(-18.7453065790062,-10.2829359603685,
0.));
#34215=CARTESIAN_POINT('Ctrl Pts',(-18.7908579693851,-10.3543459451258,
0.));
#34216=CARTESIAN_POINT('Ctrl Pts',(-18.8359245594214,-10.4262802670211,
0.));
#34217=CARTESIAN_POINT('Ctrl Pts',(-18.8805076729356,-10.4987309368494,
0.));
#34218=CARTESIAN_POINT('Ctrl Pts',(-18.9246077453188,-10.5716914651544,
0.));
#34219=CARTESIAN_POINT('Ctrl Pts',(-18.9682247574834,-10.6451561585969,
0.));
#34220=CARTESIAN_POINT('Ctrl Pts',(-19.0113586878152,-10.7191193896586,
0.));
#34221=CARTESIAN_POINT('Ctrl Pts',(-19.0540100416943,-10.7935747414879,
0.));
#34222=CARTESIAN_POINT('Ctrl Pts',(-19.0961797996403,-10.868515097783,0.));
#34223=CARTESIAN_POINT('Ctrl Pts',(-19.1378691901023,-10.9439330179206,
0.));
#34224=CARTESIAN_POINT('Ctrl Pts',(-19.1790795192393,-11.0198210228993,
0.));
#34225=CARTESIAN_POINT('Ctrl Pts',(-19.2198119937835,-11.0961718903994,
0.));
#34226=CARTESIAN_POINT('Ctrl Pts',(-19.2600675167206,-11.1729790050543,
0.));
#34227=CARTESIAN_POINT('Ctrl Pts',(-19.2998466936739,-11.2502363198588,
0.));
#34228=CARTESIAN_POINT('Ctrl Pts',(-19.3391499248083,-11.3279381634523,
0.));
#34229=CARTESIAN_POINT('Ctrl Pts',(-19.3779774742876,-11.4060790880015,
0.));
#34230=CARTESIAN_POINT('Ctrl Pts',(-19.4163295466324,-11.4846537135043,
0.));
#34231=CARTESIAN_POINT('Ctrl Pts',(-19.4542063779876,-11.5636565297382,
0.));
#34232=CARTESIAN_POINT('Ctrl Pts',(-19.4916082541529,-11.6430819099846,
0.));
#34233=CARTESIAN_POINT('Ctrl Pts',(-19.5285354853626,-11.722924244195,0.));
#34234=CARTESIAN_POINT('Ctrl Pts',(-19.5649883985826,-11.8031780389346,
0.));
#34235=CARTESIAN_POINT('Ctrl Pts',(-19.6009673241771,-11.8838380136222,
0.));
#34236=CARTESIAN_POINT('Ctrl Pts',(-19.6364725931695,-11.9648992312094,
0.));
#34237=CARTESIAN_POINT('Ctrl Pts',(-19.6715045149944,-12.0463570680308,
0.));
#34238=CARTESIAN_POINT('Ctrl Pts',(-19.7060633406705,-12.1282070378972,
0.));
#34239=CARTESIAN_POINT('Ctrl Pts',(-19.7401492304335,-12.2104446447874,
0.));
#34240=CARTESIAN_POINT('Ctrl Pts',(-19.7737622285562,-12.2930652417986,
0.));
#34241=CARTESIAN_POINT('Ctrl Pts',(-19.8069022248387,-12.3760638341708,
0.));
#34242=CARTESIAN_POINT('Ctrl Pts',(-19.839568972011,-12.4594350764989,0.));
#34243=CARTESIAN_POINT('Ctrl Pts',(-19.8717621942733,-12.5431736030595,
0.));
#34244=CARTESIAN_POINT('Ctrl Pts',(-19.9034816813503,-12.6272742843372,
0.));
#34245=CARTESIAN_POINT('Ctrl Pts',(-19.9347273847264,-12.7117325003719,
0.));
#34246=CARTESIAN_POINT('Ctrl Pts',(-19.9654995335894,-12.7965444294443,
0.));
#34247=CARTESIAN_POINT('Ctrl Pts',(-20.0018585267766,-12.8987398182747,
0.));
#34248=CARTESIAN_POINT('Ctrl Pts',(-20.0315673466055,-12.9843387891477,
0.));
#34249=CARTESIAN_POINT('Ctrl Pts',(-20.054957345404,-13.0530957702829,0.));
#34250=CARTESIAN_POINT('Ctrl Pts',(-20.0722879610899,-13.1048196144678,
0.));
#34251=CARTESIAN_POINT('Ctrl Pts',(-20.0837475345526,-13.1393715591102,
0.));
#34252=CARTESIAN_POINT('Ctrl Pts',(-16.8707481591095,-8.28171148831561,
15.));
#34253=CARTESIAN_POINT('Ctrl Pts',(-16.8848228151885,-8.28862062120314,
15.));
#34254=CARTESIAN_POINT('Ctrl Pts',(-16.9126979078877,-8.30290517019115,
15.));
#34255=CARTESIAN_POINT('Ctrl Pts',(-16.9536879065132,-8.32573081382562,
15.));
#34256=CARTESIAN_POINT('Ctrl Pts',(-17.0067806259695,-8.35882146841243,
15.));
#34257=CARTESIAN_POINT('Ctrl Pts',(-17.071033847921,-8.40379607744265,15.));
#34258=CARTESIAN_POINT('Ctrl Pts',(-17.1337886602855,-8.45135198307876,
15.));
#34259=CARTESIAN_POINT('Ctrl Pts',(-17.1956428575086,-8.50048099003882,
15.));
#34260=CARTESIAN_POINT('Ctrl Pts',(-17.2570167183611,-8.55046295192433,
15.));
#34261=CARTESIAN_POINT('Ctrl Pts',(-17.3180459442745,-8.60104338529165,
15.));
#34262=CARTESIAN_POINT('Ctrl Pts',(-17.3786861166843,-8.65226368112815,
15.));
#34263=CARTESIAN_POINT('Ctrl Pts',(-17.438788019753,-8.70433925112174,15.));
#34264=CARTESIAN_POINT('Ctrl Pts',(-17.4981785296199,-8.75752832625954,
15.));
#34265=CARTESIAN_POINT('Ctrl Pts',(-17.5567525798882,-8.8119830723955,15.));
#34266=CARTESIAN_POINT('Ctrl Pts',(-17.614513388992,-8.86768402115343,15.));
#34267=CARTESIAN_POINT('Ctrl Pts',(-17.6715250120654,-8.92451585185175,
15.));
#34268=CARTESIAN_POINT('Ctrl Pts',(-17.7278841963319,-8.98231202490685,
15.));
#34269=CARTESIAN_POINT('Ctrl Pts',(-17.7836872744016,-9.04090748239097,
15.));
#34270=CARTESIAN_POINT('Ctrl Pts',(-17.8389924349283,-9.10019864472208,
15.));
#34271=CARTESIAN_POINT('Ctrl Pts',(-17.8938116696237,-9.16015616361609,
15.));
#34272=CARTESIAN_POINT('Ctrl Pts',(-17.9481305624284,-9.22079331175917,
15.));
#34273=CARTESIAN_POINT('Ctrl Pts',(-18.0019206847747,-9.2821461557447,15.));
#34274=CARTESIAN_POINT('Ctrl Pts',(-18.0551538338035,-9.34425079614395,
15.));
#34275=CARTESIAN_POINT('Ctrl Pts',(-18.1078184146735,-9.40711718355464,
15.));
#34276=CARTESIAN_POINT('Ctrl Pts',(-18.1599204445014,-9.47072748065831,
15.));
#34277=CARTESIAN_POINT('Ctrl Pts',(-18.2114756946126,-9.53504856811685,
15.));
#34278=CARTESIAN_POINT('Ctrl Pts',(-18.2625044208165,-9.60004042085346,
15.));
#34279=CARTESIAN_POINT('Ctrl Pts',(-18.3130254811852,-9.66566546403259,
15.));
#34280=CARTESIAN_POINT('Ctrl Pts',(-18.3630495772677,-9.73189932619939,
15.));
#34281=CARTESIAN_POINT('Ctrl Pts',(-18.4125796444662,-9.79873019947433,
15.));
#34282=CARTESIAN_POINT('Ctrl Pts',(-18.461614050347,-9.86615372541684,15.));
#34283=CARTESIAN_POINT('Ctrl Pts',(-18.5101489409161,-9.93416923996828,
15.));
#34284=CARTESIAN_POINT('Ctrl Pts',(-18.5581807679204,-10.0027757313807,
15.));
#34285=CARTESIAN_POINT('Ctrl Pts',(-18.605709190442,-10.0719672018851,15.));
#34286=CARTESIAN_POINT('Ctrl Pts',(-18.6527367592664,-10.1417331637795,
15.));
#34287=CARTESIAN_POINT('Ctrl Pts',(-18.699267629819,-10.2120606864872,15.));
#34288=CARTESIAN_POINT('Ctrl Pts',(-18.7453065790062,-10.2829359603685,
15.));
#34289=CARTESIAN_POINT('Ctrl Pts',(-18.7908579693851,-10.3543459451258,
15.));
#34290=CARTESIAN_POINT('Ctrl Pts',(-18.8359245594214,-10.4262802670211,
15.));
#34291=CARTESIAN_POINT('Ctrl Pts',(-18.8805076729356,-10.4987309368494,
15.));
#34292=CARTESIAN_POINT('Ctrl Pts',(-18.9246077453188,-10.5716914651544,
15.));
#34293=CARTESIAN_POINT('Ctrl Pts',(-18.9682247574834,-10.6451561585969,
15.));
#34294=CARTESIAN_POINT('Ctrl Pts',(-19.0113586878152,-10.7191193896586,
15.));
#34295=CARTESIAN_POINT('Ctrl Pts',(-19.0540100416943,-10.7935747414879,
15.));
#34296=CARTESIAN_POINT('Ctrl Pts',(-19.0961797996403,-10.868515097783,15.));
#34297=CARTESIAN_POINT('Ctrl Pts',(-19.1378691901023,-10.9439330179206,
15.));
#34298=CARTESIAN_POINT('Ctrl Pts',(-19.1790795192393,-11.0198210228993,
15.));
#34299=CARTESIAN_POINT('Ctrl Pts',(-19.2198119937835,-11.0961718903994,
15.));
#34300=CARTESIAN_POINT('Ctrl Pts',(-19.2600675167206,-11.1729790050543,
15.));
#34301=CARTESIAN_POINT('Ctrl Pts',(-19.2998466936739,-11.2502363198588,
15.));
#34302=CARTESIAN_POINT('Ctrl Pts',(-19.3391499248083,-11.3279381634523,
15.));
#34303=CARTESIAN_POINT('Ctrl Pts',(-19.3779774742876,-11.4060790880015,
15.));
#34304=CARTESIAN_POINT('Ctrl Pts',(-19.4163295466324,-11.4846537135043,
15.));
#34305=CARTESIAN_POINT('Ctrl Pts',(-19.4542063779876,-11.5636565297382,
15.));
#34306=CARTESIAN_POINT('Ctrl Pts',(-19.4916082541529,-11.6430819099846,
15.));
#34307=CARTESIAN_POINT('Ctrl Pts',(-19.5285354853626,-11.722924244195,15.));
#34308=CARTESIAN_POINT('Ctrl Pts',(-19.5649883985826,-11.8031780389346,
15.));
#34309=CARTESIAN_POINT('Ctrl Pts',(-19.6009673241771,-11.8838380136222,
15.));
#34310=CARTESIAN_POINT('Ctrl Pts',(-19.6364725931695,-11.9648992312094,
15.));
#34311=CARTESIAN_POINT('Ctrl Pts',(-19.6715045149944,-12.0463570680308,
15.));
#34312=CARTESIAN_POINT('Ctrl Pts',(-19.7060633406705,-12.1282070378972,
15.));
#34313=CARTESIAN_POINT('Ctrl Pts',(-19.7401492304335,-12.2104446447874,
15.));
#34314=CARTESIAN_POINT('Ctrl Pts',(-19.7737622285562,-12.2930652417986,
15.));
#34315=CARTESIAN_POINT('Ctrl Pts',(-19.8069022248387,-12.3760638341708,
15.));
#34316=CARTESIAN_POINT('Ctrl Pts',(-19.839568972011,-12.4594350764989,15.));
#34317=CARTESIAN_POINT('Ctrl Pts',(-19.8717621942733,-12.5431736030595,
15.));
#34318=CARTESIAN_POINT('Ctrl Pts',(-19.9034816813503,-12.6272742843372,
15.));
#34319=CARTESIAN_POINT('Ctrl Pts',(-19.9347273847264,-12.7117325003719,
15.));
#34320=CARTESIAN_POINT('Ctrl Pts',(-19.9654995335894,-12.7965444294443,
15.));
#34321=CARTESIAN_POINT('Ctrl Pts',(-20.0018585267766,-12.8987398182747,
15.));
#34322=CARTESIAN_POINT('Ctrl Pts',(-20.0315673466055,-12.9843387891477,
15.));
#34323=CARTESIAN_POINT('Ctrl Pts',(-20.054957345404,-13.0530957702829,15.));
#34324=CARTESIAN_POINT('Ctrl Pts',(-20.0722879610899,-13.1048196144678,
15.));
#34325=CARTESIAN_POINT('Ctrl Pts',(-20.0837475345526,-13.1393715591102,
15.));
#34326=CARTESIAN_POINT('Ctrl Pts',(-23.9712218930251,-1.17495572484831,
0.));
#34327=CARTESIAN_POINT('Ctrl Pts',(-23.9712218930251,-1.17495572484831,
18.));
#34328=CARTESIAN_POINT('Ctrl Pts',(-23.9564318364582,-1.18556439589231,
0.));
#34329=CARTESIAN_POINT('Ctrl Pts',(-23.9564318364582,-1.18556439589231,
18.));
#34330=CARTESIAN_POINT('Ctrl Pts',(-23.9268340213745,-1.20672599652272,
0.));
#34331=CARTESIAN_POINT('Ctrl Pts',(-23.9268340213745,-1.20672599652272,
18.));
#34332=CARTESIAN_POINT('Ctrl Pts',(-23.8823841929226,-1.2383011730893,0.));
#34333=CARTESIAN_POINT('Ctrl Pts',(-23.8823841929226,-1.2383011730893,18.));
#34334=CARTESIAN_POINT('Ctrl Pts',(-23.8230115078373,-1.28006684869166,
0.));
#34335=CARTESIAN_POINT('Ctrl Pts',(-23.8230115078373,-1.28006684869166,
18.));
#34336=CARTESIAN_POINT('Ctrl Pts',(-23.748618507953,-1.33171549586249,0.));
#34337=CARTESIAN_POINT('Ctrl Pts',(-23.748618507953,-1.33171549586249,18.));
#34338=CARTESIAN_POINT('Ctrl Pts',(-23.6740485197917,-1.38280426780156,
0.));
#34339=CARTESIAN_POINT('Ctrl Pts',(-23.6740485197917,-1.38280426780156,
18.));
#34340=CARTESIAN_POINT('Ctrl Pts',(-23.5993021272808,-1.43333114446389,
0.));
#34341=CARTESIAN_POINT('Ctrl Pts',(-23.5993021272808,-1.43333114446389,
18.));
#34342=CARTESIAN_POINT('Ctrl Pts',(-23.5243805284282,-1.4832935129085,0.));
#34343=CARTESIAN_POINT('Ctrl Pts',(-23.5243805284282,-1.4832935129085,18.));
#34344=CARTESIAN_POINT('Ctrl Pts',(-23.4492857841673,-1.53268814658653,
0.));
#34345=CARTESIAN_POINT('Ctrl Pts',(-23.4492857841673,-1.53268814658653,
18.));
#34346=CARTESIAN_POINT('Ctrl Pts',(-23.3740206492924,-1.58151133638847,
0.));
#34347=CARTESIAN_POINT('Ctrl Pts',(-23.3740206492924,-1.58151133638847,
18.));
#34348=CARTESIAN_POINT('Ctrl Pts',(-23.2985883089733,-1.62975905604583,
0.));
#34349=CARTESIAN_POINT('Ctrl Pts',(-23.2985883089733,-1.62975905604583,
18.));
#34350=CARTESIAN_POINT('Ctrl Pts',(-23.2229921402299,-1.67742712670823,
0.));
#34351=CARTESIAN_POINT('Ctrl Pts',(-23.2229921402299,-1.67742712670823,
18.));
#34352=CARTESIAN_POINT('Ctrl Pts',(-23.1472354850579,-1.72451136919382,
0.));
#34353=CARTESIAN_POINT('Ctrl Pts',(-23.1472354850579,-1.72451136919382,
18.));
#34354=CARTESIAN_POINT('Ctrl Pts',(-23.0713213684573,-1.77100780743078,
0.));
#34355=CARTESIAN_POINT('Ctrl Pts',(-23.0713213684573,-1.77100780743078,
18.));
#34356=CARTESIAN_POINT('Ctrl Pts',(-22.9952524859917,-1.81691265597281,
0.));
#34357=CARTESIAN_POINT('Ctrl Pts',(-22.9952524859917,-1.81691265597281,
18.));
#34358=CARTESIAN_POINT('Ctrl Pts',(-22.9190313507225,-1.86222218327818,
0.));
#34359=CARTESIAN_POINT('Ctrl Pts',(-22.9190313507225,-1.86222218327818,
18.));
#34360=CARTESIAN_POINT('Ctrl Pts',(-22.8426603964871,-1.90693261239855,
0.));
#34361=CARTESIAN_POINT('Ctrl Pts',(-22.8426603964871,-1.90693261239855,
18.));
#34362=CARTESIAN_POINT('Ctrl Pts',(-22.7661420906702,-1.9510400208289,0.));
#34363=CARTESIAN_POINT('Ctrl Pts',(-22.7661420906702,-1.9510400208289,18.));
#34364=CARTESIAN_POINT('Ctrl Pts',(-22.6894790673923,-1.99454021984253,
0.));
#34365=CARTESIAN_POINT('Ctrl Pts',(-22.6894790673923,-1.99454021984253,
18.));
#34366=CARTESIAN_POINT('Ctrl Pts',(-22.6126741632309,-2.03742874317627,
0.));
#34367=CARTESIAN_POINT('Ctrl Pts',(-22.6126741632309,-2.03742874317627,
18.));
#34368=CARTESIAN_POINT('Ctrl Pts',(-22.5357303426251,-2.07970095436223,
0.));
#34369=CARTESIAN_POINT('Ctrl Pts',(-22.5357303426251,-2.07970095436223,
18.));
#34370=CARTESIAN_POINT('Ctrl Pts',(-22.4586506520939,-2.1213521324248,0.));
#34371=CARTESIAN_POINT('Ctrl Pts',(-22.4586506520939,-2.1213521324248,18.));
#34372=CARTESIAN_POINT('Ctrl Pts',(-22.3814381677224,-2.16237755726403,
0.));
#34373=CARTESIAN_POINT('Ctrl Pts',(-22.3814381677224,-2.16237755726403,
18.));
#34374=CARTESIAN_POINT('Ctrl Pts',(-22.3040959372933,-2.20277263221399,
0.));
#34375=CARTESIAN_POINT('Ctrl Pts',(-22.3040959372933,-2.20277263221399,
18.));
#34376=CARTESIAN_POINT('Ctrl Pts',(-22.2266269576315,-2.24253288454712,
0.));
#34377=CARTESIAN_POINT('Ctrl Pts',(-22.2266269576315,-2.24253288454712,
18.));
#34378=CARTESIAN_POINT('Ctrl Pts',(-22.1490342171802,-2.2816537516023,0.));
#34379=CARTESIAN_POINT('Ctrl Pts',(-22.1490342171802,-2.2816537516023,18.));
#34380=CARTESIAN_POINT('Ctrl Pts',(-22.0713207257413,-2.32013040994124,
0.));
#34381=CARTESIAN_POINT('Ctrl Pts',(-22.0713207257413,-2.32013040994124,
18.));
#34382=CARTESIAN_POINT('Ctrl Pts',(-21.9934895476958,-2.35795761145761,
0.));
#34383=CARTESIAN_POINT('Ctrl Pts',(-21.9934895476958,-2.35795761145761,
18.));
#34384=CARTESIAN_POINT('Ctrl Pts',(-21.9155438409279,-2.39512947344577,
0.));
#34385=CARTESIAN_POINT('Ctrl Pts',(-21.9155438409279,-2.39512947344577,
18.));
#34386=CARTESIAN_POINT('Ctrl Pts',(-21.8374868743435,-2.43163944362692,
0.));
#34387=CARTESIAN_POINT('Ctrl Pts',(-21.8374868743435,-2.43163944362692,
18.));
#34388=CARTESIAN_POINT('Ctrl Pts',(-21.7593219872847,-2.46748070362075,
0.));
#34389=CARTESIAN_POINT('Ctrl Pts',(-21.7593219872847,-2.46748070362075,
18.));
#34390=CARTESIAN_POINT('Ctrl Pts',(-21.6810525594039,-2.50264651177234,
0.));
#34391=CARTESIAN_POINT('Ctrl Pts',(-21.6810525594039,-2.50264651177234,
18.));
#34392=CARTESIAN_POINT('Ctrl Pts',(-21.6026819803014,-2.53713053453766,
0.));
#34393=CARTESIAN_POINT('Ctrl Pts',(-21.6026819803014,-2.53713053453766,
18.));
#34394=CARTESIAN_POINT('Ctrl Pts',(-21.5242136128466,-2.5709272835198,0.));
#34395=CARTESIAN_POINT('Ctrl Pts',(-21.5242136128466,-2.5709272835198,18.));
#34396=CARTESIAN_POINT('Ctrl Pts',(-21.4456507822983,-2.60403221866523,
0.));
#34397=CARTESIAN_POINT('Ctrl Pts',(-21.4456507822983,-2.60403221866523,
18.));
#34398=CARTESIAN_POINT('Ctrl Pts',(-21.3669968505594,-2.6364407451853,0.));
#34399=CARTESIAN_POINT('Ctrl Pts',(-21.3669968505594,-2.6364407451853,18.));
#34400=CARTESIAN_POINT('Ctrl Pts',(-21.2882552797978,-2.668147357083,0.));
#34401=CARTESIAN_POINT('Ctrl Pts',(-21.2882552797978,-2.668147357083,18.));
#34402=CARTESIAN_POINT('Ctrl Pts',(-21.2094296949571,-2.69914481283353,
0.));
#34403=CARTESIAN_POINT('Ctrl Pts',(-21.2094296949571,-2.69914481283353,
18.));
#34404=CARTESIAN_POINT('Ctrl Pts',(-21.1305239619219,-2.72942309852119,
0.));
#34405=CARTESIAN_POINT('Ctrl Pts',(-21.1305239619219,-2.72942309852119,
18.));
#34406=CARTESIAN_POINT('Ctrl Pts',(-21.0515422162039,-2.75896910007689,
0.));
#34407=CARTESIAN_POINT('Ctrl Pts',(-21.0515422162039,-2.75896910007689,
18.));
#34408=CARTESIAN_POINT('Ctrl Pts',(-20.9724887103073,-2.78776883747221,
0.));
#34409=CARTESIAN_POINT('Ctrl Pts',(-20.9724887103073,-2.78776883747221,
18.));
#34410=CARTESIAN_POINT('Ctrl Pts',(-20.8933676828246,-2.81580940715317,
0.));
#34411=CARTESIAN_POINT('Ctrl Pts',(-20.8933676828246,-2.81580940715317,
18.));
#34412=CARTESIAN_POINT('Ctrl Pts',(-20.8141832346435,-2.84308082507643,
0.));
#34413=CARTESIAN_POINT('Ctrl Pts',(-20.8141832346435,-2.84308082507643,
18.));
#34414=CARTESIAN_POINT('Ctrl Pts',(-20.7349391669725,-2.86957843933153,
0.));
#34415=CARTESIAN_POINT('Ctrl Pts',(-20.7349391669725,-2.86957843933153,
18.));
#34416=CARTESIAN_POINT('Ctrl Pts',(-20.6556389450993,-2.89530351700805,
0.));
#34417=CARTESIAN_POINT('Ctrl Pts',(-20.6556389450993,-2.89530351700805,
18.));
#34418=CARTESIAN_POINT('Ctrl Pts',(-20.5762860772943,-2.92025778619206,
0.));
#34419=CARTESIAN_POINT('Ctrl Pts',(-20.5762860772943,-2.92025778619206,
18.));
#34420=CARTESIAN_POINT('Ctrl Pts',(-20.4968844460513,-2.94443868035154,
0.));
#34421=CARTESIAN_POINT('Ctrl Pts',(-20.4968844460513,-2.94443868035154,
18.));
#34422=CARTESIAN_POINT('Ctrl Pts',(-20.4174386170774,-2.96783492132513,
0.));
#34423=CARTESIAN_POINT('Ctrl Pts',(-20.4174386170774,-2.96783492132513,
18.));
#34424=CARTESIAN_POINT('Ctrl Pts',(-20.3379542578194,-2.99042050197904,
0.));
#34425=CARTESIAN_POINT('Ctrl Pts',(-20.3379542578194,-2.99042050197904,
18.));
#34426=CARTESIAN_POINT('Ctrl Pts',(-20.2584381977107,-3.01215393913612,
0.));
#34427=CARTESIAN_POINT('Ctrl Pts',(-20.2584381977107,-3.01215393913612,
18.));
#34428=CARTESIAN_POINT('Ctrl Pts',(-20.178897575607,-3.03299094576288,0.));
#34429=CARTESIAN_POINT('Ctrl Pts',(-20.178897575607,-3.03299094576288,18.));
#34430=CARTESIAN_POINT('Ctrl Pts',(-20.0993390992966,-3.0528954575995,0.));
#34431=CARTESIAN_POINT('Ctrl Pts',(-20.0993390992966,-3.0528954575995,18.));
#34432=CARTESIAN_POINT('Ctrl Pts',(-20.0197683853426,-3.07184950717982,
0.));
#34433=CARTESIAN_POINT('Ctrl Pts',(-20.0197683853426,-3.07184950717982,
18.));
#34434=CARTESIAN_POINT('Ctrl Pts',(-19.9401889653541,-3.08986795998319,
0.));
#34435=CARTESIAN_POINT('Ctrl Pts',(-19.9401889653541,-3.08986795998319,
18.));
#34436=CARTESIAN_POINT('Ctrl Pts',(-19.8606024365399,-3.10699659920993,
0.));
#34437=CARTESIAN_POINT('Ctrl Pts',(-19.8606024365399,-3.10699659920993,
18.));
#34438=CARTESIAN_POINT('Ctrl Pts',(-19.7810105986827,-3.12328131323979,
0.));
#34439=CARTESIAN_POINT('Ctrl Pts',(-19.7810105986827,-3.12328131323979,
18.));
#34440=CARTESIAN_POINT('Ctrl Pts',(-19.7014173131304,-3.13874131344865,
0.));
#34441=CARTESIAN_POINT('Ctrl Pts',(-19.7014173131304,-3.13874131344865,
18.));
#34442=CARTESIAN_POINT('Ctrl Pts',(-19.6218301288731,-3.15334580802458,
0.));
#34443=CARTESIAN_POINT('Ctrl Pts',(-19.6218301288731,-3.15334580802458,
18.));
#34444=CARTESIAN_POINT('Ctrl Pts',(-19.5422628528517,-3.16697679689294,
0.));
#34445=CARTESIAN_POINT('Ctrl Pts',(-19.5422628528517,-3.16697679689294,
18.));
#34446=CARTESIAN_POINT('Ctrl Pts',(-19.4627345689632,-3.17944412249753,
0.));
#34447=CARTESIAN_POINT('Ctrl Pts',(-19.4627345689632,-3.17944412249753,
18.));
#34448=CARTESIAN_POINT('Ctrl Pts',(-19.3832648965708,-3.19055618489382,
0.));
#34449=CARTESIAN_POINT('Ctrl Pts',(-19.3832648965708,-3.19055618489382,
18.));
#34450=CARTESIAN_POINT('Ctrl Pts',(-19.3038697977783,-3.20018203702739,
0.));
#34451=CARTESIAN_POINT('Ctrl Pts',(-19.3038697977783,-3.20018203702739,
18.));
#34452=CARTESIAN_POINT('Ctrl Pts',(-19.2245581120423,-3.2083040369031,0.));
#34453=CARTESIAN_POINT('Ctrl Pts',(-19.2245581120423,-3.2083040369031,18.));
#34454=CARTESIAN_POINT('Ctrl Pts',(-19.1453253990185,-3.21510704576116,
0.));
#34455=CARTESIAN_POINT('Ctrl Pts',(-19.1453253990185,-3.21510704576116,
18.));
#34456=CARTESIAN_POINT('Ctrl Pts',(-19.0661599344864,-3.22090173651084,
0.));
#34457=CARTESIAN_POINT('Ctrl Pts',(-19.0661599344864,-3.22090173651084,
18.));
#34458=CARTESIAN_POINT('Ctrl Pts',(-18.987055820781,-3.22595008773714,0.));
#34459=CARTESIAN_POINT('Ctrl Pts',(-18.987055820781,-3.22595008773714,18.));
#34460=CARTESIAN_POINT('Ctrl Pts',(-18.908024664264,-3.23031169402938,0.));
#34461=CARTESIAN_POINT('Ctrl Pts',(-18.908024664264,-3.23031169402938,18.));
#34462=CARTESIAN_POINT('Ctrl Pts',(-18.8291062617862,-3.23370091065669,
0.));
#34463=CARTESIAN_POINT('Ctrl Pts',(-18.8291062617862,-3.23370091065669,
18.));
#34464=CARTESIAN_POINT('Ctrl Pts',(-18.7503838921122,-3.23528809328096,
0.));
#34465=CARTESIAN_POINT('Ctrl Pts',(-18.7503838921122,-3.23528809328096,
18.));
#34466=CARTESIAN_POINT('Ctrl Pts',(-18.6719665316945,-3.23390622002644,
0.));
#34467=CARTESIAN_POINT('Ctrl Pts',(-18.6719665316945,-3.23390622002644,
18.));
#34468=CARTESIAN_POINT('Ctrl Pts',(-18.6095634206219,-3.2294700044416,0.));
#34469=CARTESIAN_POINT('Ctrl Pts',(-18.6095634206219,-3.2294700044416,18.));
#34470=CARTESIAN_POINT('Ctrl Pts',(-18.5629852384321,-3.22384302136591,
0.));
#34471=CARTESIAN_POINT('Ctrl Pts',(-18.5629852384321,-3.22384302136591,
18.));
#34472=CARTESIAN_POINT('Ctrl Pts',(-18.5320375674878,-3.2190148958593,0.));
#34473=CARTESIAN_POINT('Ctrl Pts',(-18.5320375674878,-3.2190148958593,18.));
#34474=CARTESIAN_POINT('Ctrl Pts',(-18.5165898451125,-3.21633162650739,
0.));
#34475=CARTESIAN_POINT('Ctrl Pts',(-18.5165898451125,-3.21633162650739,
18.));
#34476=CARTESIAN_POINT('',(-23.9712218930251,-1.17495572484826,0.));
#34477=CARTESIAN_POINT('Ctrl Pts',(-18.5165898451125,-3.21633162650739,
0.));
#34478=CARTESIAN_POINT('Ctrl Pts',(-18.5320375674878,-3.2190148958593,0.));
#34479=CARTESIAN_POINT('Ctrl Pts',(-18.5629852384321,-3.22384302136591,
0.));
#34480=CARTESIAN_POINT('Ctrl Pts',(-18.6095634206219,-3.2294700044416,0.));
#34481=CARTESIAN_POINT('Ctrl Pts',(-18.6719665316945,-3.23390622002644,
0.));
#34482=CARTESIAN_POINT('Ctrl Pts',(-18.7503838921122,-3.23528809328096,
0.));
#34483=CARTESIAN_POINT('Ctrl Pts',(-18.8291062617862,-3.23370091065669,
0.));
#34484=CARTESIAN_POINT('Ctrl Pts',(-18.908024664264,-3.23031169402938,0.));
#34485=CARTESIAN_POINT('Ctrl Pts',(-18.987055820781,-3.22595008773714,0.));
#34486=CARTESIAN_POINT('Ctrl Pts',(-19.0661599344864,-3.22090173651084,
0.));
#34487=CARTESIAN_POINT('Ctrl Pts',(-19.1453253990185,-3.21510704576116,
0.));
#34488=CARTESIAN_POINT('Ctrl Pts',(-19.2245581120423,-3.2083040369031,0.));
#34489=CARTESIAN_POINT('Ctrl Pts',(-19.3038697977783,-3.20018203702739,
0.));
#34490=CARTESIAN_POINT('Ctrl Pts',(-19.3832648965708,-3.19055618489382,
0.));
#34491=CARTESIAN_POINT('Ctrl Pts',(-19.4627345689632,-3.17944412249753,
0.));
#34492=CARTESIAN_POINT('Ctrl Pts',(-19.5422628528517,-3.16697679689294,
0.));
#34493=CARTESIAN_POINT('Ctrl Pts',(-19.6218301288731,-3.15334580802458,
0.));
#34494=CARTESIAN_POINT('Ctrl Pts',(-19.7014173131304,-3.13874131344865,
0.));
#34495=CARTESIAN_POINT('Ctrl Pts',(-19.7810105986827,-3.12328131323979,
0.));
#34496=CARTESIAN_POINT('Ctrl Pts',(-19.8606024365399,-3.10699659920993,
0.));
#34497=CARTESIAN_POINT('Ctrl Pts',(-19.9401889653541,-3.08986795998319,
0.));
#34498=CARTESIAN_POINT('Ctrl Pts',(-20.0197683853426,-3.07184950717982,
0.));
#34499=CARTESIAN_POINT('Ctrl Pts',(-20.0993390992966,-3.0528954575995,0.));
#34500=CARTESIAN_POINT('Ctrl Pts',(-20.178897575607,-3.03299094576288,0.));
#34501=CARTESIAN_POINT('Ctrl Pts',(-20.2584381977107,-3.01215393913612,
0.));
#34502=CARTESIAN_POINT('Ctrl Pts',(-20.3379542578194,-2.99042050197904,
0.));
#34503=CARTESIAN_POINT('Ctrl Pts',(-20.4174386170774,-2.96783492132513,
0.));
#34504=CARTESIAN_POINT('Ctrl Pts',(-20.4968844460513,-2.94443868035154,
0.));
#34505=CARTESIAN_POINT('Ctrl Pts',(-20.5762860772943,-2.92025778619206,
0.));
#34506=CARTESIAN_POINT('Ctrl Pts',(-20.6556389450993,-2.89530351700805,
0.));
#34507=CARTESIAN_POINT('Ctrl Pts',(-20.7349391669725,-2.86957843933153,
0.));
#34508=CARTESIAN_POINT('Ctrl Pts',(-20.8141832346435,-2.84308082507643,
0.));
#34509=CARTESIAN_POINT('Ctrl Pts',(-20.8933676828246,-2.81580940715317,
0.));
#34510=CARTESIAN_POINT('Ctrl Pts',(-20.9724887103073,-2.78776883747221,
0.));
#34511=CARTESIAN_POINT('Ctrl Pts',(-21.0515422162039,-2.75896910007689,
0.));
#34512=CARTESIAN_POINT('Ctrl Pts',(-21.1305239619219,-2.72942309852119,
0.));
#34513=CARTESIAN_POINT('Ctrl Pts',(-21.2094296949571,-2.69914481283353,
0.));
#34514=CARTESIAN_POINT('Ctrl Pts',(-21.2882552797978,-2.668147357083,0.));
#34515=CARTESIAN_POINT('Ctrl Pts',(-21.3669968505594,-2.6364407451853,0.));
#34516=CARTESIAN_POINT('Ctrl Pts',(-21.4456507822983,-2.60403221866523,
0.));
#34517=CARTESIAN_POINT('Ctrl Pts',(-21.5242136128466,-2.5709272835198,0.));
#34518=CARTESIAN_POINT('Ctrl Pts',(-21.6026819803014,-2.53713053453766,
0.));
#34519=CARTESIAN_POINT('Ctrl Pts',(-21.6810525594039,-2.50264651177234,
0.));
#34520=CARTESIAN_POINT('Ctrl Pts',(-21.7593219872847,-2.46748070362075,
0.));
#34521=CARTESIAN_POINT('Ctrl Pts',(-21.8374868743435,-2.43163944362692,
0.));
#34522=CARTESIAN_POINT('Ctrl Pts',(-21.9155438409279,-2.39512947344577,
0.));
#34523=CARTESIAN_POINT('Ctrl Pts',(-21.9934895476958,-2.35795761145761,
0.));
#34524=CARTESIAN_POINT('Ctrl Pts',(-22.0713207257413,-2.32013040994124,
0.));
#34525=CARTESIAN_POINT('Ctrl Pts',(-22.1490342171802,-2.2816537516023,0.));
#34526=CARTESIAN_POINT('Ctrl Pts',(-22.2266269576315,-2.24253288454712,
0.));
#34527=CARTESIAN_POINT('Ctrl Pts',(-22.3040959372933,-2.20277263221399,
0.));
#34528=CARTESIAN_POINT('Ctrl Pts',(-22.3814381677224,-2.16237755726403,
0.));
#34529=CARTESIAN_POINT('Ctrl Pts',(-22.4586506520939,-2.1213521324248,0.));
#34530=CARTESIAN_POINT('Ctrl Pts',(-22.5357303426251,-2.07970095436223,
0.));
#34531=CARTESIAN_POINT('Ctrl Pts',(-22.6126741632309,-2.03742874317627,
0.));
#34532=CARTESIAN_POINT('Ctrl Pts',(-22.6894790673923,-1.99454021984253,
0.));
#34533=CARTESIAN_POINT('Ctrl Pts',(-22.7661420906702,-1.9510400208289,0.));
#34534=CARTESIAN_POINT('Ctrl Pts',(-22.8426603964871,-1.90693261239855,
0.));
#34535=CARTESIAN_POINT('Ctrl Pts',(-22.9190313507225,-1.86222218327818,
0.));
#34536=CARTESIAN_POINT('Ctrl Pts',(-22.9952524859917,-1.81691265597281,
0.));
#34537=CARTESIAN_POINT('Ctrl Pts',(-23.0713213684573,-1.77100780743078,
0.));
#34538=CARTESIAN_POINT('Ctrl Pts',(-23.1472354850579,-1.72451136919382,
0.));
#34539=CARTESIAN_POINT('Ctrl Pts',(-23.2229921402299,-1.67742712670823,
0.));
#34540=CARTESIAN_POINT('Ctrl Pts',(-23.2985883089733,-1.62975905604583,
0.));
#34541=CARTESIAN_POINT('Ctrl Pts',(-23.3740206492924,-1.58151133638847,
0.));
#34542=CARTESIAN_POINT('Ctrl Pts',(-23.4492857841673,-1.53268814658653,
0.));
#34543=CARTESIAN_POINT('Ctrl Pts',(-23.5243805284282,-1.4832935129085,0.));
#34544=CARTESIAN_POINT('Ctrl Pts',(-23.5993021272808,-1.43333114446389,
0.));
#34545=CARTESIAN_POINT('Ctrl Pts',(-23.6740485197917,-1.38280426780156,
0.));
#34546=CARTESIAN_POINT('Ctrl Pts',(-23.7635325055853,-1.32149774147467,
0.));
#34547=CARTESIAN_POINT('Ctrl Pts',(-23.8378812584003,-1.2697091254959,0.));
#34548=CARTESIAN_POINT('Ctrl Pts',(-23.89721850443,-1.22783185562043,0.));
#34549=CARTESIAN_POINT('Ctrl Pts',(-23.9416417798467,-1.19617306697386,
0.));
#34550=CARTESIAN_POINT('Ctrl Pts',(-23.9712218930251,-1.17495572484831,
0.));
#34551=CARTESIAN_POINT('',(-23.9712218930251,-1.17495572484826,15.));
#34552=CARTESIAN_POINT('Ctrl Pts',(-23.9712218930251,-1.17495572484831,
15.));
#34553=CARTESIAN_POINT('Ctrl Pts',(-23.9564318364582,-1.18556439589231,
15.));
#34554=CARTESIAN_POINT('Ctrl Pts',(-23.9268340213745,-1.20672599652272,
15.));
#34555=CARTESIAN_POINT('Ctrl Pts',(-23.8823841929226,-1.2383011730893,15.));
#34556=CARTESIAN_POINT('Ctrl Pts',(-23.8230115078373,-1.28006684869166,
15.));
#34557=CARTESIAN_POINT('Ctrl Pts',(-23.748618507953,-1.33171549586249,15.));
#34558=CARTESIAN_POINT('Ctrl Pts',(-23.6740485197917,-1.38280426780156,
15.));
#34559=CARTESIAN_POINT('Ctrl Pts',(-23.5993021272808,-1.43333114446389,
15.));
#34560=CARTESIAN_POINT('Ctrl Pts',(-23.5243805284282,-1.4832935129085,15.));
#34561=CARTESIAN_POINT('Ctrl Pts',(-23.4492857841673,-1.53268814658653,
15.));
#34562=CARTESIAN_POINT('Ctrl Pts',(-23.3740206492924,-1.58151133638847,
15.));
#34563=CARTESIAN_POINT('Ctrl Pts',(-23.2985883089733,-1.62975905604583,
15.));
#34564=CARTESIAN_POINT('Ctrl Pts',(-23.2229921402299,-1.67742712670823,
15.));
#34565=CARTESIAN_POINT('Ctrl Pts',(-23.1472354850579,-1.72451136919382,
15.));
#34566=CARTESIAN_POINT('Ctrl Pts',(-23.0713213684573,-1.77100780743078,
15.));
#34567=CARTESIAN_POINT('Ctrl Pts',(-22.9952524859917,-1.81691265597281,
15.));
#34568=CARTESIAN_POINT('Ctrl Pts',(-22.9190313507225,-1.86222218327818,
15.));
#34569=CARTESIAN_POINT('Ctrl Pts',(-22.8426603964871,-1.90693261239855,
15.));
#34570=CARTESIAN_POINT('Ctrl Pts',(-22.7661420906702,-1.9510400208289,15.));
#34571=CARTESIAN_POINT('Ctrl Pts',(-22.6894790673923,-1.99454021984253,
15.));
#34572=CARTESIAN_POINT('Ctrl Pts',(-22.6126741632309,-2.03742874317627,
15.));
#34573=CARTESIAN_POINT('Ctrl Pts',(-22.5357303426251,-2.07970095436223,
15.));
#34574=CARTESIAN_POINT('Ctrl Pts',(-22.4586506520939,-2.1213521324248,15.));
#34575=CARTESIAN_POINT('Ctrl Pts',(-22.3814381677224,-2.16237755726403,
15.));
#34576=CARTESIAN_POINT('Ctrl Pts',(-22.3040959372933,-2.20277263221399,
15.));
#34577=CARTESIAN_POINT('Ctrl Pts',(-22.2266269576315,-2.24253288454712,
15.));
#34578=CARTESIAN_POINT('Ctrl Pts',(-22.1490342171802,-2.2816537516023,15.));
#34579=CARTESIAN_POINT('Ctrl Pts',(-22.0713207257413,-2.32013040994124,
15.));
#34580=CARTESIAN_POINT('Ctrl Pts',(-21.9934895476958,-2.35795761145761,
15.));
#34581=CARTESIAN_POINT('Ctrl Pts',(-21.9155438409279,-2.39512947344577,
15.));
#34582=CARTESIAN_POINT('Ctrl Pts',(-21.8374868743435,-2.43163944362692,
15.));
#34583=CARTESIAN_POINT('Ctrl Pts',(-21.7593219872847,-2.46748070362075,
15.));
#34584=CARTESIAN_POINT('Ctrl Pts',(-21.6810525594039,-2.50264651177234,
15.));
#34585=CARTESIAN_POINT('Ctrl Pts',(-21.6026819803014,-2.53713053453766,
15.));
#34586=CARTESIAN_POINT('Ctrl Pts',(-21.5242136128466,-2.5709272835198,15.));
#34587=CARTESIAN_POINT('Ctrl Pts',(-21.4456507822983,-2.60403221866523,
15.));
#34588=CARTESIAN_POINT('Ctrl Pts',(-21.3669968505594,-2.6364407451853,15.));
#34589=CARTESIAN_POINT('Ctrl Pts',(-21.2882552797978,-2.668147357083,15.));
#34590=CARTESIAN_POINT('Ctrl Pts',(-21.2094296949571,-2.69914481283353,
15.));
#34591=CARTESIAN_POINT('Ctrl Pts',(-21.1305239619219,-2.72942309852119,
15.));
#34592=CARTESIAN_POINT('Ctrl Pts',(-21.0515422162039,-2.75896910007689,
15.));
#34593=CARTESIAN_POINT('Ctrl Pts',(-20.9724887103073,-2.78776883747221,
15.));
#34594=CARTESIAN_POINT('Ctrl Pts',(-20.8933676828246,-2.81580940715317,
15.));
#34595=CARTESIAN_POINT('Ctrl Pts',(-20.8141832346435,-2.84308082507643,
15.));
#34596=CARTESIAN_POINT('Ctrl Pts',(-20.7349391669725,-2.86957843933153,
15.));
#34597=CARTESIAN_POINT('Ctrl Pts',(-20.6556389450993,-2.89530351700805,
15.));
#34598=CARTESIAN_POINT('Ctrl Pts',(-20.5762860772943,-2.92025778619206,
15.));
#34599=CARTESIAN_POINT('Ctrl Pts',(-20.4968844460513,-2.94443868035154,
15.));
#34600=CARTESIAN_POINT('Ctrl Pts',(-20.4174386170774,-2.96783492132513,
15.));
#34601=CARTESIAN_POINT('Ctrl Pts',(-20.3379542578194,-2.99042050197904,
15.));
#34602=CARTESIAN_POINT('Ctrl Pts',(-20.2584381977107,-3.01215393913612,
15.));
#34603=CARTESIAN_POINT('Ctrl Pts',(-20.178897575607,-3.03299094576288,15.));
#34604=CARTESIAN_POINT('Ctrl Pts',(-20.0993390992966,-3.0528954575995,15.));
#34605=CARTESIAN_POINT('Ctrl Pts',(-20.0197683853426,-3.07184950717982,
15.));
#34606=CARTESIAN_POINT('Ctrl Pts',(-19.9401889653541,-3.08986795998319,
15.));
#34607=CARTESIAN_POINT('Ctrl Pts',(-19.8606024365399,-3.10699659920993,
15.));
#34608=CARTESIAN_POINT('Ctrl Pts',(-19.7810105986827,-3.12328131323979,
15.));
#34609=CARTESIAN_POINT('Ctrl Pts',(-19.7014173131304,-3.13874131344865,
15.));
#34610=CARTESIAN_POINT('Ctrl Pts',(-19.6218301288731,-3.15334580802458,
15.));
#34611=CARTESIAN_POINT('Ctrl Pts',(-19.5422628528517,-3.16697679689294,
15.));
#34612=CARTESIAN_POINT('Ctrl Pts',(-19.4627345689632,-3.17944412249753,
15.));
#34613=CARTESIAN_POINT('Ctrl Pts',(-19.3832648965708,-3.19055618489382,
15.));
#34614=CARTESIAN_POINT('Ctrl Pts',(-19.3038697977783,-3.20018203702739,
15.));
#34615=CARTESIAN_POINT('Ctrl Pts',(-19.2245581120423,-3.2083040369031,15.));
#34616=CARTESIAN_POINT('Ctrl Pts',(-19.1453253990185,-3.21510704576116,
15.));
#34617=CARTESIAN_POINT('Ctrl Pts',(-19.0661599344864,-3.22090173651084,
15.));
#34618=CARTESIAN_POINT('Ctrl Pts',(-18.987055820781,-3.22595008773714,15.));
#34619=CARTESIAN_POINT('Ctrl Pts',(-18.908024664264,-3.23031169402938,15.));
#34620=CARTESIAN_POINT('Ctrl Pts',(-18.8291062617862,-3.23370091065669,
15.));
#34621=CARTESIAN_POINT('Ctrl Pts',(-18.7503838921122,-3.23528809328096,
15.));
#34622=CARTESIAN_POINT('Ctrl Pts',(-18.6719665316945,-3.23390622002644,
15.));
#34623=CARTESIAN_POINT('Ctrl Pts',(-18.6095634206219,-3.2294700044416,15.));
#34624=CARTESIAN_POINT('Ctrl Pts',(-18.5629852384321,-3.22384302136591,
15.));
#34625=CARTESIAN_POINT('Ctrl Pts',(-18.5320375674878,-3.2190148958593,15.));
#34626=CARTESIAN_POINT('Ctrl Pts',(-18.5165898451125,-3.21633162650739,
15.));
#34627=CARTESIAN_POINT('',(-23.9712218930251,-1.17495572484826,0.));
#34628=CARTESIAN_POINT('Origin',(-1.15463194561016E-13,6.93889390390802E-17,
0.));
#34629=CARTESIAN_POINT('',(-23.9712218930251,1.17495572484832,0.));
#34630=CARTESIAN_POINT('Origin',(-1.15463194561016E-13,6.93889390390802E-17,
0.));
#34631=CARTESIAN_POINT('',(-23.9712218930251,1.17495572484832,15.));
#34632=CARTESIAN_POINT('Origin',(-1.15463194561016E-13,6.93889390390802E-17,
15.));
#34633=CARTESIAN_POINT('',(-23.9712218930251,1.17495572484832,0.));
#34634=CARTESIAN_POINT('Ctrl Pts',(-18.5165898451125,3.2163316265074,0.));
#34635=CARTESIAN_POINT('Ctrl Pts',(-18.5165898451125,3.2163316265074,18.));
#34636=CARTESIAN_POINT('Ctrl Pts',(-18.5320375674878,3.21901489585931,0.));
#34637=CARTESIAN_POINT('Ctrl Pts',(-18.5320375674878,3.21901489585931,18.));
#34638=CARTESIAN_POINT('Ctrl Pts',(-18.5629852384321,3.22384302136592,0.));
#34639=CARTESIAN_POINT('Ctrl Pts',(-18.5629852384321,3.22384302136592,18.));
#34640=CARTESIAN_POINT('Ctrl Pts',(-18.6095634206219,3.22947000444161,0.));
#34641=CARTESIAN_POINT('Ctrl Pts',(-18.6095634206219,3.22947000444161,18.));
#34642=CARTESIAN_POINT('Ctrl Pts',(-18.6719665316945,3.23390622002644,0.));
#34643=CARTESIAN_POINT('Ctrl Pts',(-18.6719665316945,3.23390622002644,18.));
#34644=CARTESIAN_POINT('Ctrl Pts',(-18.7503838921122,3.23528809328097,0.));
#34645=CARTESIAN_POINT('Ctrl Pts',(-18.7503838921122,3.23528809328097,18.));
#34646=CARTESIAN_POINT('Ctrl Pts',(-18.8291062617862,3.2337009106567,0.));
#34647=CARTESIAN_POINT('Ctrl Pts',(-18.8291062617862,3.2337009106567,18.));
#34648=CARTESIAN_POINT('Ctrl Pts',(-18.908024664264,3.23031169402939,0.));
#34649=CARTESIAN_POINT('Ctrl Pts',(-18.908024664264,3.23031169402939,18.));
#34650=CARTESIAN_POINT('Ctrl Pts',(-18.987055820781,3.22595008773715,0.));
#34651=CARTESIAN_POINT('Ctrl Pts',(-18.987055820781,3.22595008773715,18.));
#34652=CARTESIAN_POINT('Ctrl Pts',(-19.0661599344864,3.22090173651085,0.));
#34653=CARTESIAN_POINT('Ctrl Pts',(-19.0661599344864,3.22090173651085,18.));
#34654=CARTESIAN_POINT('Ctrl Pts',(-19.1453253990185,3.21510704576117,0.));
#34655=CARTESIAN_POINT('Ctrl Pts',(-19.1453253990185,3.21510704576117,18.));
#34656=CARTESIAN_POINT('Ctrl Pts',(-19.2245581120423,3.2083040369031,0.));
#34657=CARTESIAN_POINT('Ctrl Pts',(-19.2245581120423,3.2083040369031,18.));
#34658=CARTESIAN_POINT('Ctrl Pts',(-19.3038697977783,3.2001820370274,0.));
#34659=CARTESIAN_POINT('Ctrl Pts',(-19.3038697977783,3.2001820370274,18.));
#34660=CARTESIAN_POINT('Ctrl Pts',(-19.3832648965708,3.19055618489382,0.));
#34661=CARTESIAN_POINT('Ctrl Pts',(-19.3832648965708,3.19055618489382,18.));
#34662=CARTESIAN_POINT('Ctrl Pts',(-19.4627345689632,3.17944412249754,0.));
#34663=CARTESIAN_POINT('Ctrl Pts',(-19.4627345689632,3.17944412249754,18.));
#34664=CARTESIAN_POINT('Ctrl Pts',(-19.5422628528517,3.16697679689295,0.));
#34665=CARTESIAN_POINT('Ctrl Pts',(-19.5422628528517,3.16697679689295,18.));
#34666=CARTESIAN_POINT('Ctrl Pts',(-19.6218301288731,3.15334580802458,0.));
#34667=CARTESIAN_POINT('Ctrl Pts',(-19.6218301288731,3.15334580802458,18.));
#34668=CARTESIAN_POINT('Ctrl Pts',(-19.7014173131304,3.13874131344865,0.));
#34669=CARTESIAN_POINT('Ctrl Pts',(-19.7014173131304,3.13874131344865,18.));
#34670=CARTESIAN_POINT('Ctrl Pts',(-19.7810105986827,3.1232813132398,0.));
#34671=CARTESIAN_POINT('Ctrl Pts',(-19.7810105986827,3.1232813132398,18.));
#34672=CARTESIAN_POINT('Ctrl Pts',(-19.8606024365399,3.10699659920993,0.));
#34673=CARTESIAN_POINT('Ctrl Pts',(-19.8606024365399,3.10699659920993,18.));
#34674=CARTESIAN_POINT('Ctrl Pts',(-19.940188965354,3.08986795998319,0.));
#34675=CARTESIAN_POINT('Ctrl Pts',(-19.940188965354,3.08986795998319,18.));
#34676=CARTESIAN_POINT('Ctrl Pts',(-20.0197683853426,3.07184950717982,0.));
#34677=CARTESIAN_POINT('Ctrl Pts',(-20.0197683853426,3.07184950717982,18.));
#34678=CARTESIAN_POINT('Ctrl Pts',(-20.0993390992966,3.05289545759951,0.));
#34679=CARTESIAN_POINT('Ctrl Pts',(-20.0993390992966,3.05289545759951,18.));
#34680=CARTESIAN_POINT('Ctrl Pts',(-20.178897575607,3.03299094576289,0.));
#34681=CARTESIAN_POINT('Ctrl Pts',(-20.178897575607,3.03299094576289,18.));
#34682=CARTESIAN_POINT('Ctrl Pts',(-20.2584381977107,3.01215393913612,0.));
#34683=CARTESIAN_POINT('Ctrl Pts',(-20.2584381977107,3.01215393913612,18.));
#34684=CARTESIAN_POINT('Ctrl Pts',(-20.3379542578194,2.99042050197905,0.));
#34685=CARTESIAN_POINT('Ctrl Pts',(-20.3379542578194,2.99042050197905,18.));
#34686=CARTESIAN_POINT('Ctrl Pts',(-20.4174386170774,2.96783492132513,0.));
#34687=CARTESIAN_POINT('Ctrl Pts',(-20.4174386170774,2.96783492132513,18.));
#34688=CARTESIAN_POINT('Ctrl Pts',(-20.4968844460513,2.94443868035155,0.));
#34689=CARTESIAN_POINT('Ctrl Pts',(-20.4968844460513,2.94443868035155,18.));
#34690=CARTESIAN_POINT('Ctrl Pts',(-20.5762860772943,2.92025778619207,0.));
#34691=CARTESIAN_POINT('Ctrl Pts',(-20.5762860772943,2.92025778619207,18.));
#34692=CARTESIAN_POINT('Ctrl Pts',(-20.6556389450993,2.89530351700806,0.));
#34693=CARTESIAN_POINT('Ctrl Pts',(-20.6556389450993,2.89530351700806,18.));
#34694=CARTESIAN_POINT('Ctrl Pts',(-20.7349391669725,2.86957843933153,0.));
#34695=CARTESIAN_POINT('Ctrl Pts',(-20.7349391669725,2.86957843933153,18.));
#34696=CARTESIAN_POINT('Ctrl Pts',(-20.8141832346435,2.84308082507644,0.));
#34697=CARTESIAN_POINT('Ctrl Pts',(-20.8141832346435,2.84308082507644,18.));
#34698=CARTESIAN_POINT('Ctrl Pts',(-20.8933676828246,2.81580940715318,0.));
#34699=CARTESIAN_POINT('Ctrl Pts',(-20.8933676828246,2.81580940715318,18.));
#34700=CARTESIAN_POINT('Ctrl Pts',(-20.9724887103073,2.78776883747222,0.));
#34701=CARTESIAN_POINT('Ctrl Pts',(-20.9724887103073,2.78776883747222,18.));
#34702=CARTESIAN_POINT('Ctrl Pts',(-21.0515422162039,2.7589691000769,0.));
#34703=CARTESIAN_POINT('Ctrl Pts',(-21.0515422162039,2.7589691000769,18.));
#34704=CARTESIAN_POINT('Ctrl Pts',(-21.1305239619219,2.72942309852119,0.));
#34705=CARTESIAN_POINT('Ctrl Pts',(-21.1305239619219,2.72942309852119,18.));
#34706=CARTESIAN_POINT('Ctrl Pts',(-21.2094296949571,2.69914481283353,0.));
#34707=CARTESIAN_POINT('Ctrl Pts',(-21.2094296949571,2.69914481283353,18.));
#34708=CARTESIAN_POINT('Ctrl Pts',(-21.2882552797978,2.66814735708301,0.));
#34709=CARTESIAN_POINT('Ctrl Pts',(-21.2882552797978,2.66814735708301,18.));
#34710=CARTESIAN_POINT('Ctrl Pts',(-21.3669968505594,2.6364407451853,0.));
#34711=CARTESIAN_POINT('Ctrl Pts',(-21.3669968505594,2.6364407451853,18.));
#34712=CARTESIAN_POINT('Ctrl Pts',(-21.4456507822983,2.60403221866524,0.));
#34713=CARTESIAN_POINT('Ctrl Pts',(-21.4456507822983,2.60403221866524,18.));
#34714=CARTESIAN_POINT('Ctrl Pts',(-21.5242136128466,2.57092728351981,0.));
#34715=CARTESIAN_POINT('Ctrl Pts',(-21.5242136128466,2.57092728351981,18.));
#34716=CARTESIAN_POINT('Ctrl Pts',(-21.6026819803014,2.53713053453767,0.));
#34717=CARTESIAN_POINT('Ctrl Pts',(-21.6026819803014,2.53713053453767,18.));
#34718=CARTESIAN_POINT('Ctrl Pts',(-21.6810525594039,2.50264651177235,0.));
#34719=CARTESIAN_POINT('Ctrl Pts',(-21.6810525594039,2.50264651177235,18.));
#34720=CARTESIAN_POINT('Ctrl Pts',(-21.7593219872847,2.46748070362076,0.));
#34721=CARTESIAN_POINT('Ctrl Pts',(-21.7593219872847,2.46748070362076,18.));
#34722=CARTESIAN_POINT('Ctrl Pts',(-21.8374868743435,2.43163944362692,0.));
#34723=CARTESIAN_POINT('Ctrl Pts',(-21.8374868743435,2.43163944362692,18.));
#34724=CARTESIAN_POINT('Ctrl Pts',(-21.9155438409279,2.39512947344577,0.));
#34725=CARTESIAN_POINT('Ctrl Pts',(-21.9155438409279,2.39512947344577,18.));
#34726=CARTESIAN_POINT('Ctrl Pts',(-21.9934895476958,2.35795761145762,0.));
#34727=CARTESIAN_POINT('Ctrl Pts',(-21.9934895476958,2.35795761145762,18.));
#34728=CARTESIAN_POINT('Ctrl Pts',(-22.0713207257413,2.32013040994125,0.));
#34729=CARTESIAN_POINT('Ctrl Pts',(-22.0713207257413,2.32013040994125,18.));
#34730=CARTESIAN_POINT('Ctrl Pts',(-22.1490342171802,2.28165375160231,0.));
#34731=CARTESIAN_POINT('Ctrl Pts',(-22.1490342171802,2.28165375160231,18.));
#34732=CARTESIAN_POINT('Ctrl Pts',(-22.2266269576315,2.24253288454712,0.));
#34733=CARTESIAN_POINT('Ctrl Pts',(-22.2266269576315,2.24253288454712,18.));
#34734=CARTESIAN_POINT('Ctrl Pts',(-22.3040959372933,2.202772632214,0.));
#34735=CARTESIAN_POINT('Ctrl Pts',(-22.3040959372933,2.202772632214,18.));
#34736=CARTESIAN_POINT('Ctrl Pts',(-22.3814381677224,2.16237755726405,0.));
#34737=CARTESIAN_POINT('Ctrl Pts',(-22.3814381677224,2.16237755726405,18.));
#34738=CARTESIAN_POINT('Ctrl Pts',(-22.4586506520939,2.1213521324248,0.));
#34739=CARTESIAN_POINT('Ctrl Pts',(-22.4586506520939,2.1213521324248,18.));
#34740=CARTESIAN_POINT('Ctrl Pts',(-22.5357303426251,2.07970095436224,0.));
#34741=CARTESIAN_POINT('Ctrl Pts',(-22.5357303426251,2.07970095436224,18.));
#34742=CARTESIAN_POINT('Ctrl Pts',(-22.6126741632309,2.03742874317627,0.));
#34743=CARTESIAN_POINT('Ctrl Pts',(-22.6126741632309,2.03742874317627,18.));
#34744=CARTESIAN_POINT('Ctrl Pts',(-22.6894790673923,1.99454021984253,0.));
#34745=CARTESIAN_POINT('Ctrl Pts',(-22.6894790673923,1.99454021984253,18.));
#34746=CARTESIAN_POINT('Ctrl Pts',(-22.7661420906702,1.95104002082891,0.));
#34747=CARTESIAN_POINT('Ctrl Pts',(-22.7661420906702,1.95104002082891,18.));
#34748=CARTESIAN_POINT('Ctrl Pts',(-22.8426603964871,1.90693261239855,0.));
#34749=CARTESIAN_POINT('Ctrl Pts',(-22.8426603964871,1.90693261239855,18.));
#34750=CARTESIAN_POINT('Ctrl Pts',(-22.9190313507225,1.86222218327819,0.));
#34751=CARTESIAN_POINT('Ctrl Pts',(-22.9190313507225,1.86222218327819,18.));
#34752=CARTESIAN_POINT('Ctrl Pts',(-22.9952524859917,1.81691265597282,0.));
#34753=CARTESIAN_POINT('Ctrl Pts',(-22.9952524859917,1.81691265597282,18.));
#34754=CARTESIAN_POINT('Ctrl Pts',(-23.0713213684573,1.77100780743078,0.));
#34755=CARTESIAN_POINT('Ctrl Pts',(-23.0713213684573,1.77100780743078,18.));
#34756=CARTESIAN_POINT('Ctrl Pts',(-23.1472354850579,1.72451136919382,0.));
#34757=CARTESIAN_POINT('Ctrl Pts',(-23.1472354850579,1.72451136919382,18.));
#34758=CARTESIAN_POINT('Ctrl Pts',(-23.2229921402299,1.67742712670823,0.));
#34759=CARTESIAN_POINT('Ctrl Pts',(-23.2229921402299,1.67742712670823,18.));
#34760=CARTESIAN_POINT('Ctrl Pts',(-23.2985883089733,1.62975905604583,0.));
#34761=CARTESIAN_POINT('Ctrl Pts',(-23.2985883089733,1.62975905604583,18.));
#34762=CARTESIAN_POINT('Ctrl Pts',(-23.3740206492924,1.58151133638848,0.));
#34763=CARTESIAN_POINT('Ctrl Pts',(-23.3740206492924,1.58151133638848,18.));
#34764=CARTESIAN_POINT('Ctrl Pts',(-23.4492857841673,1.53268814658653,0.));
#34765=CARTESIAN_POINT('Ctrl Pts',(-23.4492857841673,1.53268814658653,18.));
#34766=CARTESIAN_POINT('Ctrl Pts',(-23.5243805284282,1.48329351290851,0.));
#34767=CARTESIAN_POINT('Ctrl Pts',(-23.5243805284282,1.48329351290851,18.));
#34768=CARTESIAN_POINT('Ctrl Pts',(-23.5993021272808,1.4333311444639,0.));
#34769=CARTESIAN_POINT('Ctrl Pts',(-23.5993021272808,1.4333311444639,18.));
#34770=CARTESIAN_POINT('Ctrl Pts',(-23.6740485197917,1.38280426780156,0.));
#34771=CARTESIAN_POINT('Ctrl Pts',(-23.6740485197917,1.38280426780156,18.));
#34772=CARTESIAN_POINT('Ctrl Pts',(-23.748618507953,1.3317154958625,0.));
#34773=CARTESIAN_POINT('Ctrl Pts',(-23.748618507953,1.3317154958625,18.));
#34774=CARTESIAN_POINT('Ctrl Pts',(-23.8230115078373,1.28006684869166,0.));
#34775=CARTESIAN_POINT('Ctrl Pts',(-23.8230115078373,1.28006684869166,18.));
#34776=CARTESIAN_POINT('Ctrl Pts',(-23.8823841929226,1.23830117308931,0.));
#34777=CARTESIAN_POINT('Ctrl Pts',(-23.8823841929226,1.23830117308931,18.));
#34778=CARTESIAN_POINT('Ctrl Pts',(-23.9268340213744,1.20672599652273,0.));
#34779=CARTESIAN_POINT('Ctrl Pts',(-23.9268340213744,1.20672599652273,18.));
#34780=CARTESIAN_POINT('Ctrl Pts',(-23.9564318364582,1.18556439589232,0.));
#34781=CARTESIAN_POINT('Ctrl Pts',(-23.9564318364582,1.18556439589232,18.));
#34782=CARTESIAN_POINT('Ctrl Pts',(-23.9712218930251,1.17495572484832,0.));
#34783=CARTESIAN_POINT('Ctrl Pts',(-23.9712218930251,1.17495572484832,18.));
#34784=CARTESIAN_POINT('Ctrl Pts',(-18.5165898451125,3.2163316265074,0.));
#34785=CARTESIAN_POINT('Ctrl Pts',(-18.5320375674878,3.21901489585931,0.));
#34786=CARTESIAN_POINT('Ctrl Pts',(-18.5629852384321,3.22384302136592,0.));
#34787=CARTESIAN_POINT('Ctrl Pts',(-18.6095634206219,3.22947000444161,0.));
#34788=CARTESIAN_POINT('Ctrl Pts',(-18.6719665316945,3.23390622002644,0.));
#34789=CARTESIAN_POINT('Ctrl Pts',(-18.7503838921122,3.23528809328097,0.));
#34790=CARTESIAN_POINT('Ctrl Pts',(-18.8291062617862,3.2337009106567,0.));
#34791=CARTESIAN_POINT('Ctrl Pts',(-18.908024664264,3.23031169402939,0.));
#34792=CARTESIAN_POINT('Ctrl Pts',(-18.987055820781,3.22595008773715,0.));
#34793=CARTESIAN_POINT('Ctrl Pts',(-19.0661599344864,3.22090173651085,0.));
#34794=CARTESIAN_POINT('Ctrl Pts',(-19.1453253990185,3.21510704576117,0.));
#34795=CARTESIAN_POINT('Ctrl Pts',(-19.2245581120423,3.2083040369031,0.));
#34796=CARTESIAN_POINT('Ctrl Pts',(-19.3038697977783,3.2001820370274,0.));
#34797=CARTESIAN_POINT('Ctrl Pts',(-19.3832648965708,3.19055618489382,0.));
#34798=CARTESIAN_POINT('Ctrl Pts',(-19.4627345689632,3.17944412249754,0.));
#34799=CARTESIAN_POINT('Ctrl Pts',(-19.5422628528517,3.16697679689295,0.));
#34800=CARTESIAN_POINT('Ctrl Pts',(-19.6218301288731,3.15334580802458,0.));
#34801=CARTESIAN_POINT('Ctrl Pts',(-19.7014173131304,3.13874131344865,0.));
#34802=CARTESIAN_POINT('Ctrl Pts',(-19.7810105986827,3.1232813132398,0.));
#34803=CARTESIAN_POINT('Ctrl Pts',(-19.8606024365399,3.10699659920993,0.));
#34804=CARTESIAN_POINT('Ctrl Pts',(-19.940188965354,3.08986795998319,0.));
#34805=CARTESIAN_POINT('Ctrl Pts',(-20.0197683853426,3.07184950717982,0.));
#34806=CARTESIAN_POINT('Ctrl Pts',(-20.0993390992966,3.05289545759951,0.));
#34807=CARTESIAN_POINT('Ctrl Pts',(-20.178897575607,3.03299094576289,0.));
#34808=CARTESIAN_POINT('Ctrl Pts',(-20.2584381977107,3.01215393913612,0.));
#34809=CARTESIAN_POINT('Ctrl Pts',(-20.3379542578194,2.99042050197905,0.));
#34810=CARTESIAN_POINT('Ctrl Pts',(-20.4174386170774,2.96783492132513,0.));
#34811=CARTESIAN_POINT('Ctrl Pts',(-20.4968844460513,2.94443868035155,0.));
#34812=CARTESIAN_POINT('Ctrl Pts',(-20.5762860772943,2.92025778619207,0.));
#34813=CARTESIAN_POINT('Ctrl Pts',(-20.6556389450993,2.89530351700806,0.));
#34814=CARTESIAN_POINT('Ctrl Pts',(-20.7349391669725,2.86957843933153,0.));
#34815=CARTESIAN_POINT('Ctrl Pts',(-20.8141832346435,2.84308082507644,0.));
#34816=CARTESIAN_POINT('Ctrl Pts',(-20.8933676828246,2.81580940715318,0.));
#34817=CARTESIAN_POINT('Ctrl Pts',(-20.9724887103073,2.78776883747222,0.));
#34818=CARTESIAN_POINT('Ctrl Pts',(-21.0515422162039,2.7589691000769,0.));
#34819=CARTESIAN_POINT('Ctrl Pts',(-21.1305239619219,2.72942309852119,0.));
#34820=CARTESIAN_POINT('Ctrl Pts',(-21.2094296949571,2.69914481283353,0.));
#34821=CARTESIAN_POINT('Ctrl Pts',(-21.2882552797978,2.66814735708301,0.));
#34822=CARTESIAN_POINT('Ctrl Pts',(-21.3669968505594,2.6364407451853,0.));
#34823=CARTESIAN_POINT('Ctrl Pts',(-21.4456507822983,2.60403221866524,0.));
#34824=CARTESIAN_POINT('Ctrl Pts',(-21.5242136128466,2.57092728351981,0.));
#34825=CARTESIAN_POINT('Ctrl Pts',(-21.6026819803014,2.53713053453767,0.));
#34826=CARTESIAN_POINT('Ctrl Pts',(-21.6810525594039,2.50264651177235,0.));
#34827=CARTESIAN_POINT('Ctrl Pts',(-21.7593219872847,2.46748070362076,0.));
#34828=CARTESIAN_POINT('Ctrl Pts',(-21.8374868743435,2.43163944362692,0.));
#34829=CARTESIAN_POINT('Ctrl Pts',(-21.9155438409279,2.39512947344577,0.));
#34830=CARTESIAN_POINT('Ctrl Pts',(-21.9934895476958,2.35795761145762,0.));
#34831=CARTESIAN_POINT('Ctrl Pts',(-22.0713207257413,2.32013040994125,0.));
#34832=CARTESIAN_POINT('Ctrl Pts',(-22.1490342171802,2.28165375160231,0.));
#34833=CARTESIAN_POINT('Ctrl Pts',(-22.2266269576315,2.24253288454712,0.));
#34834=CARTESIAN_POINT('Ctrl Pts',(-22.3040959372933,2.202772632214,0.));
#34835=CARTESIAN_POINT('Ctrl Pts',(-22.3814381677224,2.16237755726405,0.));
#34836=CARTESIAN_POINT('Ctrl Pts',(-22.4586506520939,2.1213521324248,0.));
#34837=CARTESIAN_POINT('Ctrl Pts',(-22.5357303426251,2.07970095436224,0.));
#34838=CARTESIAN_POINT('Ctrl Pts',(-22.6126741632309,2.03742874317627,0.));
#34839=CARTESIAN_POINT('Ctrl Pts',(-22.6894790673923,1.99454021984253,0.));
#34840=CARTESIAN_POINT('Ctrl Pts',(-22.7661420906702,1.95104002082891,0.));
#34841=CARTESIAN_POINT('Ctrl Pts',(-22.8426603964871,1.90693261239855,0.));
#34842=CARTESIAN_POINT('Ctrl Pts',(-22.9190313507225,1.86222218327819,0.));
#34843=CARTESIAN_POINT('Ctrl Pts',(-22.9952524859917,1.81691265597282,0.));
#34844=CARTESIAN_POINT('Ctrl Pts',(-23.0713213684573,1.77100780743078,0.));
#34845=CARTESIAN_POINT('Ctrl Pts',(-23.1472354850579,1.72451136919382,0.));
#34846=CARTESIAN_POINT('Ctrl Pts',(-23.2229921402299,1.67742712670823,0.));
#34847=CARTESIAN_POINT('Ctrl Pts',(-23.2985883089733,1.62975905604583,0.));
#34848=CARTESIAN_POINT('Ctrl Pts',(-23.3740206492924,1.58151133638848,0.));
#34849=CARTESIAN_POINT('Ctrl Pts',(-23.4492857841673,1.53268814658653,0.));
#34850=CARTESIAN_POINT('Ctrl Pts',(-23.5243805284282,1.48329351290851,0.));
#34851=CARTESIAN_POINT('Ctrl Pts',(-23.5993021272808,1.4333311444639,0.));
#34852=CARTESIAN_POINT('Ctrl Pts',(-23.6740485197917,1.38280426780156,0.));
#34853=CARTESIAN_POINT('Ctrl Pts',(-23.7635325055853,1.32149774147469,0.));
#34854=CARTESIAN_POINT('Ctrl Pts',(-23.8378812584003,1.2697091254959,0.));
#34855=CARTESIAN_POINT('Ctrl Pts',(-23.89721850443,1.22783185562045,0.));
#34856=CARTESIAN_POINT('Ctrl Pts',(-23.9416417798466,1.19617306697387,0.));
#34857=CARTESIAN_POINT('Ctrl Pts',(-23.9712218930251,1.17495572484832,0.));
#34858=CARTESIAN_POINT('Ctrl Pts',(-18.5165898451125,3.2163316265074,15.));
#34859=CARTESIAN_POINT('Ctrl Pts',(-18.5320375674878,3.21901489585931,15.));
#34860=CARTESIAN_POINT('Ctrl Pts',(-18.5629852384321,3.22384302136592,15.));
#34861=CARTESIAN_POINT('Ctrl Pts',(-18.6095634206219,3.22947000444161,15.));
#34862=CARTESIAN_POINT('Ctrl Pts',(-18.6719665316945,3.23390622002644,15.));
#34863=CARTESIAN_POINT('Ctrl Pts',(-18.7503838921122,3.23528809328097,15.));
#34864=CARTESIAN_POINT('Ctrl Pts',(-18.8291062617862,3.2337009106567,15.));
#34865=CARTESIAN_POINT('Ctrl Pts',(-18.908024664264,3.23031169402939,15.));
#34866=CARTESIAN_POINT('Ctrl Pts',(-18.987055820781,3.22595008773715,15.));
#34867=CARTESIAN_POINT('Ctrl Pts',(-19.0661599344864,3.22090173651085,15.));
#34868=CARTESIAN_POINT('Ctrl Pts',(-19.1453253990185,3.21510704576117,15.));
#34869=CARTESIAN_POINT('Ctrl Pts',(-19.2245581120423,3.2083040369031,15.));
#34870=CARTESIAN_POINT('Ctrl Pts',(-19.3038697977783,3.2001820370274,15.));
#34871=CARTESIAN_POINT('Ctrl Pts',(-19.3832648965708,3.19055618489382,15.));
#34872=CARTESIAN_POINT('Ctrl Pts',(-19.4627345689632,3.17944412249754,15.));
#34873=CARTESIAN_POINT('Ctrl Pts',(-19.5422628528517,3.16697679689295,15.));
#34874=CARTESIAN_POINT('Ctrl Pts',(-19.6218301288731,3.15334580802458,15.));
#34875=CARTESIAN_POINT('Ctrl Pts',(-19.7014173131304,3.13874131344865,15.));
#34876=CARTESIAN_POINT('Ctrl Pts',(-19.7810105986827,3.1232813132398,15.));
#34877=CARTESIAN_POINT('Ctrl Pts',(-19.8606024365399,3.10699659920993,15.));
#34878=CARTESIAN_POINT('Ctrl Pts',(-19.940188965354,3.08986795998319,15.));
#34879=CARTESIAN_POINT('Ctrl Pts',(-20.0197683853426,3.07184950717982,15.));
#34880=CARTESIAN_POINT('Ctrl Pts',(-20.0993390992966,3.05289545759951,15.));
#34881=CARTESIAN_POINT('Ctrl Pts',(-20.178897575607,3.03299094576289,15.));
#34882=CARTESIAN_POINT('Ctrl Pts',(-20.2584381977107,3.01215393913612,15.));
#34883=CARTESIAN_POINT('Ctrl Pts',(-20.3379542578194,2.99042050197905,15.));
#34884=CARTESIAN_POINT('Ctrl Pts',(-20.4174386170774,2.96783492132513,15.));
#34885=CARTESIAN_POINT('Ctrl Pts',(-20.4968844460513,2.94443868035155,15.));
#34886=CARTESIAN_POINT('Ctrl Pts',(-20.5762860772943,2.92025778619207,15.));
#34887=CARTESIAN_POINT('Ctrl Pts',(-20.6556389450993,2.89530351700806,15.));
#34888=CARTESIAN_POINT('Ctrl Pts',(-20.7349391669725,2.86957843933153,15.));
#34889=CARTESIAN_POINT('Ctrl Pts',(-20.8141832346435,2.84308082507644,15.));
#34890=CARTESIAN_POINT('Ctrl Pts',(-20.8933676828246,2.81580940715318,15.));
#34891=CARTESIAN_POINT('Ctrl Pts',(-20.9724887103073,2.78776883747222,15.));
#34892=CARTESIAN_POINT('Ctrl Pts',(-21.0515422162039,2.7589691000769,15.));
#34893=CARTESIAN_POINT('Ctrl Pts',(-21.1305239619219,2.72942309852119,15.));
#34894=CARTESIAN_POINT('Ctrl Pts',(-21.2094296949571,2.69914481283353,15.));
#34895=CARTESIAN_POINT('Ctrl Pts',(-21.2882552797978,2.66814735708301,15.));
#34896=CARTESIAN_POINT('Ctrl Pts',(-21.3669968505594,2.6364407451853,15.));
#34897=CARTESIAN_POINT('Ctrl Pts',(-21.4456507822983,2.60403221866524,15.));
#34898=CARTESIAN_POINT('Ctrl Pts',(-21.5242136128466,2.57092728351981,15.));
#34899=CARTESIAN_POINT('Ctrl Pts',(-21.6026819803014,2.53713053453767,15.));
#34900=CARTESIAN_POINT('Ctrl Pts',(-21.6810525594039,2.50264651177235,15.));
#34901=CARTESIAN_POINT('Ctrl Pts',(-21.7593219872847,2.46748070362076,15.));
#34902=CARTESIAN_POINT('Ctrl Pts',(-21.8374868743435,2.43163944362692,15.));
#34903=CARTESIAN_POINT('Ctrl Pts',(-21.9155438409279,2.39512947344577,15.));
#34904=CARTESIAN_POINT('Ctrl Pts',(-21.9934895476958,2.35795761145762,15.));
#34905=CARTESIAN_POINT('Ctrl Pts',(-22.0713207257413,2.32013040994125,15.));
#34906=CARTESIAN_POINT('Ctrl Pts',(-22.1490342171802,2.28165375160231,15.));
#34907=CARTESIAN_POINT('Ctrl Pts',(-22.2266269576315,2.24253288454712,15.));
#34908=CARTESIAN_POINT('Ctrl Pts',(-22.3040959372933,2.202772632214,15.));
#34909=CARTESIAN_POINT('Ctrl Pts',(-22.3814381677224,2.16237755726405,15.));
#34910=CARTESIAN_POINT('Ctrl Pts',(-22.4586506520939,2.1213521324248,15.));
#34911=CARTESIAN_POINT('Ctrl Pts',(-22.5357303426251,2.07970095436224,15.));
#34912=CARTESIAN_POINT('Ctrl Pts',(-22.6126741632309,2.03742874317627,15.));
#34913=CARTESIAN_POINT('Ctrl Pts',(-22.6894790673923,1.99454021984253,15.));
#34914=CARTESIAN_POINT('Ctrl Pts',(-22.7661420906702,1.95104002082891,15.));
#34915=CARTESIAN_POINT('Ctrl Pts',(-22.8426603964871,1.90693261239855,15.));
#34916=CARTESIAN_POINT('Ctrl Pts',(-22.9190313507225,1.86222218327819,15.));
#34917=CARTESIAN_POINT('Ctrl Pts',(-22.9952524859917,1.81691265597282,15.));
#34918=CARTESIAN_POINT('Ctrl Pts',(-23.0713213684573,1.77100780743078,15.));
#34919=CARTESIAN_POINT('Ctrl Pts',(-23.1472354850579,1.72451136919382,15.));
#34920=CARTESIAN_POINT('Ctrl Pts',(-23.2229921402299,1.67742712670823,15.));
#34921=CARTESIAN_POINT('Ctrl Pts',(-23.2985883089733,1.62975905604583,15.));
#34922=CARTESIAN_POINT('Ctrl Pts',(-23.3740206492924,1.58151133638848,15.));
#34923=CARTESIAN_POINT('Ctrl Pts',(-23.4492857841673,1.53268814658653,15.));
#34924=CARTESIAN_POINT('Ctrl Pts',(-23.5243805284282,1.48329351290851,15.));
#34925=CARTESIAN_POINT('Ctrl Pts',(-23.5993021272808,1.4333311444639,15.));
#34926=CARTESIAN_POINT('Ctrl Pts',(-23.6740485197917,1.38280426780156,15.));
#34927=CARTESIAN_POINT('Ctrl Pts',(-23.7635325055853,1.32149774147469,15.));
#34928=CARTESIAN_POINT('Ctrl Pts',(-23.8378812584003,1.2697091254959,15.));
#34929=CARTESIAN_POINT('Ctrl Pts',(-23.89721850443,1.22783185562045,15.));
#34930=CARTESIAN_POINT('Ctrl Pts',(-23.9416417798466,1.19617306697387,15.));
#34931=CARTESIAN_POINT('Ctrl Pts',(-23.9712218930251,1.17495572484832,15.));
#34932=CARTESIAN_POINT('Ctrl Pts',(-20.0837475345526,13.1393715591102,0.));
#34933=CARTESIAN_POINT('Ctrl Pts',(-20.0837475345526,13.1393715591102,18.));
#34934=CARTESIAN_POINT('Ctrl Pts',(-20.0780177478283,13.1220955868173,0.));
#34935=CARTESIAN_POINT('Ctrl Pts',(-20.0780177478283,13.1220955868173,18.));
#34936=CARTESIAN_POINT('Ctrl Pts',(-20.0665110891946,13.0875783330728,0.));
#34937=CARTESIAN_POINT('Ctrl Pts',(-20.0665110891946,13.0875783330728,18.));
#34938=CARTESIAN_POINT('Ctrl Pts',(-20.0491098457044,13.0359065249991,0.));
#34939=CARTESIAN_POINT('Ctrl Pts',(-20.0491098457044,13.0359065249991,18.));
#34940=CARTESIAN_POINT('Ctrl Pts',(-20.0256255826397,12.9672189949731,0.));
#34941=CARTESIAN_POINT('Ctrl Pts',(-20.0256255826397,12.9672189949731,18.));
#34942=CARTESIAN_POINT('Ctrl Pts',(-19.9957986945787,12.8817072534696,0.));
#34943=CARTESIAN_POINT('Ctrl Pts',(-19.9957986945787,12.8817072534696,18.));
#34944=CARTESIAN_POINT('Ctrl Pts',(-19.9654995335894,12.7965444294443,0.));
#34945=CARTESIAN_POINT('Ctrl Pts',(-19.9654995335894,12.7965444294443,18.));
#34946=CARTESIAN_POINT('Ctrl Pts',(-19.9347273847264,12.7117325003719,0.));
#34947=CARTESIAN_POINT('Ctrl Pts',(-19.9347273847264,12.7117325003719,18.));
#34948=CARTESIAN_POINT('Ctrl Pts',(-19.9034816813503,12.6272742843372,0.));
#34949=CARTESIAN_POINT('Ctrl Pts',(-19.9034816813503,12.6272742843372,18.));
#34950=CARTESIAN_POINT('Ctrl Pts',(-19.8717621942733,12.5431736030596,0.));
#34951=CARTESIAN_POINT('Ctrl Pts',(-19.8717621942733,12.5431736030596,18.));
#34952=CARTESIAN_POINT('Ctrl Pts',(-19.839568972011,12.4594350764989,0.));
#34953=CARTESIAN_POINT('Ctrl Pts',(-19.839568972011,12.4594350764989,18.));
#34954=CARTESIAN_POINT('Ctrl Pts',(-19.8069022248387,12.3760638341708,0.));
#34955=CARTESIAN_POINT('Ctrl Pts',(-19.8069022248387,12.3760638341708,18.));
#34956=CARTESIAN_POINT('Ctrl Pts',(-19.7737622285562,12.2930652417987,0.));
#34957=CARTESIAN_POINT('Ctrl Pts',(-19.7737622285562,12.2930652417987,18.));
#34958=CARTESIAN_POINT('Ctrl Pts',(-19.7401492304335,12.2104446447874,0.));
#34959=CARTESIAN_POINT('Ctrl Pts',(-19.7401492304335,12.2104446447874,18.));
#34960=CARTESIAN_POINT('Ctrl Pts',(-19.7060633406705,12.1282070378972,0.));
#34961=CARTESIAN_POINT('Ctrl Pts',(-19.7060633406705,12.1282070378972,18.));
#34962=CARTESIAN_POINT('Ctrl Pts',(-19.6715045149944,12.0463570680309,0.));
#34963=CARTESIAN_POINT('Ctrl Pts',(-19.6715045149944,12.0463570680309,18.));
#34964=CARTESIAN_POINT('Ctrl Pts',(-19.6364725931695,11.9648992312094,0.));
#34965=CARTESIAN_POINT('Ctrl Pts',(-19.6364725931695,11.9648992312094,18.));
#34966=CARTESIAN_POINT('Ctrl Pts',(-19.6009673241771,11.8838380136222,0.));
#34967=CARTESIAN_POINT('Ctrl Pts',(-19.6009673241771,11.8838380136222,18.));
#34968=CARTESIAN_POINT('Ctrl Pts',(-19.5649883985826,11.8031780389346,0.));
#34969=CARTESIAN_POINT('Ctrl Pts',(-19.5649883985826,11.8031780389346,18.));
#34970=CARTESIAN_POINT('Ctrl Pts',(-19.5285354853626,11.722924244195,0.));
#34971=CARTESIAN_POINT('Ctrl Pts',(-19.5285354853626,11.722924244195,18.));
#34972=CARTESIAN_POINT('Ctrl Pts',(-19.4916082541529,11.6430819099846,0.));
#34973=CARTESIAN_POINT('Ctrl Pts',(-19.4916082541529,11.6430819099846,18.));
#34974=CARTESIAN_POINT('Ctrl Pts',(-19.4542063779876,11.5636565297382,0.));
#34975=CARTESIAN_POINT('Ctrl Pts',(-19.4542063779876,11.5636565297382,18.));
#34976=CARTESIAN_POINT('Ctrl Pts',(-19.4163295466324,11.4846537135043,0.));
#34977=CARTESIAN_POINT('Ctrl Pts',(-19.4163295466324,11.4846537135043,18.));
#34978=CARTESIAN_POINT('Ctrl Pts',(-19.3779774742875,11.4060790880015,0.));
#34979=CARTESIAN_POINT('Ctrl Pts',(-19.3779774742875,11.4060790880015,18.));
#34980=CARTESIAN_POINT('Ctrl Pts',(-19.3391499248083,11.3279381634523,0.));
#34981=CARTESIAN_POINT('Ctrl Pts',(-19.3391499248083,11.3279381634523,18.));
#34982=CARTESIAN_POINT('Ctrl Pts',(-19.2998466936739,11.2502363198588,0.));
#34983=CARTESIAN_POINT('Ctrl Pts',(-19.2998466936739,11.2502363198588,18.));
#34984=CARTESIAN_POINT('Ctrl Pts',(-19.2600675167206,11.1729790050543,0.));
#34985=CARTESIAN_POINT('Ctrl Pts',(-19.2600675167206,11.1729790050543,18.));
#34986=CARTESIAN_POINT('Ctrl Pts',(-19.2198119937835,11.0961718903994,0.));
#34987=CARTESIAN_POINT('Ctrl Pts',(-19.2198119937835,11.0961718903994,18.));
#34988=CARTESIAN_POINT('Ctrl Pts',(-19.1790795192393,11.0198210228993,0.));
#34989=CARTESIAN_POINT('Ctrl Pts',(-19.1790795192393,11.0198210228993,18.));
#34990=CARTESIAN_POINT('Ctrl Pts',(-19.1378691901023,10.9439330179206,0.));
#34991=CARTESIAN_POINT('Ctrl Pts',(-19.1378691901023,10.9439330179206,18.));
#34992=CARTESIAN_POINT('Ctrl Pts',(-19.0961797996403,10.868515097783,0.));
#34993=CARTESIAN_POINT('Ctrl Pts',(-19.0961797996403,10.868515097783,18.));
#34994=CARTESIAN_POINT('Ctrl Pts',(-19.0540100416943,10.7935747414879,0.));
#34995=CARTESIAN_POINT('Ctrl Pts',(-19.0540100416943,10.7935747414879,18.));
#34996=CARTESIAN_POINT('Ctrl Pts',(-19.0113586878152,10.7191193896586,0.));
#34997=CARTESIAN_POINT('Ctrl Pts',(-19.0113586878152,10.7191193896586,18.));
#34998=CARTESIAN_POINT('Ctrl Pts',(-18.9682247574834,10.6451561585969,0.));
#34999=CARTESIAN_POINT('Ctrl Pts',(-18.9682247574834,10.6451561585969,18.));
#35000=CARTESIAN_POINT('Ctrl Pts',(-18.9246077453188,10.5716914651544,0.));
#35001=CARTESIAN_POINT('Ctrl Pts',(-18.9246077453188,10.5716914651544,18.));
#35002=CARTESIAN_POINT('Ctrl Pts',(-18.8805076729356,10.4987309368494,0.));
#35003=CARTESIAN_POINT('Ctrl Pts',(-18.8805076729356,10.4987309368494,18.));
#35004=CARTESIAN_POINT('Ctrl Pts',(-18.8359245594214,10.4262802670211,0.));
#35005=CARTESIAN_POINT('Ctrl Pts',(-18.8359245594214,10.4262802670211,18.));
#35006=CARTESIAN_POINT('Ctrl Pts',(-18.7908579693851,10.3543459451258,0.));
#35007=CARTESIAN_POINT('Ctrl Pts',(-18.7908579693851,10.3543459451258,18.));
#35008=CARTESIAN_POINT('Ctrl Pts',(-18.7453065790062,10.2829359603685,0.));
#35009=CARTESIAN_POINT('Ctrl Pts',(-18.7453065790062,10.2829359603685,18.));
#35010=CARTESIAN_POINT('Ctrl Pts',(-18.699267629819,10.2120606864872,0.));
#35011=CARTESIAN_POINT('Ctrl Pts',(-18.699267629819,10.2120606864872,18.));
#35012=CARTESIAN_POINT('Ctrl Pts',(-18.6527367592664,10.1417331637795,0.));
#35013=CARTESIAN_POINT('Ctrl Pts',(-18.6527367592664,10.1417331637795,18.));
#35014=CARTESIAN_POINT('Ctrl Pts',(-18.605709190442,10.0719672018851,0.));
#35015=CARTESIAN_POINT('Ctrl Pts',(-18.605709190442,10.0719672018851,18.));
#35016=CARTESIAN_POINT('Ctrl Pts',(-18.5581807679204,10.0027757313807,0.));
#35017=CARTESIAN_POINT('Ctrl Pts',(-18.5581807679204,10.0027757313807,18.));
#35018=CARTESIAN_POINT('Ctrl Pts',(-18.5101489409161,9.93416923996829,0.));
#35019=CARTESIAN_POINT('Ctrl Pts',(-18.5101489409161,9.93416923996829,18.));
#35020=CARTESIAN_POINT('Ctrl Pts',(-18.461614050347,9.86615372541685,0.));
#35021=CARTESIAN_POINT('Ctrl Pts',(-18.461614050347,9.86615372541685,18.));
#35022=CARTESIAN_POINT('Ctrl Pts',(-18.4125796444662,9.79873019947434,0.));
#35023=CARTESIAN_POINT('Ctrl Pts',(-18.4125796444662,9.79873019947434,18.));
#35024=CARTESIAN_POINT('Ctrl Pts',(-18.3630495772677,9.73189932619939,0.));
#35025=CARTESIAN_POINT('Ctrl Pts',(-18.3630495772677,9.73189932619939,18.));
#35026=CARTESIAN_POINT('Ctrl Pts',(-18.3130254811852,9.6656654640326,0.));
#35027=CARTESIAN_POINT('Ctrl Pts',(-18.3130254811852,9.6656654640326,18.));
#35028=CARTESIAN_POINT('Ctrl Pts',(-18.2625044208165,9.60004042085347,0.));
#35029=CARTESIAN_POINT('Ctrl Pts',(-18.2625044208165,9.60004042085347,18.));
#35030=CARTESIAN_POINT('Ctrl Pts',(-18.2114756946126,9.53504856811685,0.));
#35031=CARTESIAN_POINT('Ctrl Pts',(-18.2114756946126,9.53504856811685,18.));
#35032=CARTESIAN_POINT('Ctrl Pts',(-18.1599204445014,9.47072748065832,0.));
#35033=CARTESIAN_POINT('Ctrl Pts',(-18.1599204445014,9.47072748065832,18.));
#35034=CARTESIAN_POINT('Ctrl Pts',(-18.1078184146735,9.40711718355464,0.));
#35035=CARTESIAN_POINT('Ctrl Pts',(-18.1078184146735,9.40711718355464,18.));
#35036=CARTESIAN_POINT('Ctrl Pts',(-18.0551538338035,9.34425079614396,0.));
#35037=CARTESIAN_POINT('Ctrl Pts',(-18.0551538338035,9.34425079614396,18.));
#35038=CARTESIAN_POINT('Ctrl Pts',(-18.0019206847747,9.28214615574471,0.));
#35039=CARTESIAN_POINT('Ctrl Pts',(-18.0019206847747,9.28214615574471,18.));
#35040=CARTESIAN_POINT('Ctrl Pts',(-17.9481305624284,9.22079331175917,0.));
#35041=CARTESIAN_POINT('Ctrl Pts',(-17.9481305624284,9.22079331175917,18.));
#35042=CARTESIAN_POINT('Ctrl Pts',(-17.8938116696237,9.1601561636161,0.));
#35043=CARTESIAN_POINT('Ctrl Pts',(-17.8938116696237,9.1601561636161,18.));
#35044=CARTESIAN_POINT('Ctrl Pts',(-17.8389924349283,9.10019864472208,0.));
#35045=CARTESIAN_POINT('Ctrl Pts',(-17.8389924349283,9.10019864472208,18.));
#35046=CARTESIAN_POINT('Ctrl Pts',(-17.7836872744016,9.04090748239097,0.));
#35047=CARTESIAN_POINT('Ctrl Pts',(-17.7836872744016,9.04090748239097,18.));
#35048=CARTESIAN_POINT('Ctrl Pts',(-17.7278841963319,8.98231202490686,0.));
#35049=CARTESIAN_POINT('Ctrl Pts',(-17.7278841963319,8.98231202490686,18.));
#35050=CARTESIAN_POINT('Ctrl Pts',(-17.6715250120654,8.92451585185175,0.));
#35051=CARTESIAN_POINT('Ctrl Pts',(-17.6715250120654,8.92451585185175,18.));
#35052=CARTESIAN_POINT('Ctrl Pts',(-17.614513388992,8.86768402115344,0.));
#35053=CARTESIAN_POINT('Ctrl Pts',(-17.614513388992,8.86768402115344,18.));
#35054=CARTESIAN_POINT('Ctrl Pts',(-17.5567525798882,8.81198307239551,0.));
#35055=CARTESIAN_POINT('Ctrl Pts',(-17.5567525798882,8.81198307239551,18.));
#35056=CARTESIAN_POINT('Ctrl Pts',(-17.4981785296199,8.75752832625954,0.));
#35057=CARTESIAN_POINT('Ctrl Pts',(-17.4981785296199,8.75752832625954,18.));
#35058=CARTESIAN_POINT('Ctrl Pts',(-17.438788019753,8.70433925112174,0.));
#35059=CARTESIAN_POINT('Ctrl Pts',(-17.438788019753,8.70433925112174,18.));
#35060=CARTESIAN_POINT('Ctrl Pts',(-17.3786861166843,8.65226368112816,0.));
#35061=CARTESIAN_POINT('Ctrl Pts',(-17.3786861166843,8.65226368112816,18.));
#35062=CARTESIAN_POINT('Ctrl Pts',(-17.3180459442745,8.60104338529165,0.));
#35063=CARTESIAN_POINT('Ctrl Pts',(-17.3180459442745,8.60104338529165,18.));
#35064=CARTESIAN_POINT('Ctrl Pts',(-17.2570167183611,8.55046295192433,0.));
#35065=CARTESIAN_POINT('Ctrl Pts',(-17.2570167183611,8.55046295192433,18.));
#35066=CARTESIAN_POINT('Ctrl Pts',(-17.1956428575086,8.50048099003883,0.));
#35067=CARTESIAN_POINT('Ctrl Pts',(-17.1956428575086,8.50048099003883,18.));
#35068=CARTESIAN_POINT('Ctrl Pts',(-17.1337886602855,8.45135198307877,0.));
#35069=CARTESIAN_POINT('Ctrl Pts',(-17.1337886602855,8.45135198307877,18.));
#35070=CARTESIAN_POINT('Ctrl Pts',(-17.071033847921,8.40379607744266,0.));
#35071=CARTESIAN_POINT('Ctrl Pts',(-17.071033847921,8.40379607744266,18.));
#35072=CARTESIAN_POINT('Ctrl Pts',(-17.0067806259695,8.35882146841244,0.));
#35073=CARTESIAN_POINT('Ctrl Pts',(-17.0067806259695,8.35882146841244,18.));
#35074=CARTESIAN_POINT('Ctrl Pts',(-16.9536879065132,8.32573081382563,0.));
#35075=CARTESIAN_POINT('Ctrl Pts',(-16.9536879065132,8.32573081382563,18.));
#35076=CARTESIAN_POINT('Ctrl Pts',(-16.9126979078877,8.30290517019115,0.));
#35077=CARTESIAN_POINT('Ctrl Pts',(-16.9126979078877,8.30290517019115,18.));
#35078=CARTESIAN_POINT('Ctrl Pts',(-16.8848228151885,8.28862062120315,0.));
#35079=CARTESIAN_POINT('Ctrl Pts',(-16.8848228151885,8.28862062120315,18.));
#35080=CARTESIAN_POINT('Ctrl Pts',(-16.8707481591095,8.28171148831561,0.));
#35081=CARTESIAN_POINT('Ctrl Pts',(-16.8707481591095,8.28171148831561,18.));
#35082=CARTESIAN_POINT('',(-20.0837475345525,13.1393715591102,0.));
#35083=CARTESIAN_POINT('Ctrl Pts',(-16.8707481591095,8.28171148831561,0.));
#35084=CARTESIAN_POINT('Ctrl Pts',(-16.8848228151885,8.28862062120315,0.));
#35085=CARTESIAN_POINT('Ctrl Pts',(-16.9126979078877,8.30290517019115,0.));
#35086=CARTESIAN_POINT('Ctrl Pts',(-16.9536879065132,8.32573081382563,0.));
#35087=CARTESIAN_POINT('Ctrl Pts',(-17.0067806259695,8.35882146841244,0.));
#35088=CARTESIAN_POINT('Ctrl Pts',(-17.071033847921,8.40379607744266,0.));
#35089=CARTESIAN_POINT('Ctrl Pts',(-17.1337886602855,8.45135198307877,0.));
#35090=CARTESIAN_POINT('Ctrl Pts',(-17.1956428575086,8.50048099003883,0.));
#35091=CARTESIAN_POINT('Ctrl Pts',(-17.2570167183611,8.55046295192433,0.));
#35092=CARTESIAN_POINT('Ctrl Pts',(-17.3180459442745,8.60104338529165,0.));
#35093=CARTESIAN_POINT('Ctrl Pts',(-17.3786861166843,8.65226368112816,0.));
#35094=CARTESIAN_POINT('Ctrl Pts',(-17.438788019753,8.70433925112174,0.));
#35095=CARTESIAN_POINT('Ctrl Pts',(-17.4981785296199,8.75752832625954,0.));
#35096=CARTESIAN_POINT('Ctrl Pts',(-17.5567525798882,8.81198307239551,0.));
#35097=CARTESIAN_POINT('Ctrl Pts',(-17.614513388992,8.86768402115344,0.));
#35098=CARTESIAN_POINT('Ctrl Pts',(-17.6715250120654,8.92451585185175,0.));
#35099=CARTESIAN_POINT('Ctrl Pts',(-17.7278841963319,8.98231202490686,0.));
#35100=CARTESIAN_POINT('Ctrl Pts',(-17.7836872744016,9.04090748239097,0.));
#35101=CARTESIAN_POINT('Ctrl Pts',(-17.8389924349283,9.10019864472208,0.));
#35102=CARTESIAN_POINT('Ctrl Pts',(-17.8938116696237,9.1601561636161,0.));
#35103=CARTESIAN_POINT('Ctrl Pts',(-17.9481305624284,9.22079331175917,0.));
#35104=CARTESIAN_POINT('Ctrl Pts',(-18.0019206847747,9.28214615574471,0.));
#35105=CARTESIAN_POINT('Ctrl Pts',(-18.0551538338035,9.34425079614396,0.));
#35106=CARTESIAN_POINT('Ctrl Pts',(-18.1078184146735,9.40711718355464,0.));
#35107=CARTESIAN_POINT('Ctrl Pts',(-18.1599204445014,9.47072748065832,0.));
#35108=CARTESIAN_POINT('Ctrl Pts',(-18.2114756946126,9.53504856811685,0.));
#35109=CARTESIAN_POINT('Ctrl Pts',(-18.2625044208165,9.60004042085347,0.));
#35110=CARTESIAN_POINT('Ctrl Pts',(-18.3130254811852,9.6656654640326,0.));
#35111=CARTESIAN_POINT('Ctrl Pts',(-18.3630495772677,9.73189932619939,0.));
#35112=CARTESIAN_POINT('Ctrl Pts',(-18.4125796444662,9.79873019947434,0.));
#35113=CARTESIAN_POINT('Ctrl Pts',(-18.461614050347,9.86615372541685,0.));
#35114=CARTESIAN_POINT('Ctrl Pts',(-18.5101489409161,9.93416923996829,0.));
#35115=CARTESIAN_POINT('Ctrl Pts',(-18.5581807679204,10.0027757313807,0.));
#35116=CARTESIAN_POINT('Ctrl Pts',(-18.605709190442,10.0719672018851,0.));
#35117=CARTESIAN_POINT('Ctrl Pts',(-18.6527367592664,10.1417331637795,0.));
#35118=CARTESIAN_POINT('Ctrl Pts',(-18.699267629819,10.2120606864872,0.));
#35119=CARTESIAN_POINT('Ctrl Pts',(-18.7453065790062,10.2829359603685,0.));
#35120=CARTESIAN_POINT('Ctrl Pts',(-18.7908579693851,10.3543459451258,0.));
#35121=CARTESIAN_POINT('Ctrl Pts',(-18.8359245594214,10.4262802670211,0.));
#35122=CARTESIAN_POINT('Ctrl Pts',(-18.8805076729356,10.4987309368494,0.));
#35123=CARTESIAN_POINT('Ctrl Pts',(-18.9246077453188,10.5716914651544,0.));
#35124=CARTESIAN_POINT('Ctrl Pts',(-18.9682247574834,10.6451561585969,0.));
#35125=CARTESIAN_POINT('Ctrl Pts',(-19.0113586878152,10.7191193896586,0.));
#35126=CARTESIAN_POINT('Ctrl Pts',(-19.0540100416943,10.7935747414879,0.));
#35127=CARTESIAN_POINT('Ctrl Pts',(-19.0961797996403,10.868515097783,0.));
#35128=CARTESIAN_POINT('Ctrl Pts',(-19.1378691901023,10.9439330179206,0.));
#35129=CARTESIAN_POINT('Ctrl Pts',(-19.1790795192393,11.0198210228993,0.));
#35130=CARTESIAN_POINT('Ctrl Pts',(-19.2198119937835,11.0961718903994,0.));
#35131=CARTESIAN_POINT('Ctrl Pts',(-19.2600675167206,11.1729790050543,0.));
#35132=CARTESIAN_POINT('Ctrl Pts',(-19.2998466936739,11.2502363198588,0.));
#35133=CARTESIAN_POINT('Ctrl Pts',(-19.3391499248083,11.3279381634523,0.));
#35134=CARTESIAN_POINT('Ctrl Pts',(-19.3779774742875,11.4060790880015,0.));
#35135=CARTESIAN_POINT('Ctrl Pts',(-19.4163295466324,11.4846537135043,0.));
#35136=CARTESIAN_POINT('Ctrl Pts',(-19.4542063779876,11.5636565297382,0.));
#35137=CARTESIAN_POINT('Ctrl Pts',(-19.4916082541529,11.6430819099846,0.));
#35138=CARTESIAN_POINT('Ctrl Pts',(-19.5285354853626,11.722924244195,0.));
#35139=CARTESIAN_POINT('Ctrl Pts',(-19.5649883985826,11.8031780389346,0.));
#35140=CARTESIAN_POINT('Ctrl Pts',(-19.6009673241771,11.8838380136222,0.));
#35141=CARTESIAN_POINT('Ctrl Pts',(-19.6364725931695,11.9648992312094,0.));
#35142=CARTESIAN_POINT('Ctrl Pts',(-19.6715045149944,12.0463570680309,0.));
#35143=CARTESIAN_POINT('Ctrl Pts',(-19.7060633406705,12.1282070378972,0.));
#35144=CARTESIAN_POINT('Ctrl Pts',(-19.7401492304335,12.2104446447874,0.));
#35145=CARTESIAN_POINT('Ctrl Pts',(-19.7737622285562,12.2930652417987,0.));
#35146=CARTESIAN_POINT('Ctrl Pts',(-19.8069022248387,12.3760638341708,0.));
#35147=CARTESIAN_POINT('Ctrl Pts',(-19.839568972011,12.4594350764989,0.));
#35148=CARTESIAN_POINT('Ctrl Pts',(-19.8717621942733,12.5431736030596,0.));
#35149=CARTESIAN_POINT('Ctrl Pts',(-19.9034816813503,12.6272742843372,0.));
#35150=CARTESIAN_POINT('Ctrl Pts',(-19.9347273847264,12.7117325003719,0.));
#35151=CARTESIAN_POINT('Ctrl Pts',(-19.9654995335894,12.7965444294443,0.));
#35152=CARTESIAN_POINT('Ctrl Pts',(-20.0018585267766,12.8987398182747,0.));
#35153=CARTESIAN_POINT('Ctrl Pts',(-20.0315673466055,12.9843387891477,0.));
#35154=CARTESIAN_POINT('Ctrl Pts',(-20.054957345404,13.0530957702829,0.));
#35155=CARTESIAN_POINT('Ctrl Pts',(-20.0722879610899,13.1048196144678,0.));
#35156=CARTESIAN_POINT('Ctrl Pts',(-20.0837475345526,13.1393715591102,0.));
#35157=CARTESIAN_POINT('',(-20.0837475345525,13.1393715591102,15.));
#35158=CARTESIAN_POINT('Ctrl Pts',(-20.0837475345526,13.1393715591102,15.));
#35159=CARTESIAN_POINT('Ctrl Pts',(-20.0780177478283,13.1220955868173,15.));
#35160=CARTESIAN_POINT('Ctrl Pts',(-20.0665110891946,13.0875783330728,15.));
#35161=CARTESIAN_POINT('Ctrl Pts',(-20.0491098457044,13.0359065249991,15.));
#35162=CARTESIAN_POINT('Ctrl Pts',(-20.0256255826397,12.9672189949731,15.));
#35163=CARTESIAN_POINT('Ctrl Pts',(-19.9957986945787,12.8817072534696,15.));
#35164=CARTESIAN_POINT('Ctrl Pts',(-19.9654995335894,12.7965444294443,15.));
#35165=CARTESIAN_POINT('Ctrl Pts',(-19.9347273847264,12.7117325003719,15.));
#35166=CARTESIAN_POINT('Ctrl Pts',(-19.9034816813503,12.6272742843372,15.));
#35167=CARTESIAN_POINT('Ctrl Pts',(-19.8717621942733,12.5431736030596,15.));
#35168=CARTESIAN_POINT('Ctrl Pts',(-19.839568972011,12.4594350764989,15.));
#35169=CARTESIAN_POINT('Ctrl Pts',(-19.8069022248387,12.3760638341708,15.));
#35170=CARTESIAN_POINT('Ctrl Pts',(-19.7737622285562,12.2930652417987,15.));
#35171=CARTESIAN_POINT('Ctrl Pts',(-19.7401492304335,12.2104446447874,15.));
#35172=CARTESIAN_POINT('Ctrl Pts',(-19.7060633406705,12.1282070378972,15.));
#35173=CARTESIAN_POINT('Ctrl Pts',(-19.6715045149944,12.0463570680309,15.));
#35174=CARTESIAN_POINT('Ctrl Pts',(-19.6364725931695,11.9648992312094,15.));
#35175=CARTESIAN_POINT('Ctrl Pts',(-19.6009673241771,11.8838380136222,15.));
#35176=CARTESIAN_POINT('Ctrl Pts',(-19.5649883985826,11.8031780389346,15.));
#35177=CARTESIAN_POINT('Ctrl Pts',(-19.5285354853626,11.722924244195,15.));
#35178=CARTESIAN_POINT('Ctrl Pts',(-19.4916082541529,11.6430819099846,15.));
#35179=CARTESIAN_POINT('Ctrl Pts',(-19.4542063779876,11.5636565297382,15.));
#35180=CARTESIAN_POINT('Ctrl Pts',(-19.4163295466324,11.4846537135043,15.));
#35181=CARTESIAN_POINT('Ctrl Pts',(-19.3779774742875,11.4060790880015,15.));
#35182=CARTESIAN_POINT('Ctrl Pts',(-19.3391499248083,11.3279381634523,15.));
#35183=CARTESIAN_POINT('Ctrl Pts',(-19.2998466936739,11.2502363198588,15.));
#35184=CARTESIAN_POINT('Ctrl Pts',(-19.2600675167206,11.1729790050543,15.));
#35185=CARTESIAN_POINT('Ctrl Pts',(-19.2198119937835,11.0961718903994,15.));
#35186=CARTESIAN_POINT('Ctrl Pts',(-19.1790795192393,11.0198210228993,15.));
#35187=CARTESIAN_POINT('Ctrl Pts',(-19.1378691901023,10.9439330179206,15.));
#35188=CARTESIAN_POINT('Ctrl Pts',(-19.0961797996403,10.868515097783,15.));
#35189=CARTESIAN_POINT('Ctrl Pts',(-19.0540100416943,10.7935747414879,15.));
#35190=CARTESIAN_POINT('Ctrl Pts',(-19.0113586878152,10.7191193896586,15.));
#35191=CARTESIAN_POINT('Ctrl Pts',(-18.9682247574834,10.6451561585969,15.));
#35192=CARTESIAN_POINT('Ctrl Pts',(-18.9246077453188,10.5716914651544,15.));
#35193=CARTESIAN_POINT('Ctrl Pts',(-18.8805076729356,10.4987309368494,15.));
#35194=CARTESIAN_POINT('Ctrl Pts',(-18.8359245594214,10.4262802670211,15.));
#35195=CARTESIAN_POINT('Ctrl Pts',(-18.7908579693851,10.3543459451258,15.));
#35196=CARTESIAN_POINT('Ctrl Pts',(-18.7453065790062,10.2829359603685,15.));
#35197=CARTESIAN_POINT('Ctrl Pts',(-18.699267629819,10.2120606864872,15.));
#35198=CARTESIAN_POINT('Ctrl Pts',(-18.6527367592664,10.1417331637795,15.));
#35199=CARTESIAN_POINT('Ctrl Pts',(-18.605709190442,10.0719672018851,15.));
#35200=CARTESIAN_POINT('Ctrl Pts',(-18.5581807679204,10.0027757313807,15.));
#35201=CARTESIAN_POINT('Ctrl Pts',(-18.5101489409161,9.93416923996829,15.));
#35202=CARTESIAN_POINT('Ctrl Pts',(-18.461614050347,9.86615372541685,15.));
#35203=CARTESIAN_POINT('Ctrl Pts',(-18.4125796444662,9.79873019947434,15.));
#35204=CARTESIAN_POINT('Ctrl Pts',(-18.3630495772677,9.73189932619939,15.));
#35205=CARTESIAN_POINT('Ctrl Pts',(-18.3130254811852,9.6656654640326,15.));
#35206=CARTESIAN_POINT('Ctrl Pts',(-18.2625044208165,9.60004042085347,15.));
#35207=CARTESIAN_POINT('Ctrl Pts',(-18.2114756946126,9.53504856811685,15.));
#35208=CARTESIAN_POINT('Ctrl Pts',(-18.1599204445014,9.47072748065832,15.));
#35209=CARTESIAN_POINT('Ctrl Pts',(-18.1078184146735,9.40711718355464,15.));
#35210=CARTESIAN_POINT('Ctrl Pts',(-18.0551538338035,9.34425079614396,15.));
#35211=CARTESIAN_POINT('Ctrl Pts',(-18.0019206847747,9.28214615574471,15.));
#35212=CARTESIAN_POINT('Ctrl Pts',(-17.9481305624284,9.22079331175917,15.));
#35213=CARTESIAN_POINT('Ctrl Pts',(-17.8938116696237,9.1601561636161,15.));
#35214=CARTESIAN_POINT('Ctrl Pts',(-17.8389924349283,9.10019864472208,15.));
#35215=CARTESIAN_POINT('Ctrl Pts',(-17.7836872744016,9.04090748239097,15.));
#35216=CARTESIAN_POINT('Ctrl Pts',(-17.7278841963319,8.98231202490686,15.));
#35217=CARTESIAN_POINT('Ctrl Pts',(-17.6715250120654,8.92451585185175,15.));
#35218=CARTESIAN_POINT('Ctrl Pts',(-17.614513388992,8.86768402115344,15.));
#35219=CARTESIAN_POINT('Ctrl Pts',(-17.5567525798882,8.81198307239551,15.));
#35220=CARTESIAN_POINT('Ctrl Pts',(-17.4981785296199,8.75752832625954,15.));
#35221=CARTESIAN_POINT('Ctrl Pts',(-17.438788019753,8.70433925112174,15.));
#35222=CARTESIAN_POINT('Ctrl Pts',(-17.3786861166843,8.65226368112816,15.));
#35223=CARTESIAN_POINT('Ctrl Pts',(-17.3180459442745,8.60104338529165,15.));
#35224=CARTESIAN_POINT('Ctrl Pts',(-17.2570167183611,8.55046295192433,15.));
#35225=CARTESIAN_POINT('Ctrl Pts',(-17.1956428575086,8.50048099003883,15.));
#35226=CARTESIAN_POINT('Ctrl Pts',(-17.1337886602855,8.45135198307877,15.));
#35227=CARTESIAN_POINT('Ctrl Pts',(-17.071033847921,8.40379607744266,15.));
#35228=CARTESIAN_POINT('Ctrl Pts',(-17.0067806259695,8.35882146841244,15.));
#35229=CARTESIAN_POINT('Ctrl Pts',(-16.9536879065132,8.32573081382563,15.));
#35230=CARTESIAN_POINT('Ctrl Pts',(-16.9126979078877,8.30290517019115,15.));
#35231=CARTESIAN_POINT('Ctrl Pts',(-16.8848228151885,8.28862062120315,15.));
#35232=CARTESIAN_POINT('Ctrl Pts',(-16.8707481591095,8.28171148831561,15.));
#35233=CARTESIAN_POINT('',(-20.0837475345525,13.1393715591102,0.));
#35234=CARTESIAN_POINT('Origin',(-9.33709008296438E-14,6.79236997764462E-14,
0.));
#35235=CARTESIAN_POINT('',(-18.7025042402277,15.040489857191,0.));
#35236=CARTESIAN_POINT('Origin',(-9.33709008296438E-14,6.79236997764462E-14,
0.));
#35237=CARTESIAN_POINT('',(-18.7025042402277,15.040489857191,15.));
#35238=CARTESIAN_POINT('Origin',(-9.33709008296438E-14,6.79236997764462E-14,
15.));
#35239=CARTESIAN_POINT('',(-18.7025042402277,15.040489857191,0.));
#35240=CARTESIAN_POINT('Ctrl Pts',(-13.0897235660237,13.4858453790958,0.));
#35241=CARTESIAN_POINT('Ctrl Pts',(-13.0897235660237,13.4858453790958,18.));
#35242=CARTESIAN_POINT('Ctrl Pts',(-13.1006438497967,13.4970961329957,0.));
#35243=CARTESIAN_POINT('Ctrl Pts',(-13.1006438497967,13.4970961329957,18.));
#35244=CARTESIAN_POINT('Ctrl Pts',(-13.1228431405579,13.5191927531554,0.));
#35245=CARTESIAN_POINT('Ctrl Pts',(-13.1228431405579,13.5191927531554,18.));
#35246=CARTESIAN_POINT('Ctrl Pts',(-13.1572182238498,13.5511230466604,0.));
#35247=CARTESIAN_POINT('Ctrl Pts',(-13.1572182238498,13.5511230466604,18.));
#35248=CARTESIAN_POINT('Ctrl Pts',(-13.2050958591127,13.5913916488449,0.));
#35249=CARTESIAN_POINT('Ctrl Pts',(-13.2050958591127,13.5913916488449,18.));
#35250=CARTESIAN_POINT('Ctrl Pts',(-13.267724591625,13.6386021757691,0.));
#35251=CARTESIAN_POINT('Ctrl Pts',(-13.267724591625,13.6386021757691,18.));
#35252=CARTESIAN_POINT('Ctrl Pts',(-13.332345249068,13.6835899659728,0.));
#35253=CARTESIAN_POINT('Ctrl Pts',(-13.332345249068,13.6835899659728,18.));
#35254=CARTESIAN_POINT('Ctrl Pts',(-13.3981837093918,13.7272351052346,0.));
#35255=CARTESIAN_POINT('Ctrl Pts',(-13.3981837093918,13.7272351052346,18.));
#35256=CARTESIAN_POINT('Ctrl Pts',(-13.4646849459541,13.7701598398937,0.));
#35257=CARTESIAN_POINT('Ctrl Pts',(-13.4646849459541,13.7701598398937,18.));
#35258=CARTESIAN_POINT('Ctrl Pts',(-13.5316488646659,13.8125718693898,0.));
#35259=CARTESIAN_POINT('Ctrl Pts',(-13.5316488646659,13.8125718693898,18.));
#35260=CARTESIAN_POINT('Ctrl Pts',(-13.5991011046042,13.854416158639,0.));
#35261=CARTESIAN_POINT('Ctrl Pts',(-13.5991011046042,13.854416158639,18.));
#35262=CARTESIAN_POINT('Ctrl Pts',(-13.6672004242289,13.8954842290745,0.));
#35263=CARTESIAN_POINT('Ctrl Pts',(-13.6672004242289,13.8954842290745,18.));
#35264=CARTESIAN_POINT('Ctrl Pts',(-13.7361389175879,13.9355316323567,0.));
#35265=CARTESIAN_POINT('Ctrl Pts',(-13.7361389175879,13.9355316323567,18.));
#35266=CARTESIAN_POINT('Ctrl Pts',(-13.806028835706,13.9744114225699,0.));
#35267=CARTESIAN_POINT('Ctrl Pts',(-13.806028835706,13.9744114225699,18.));
#35268=CARTESIAN_POINT('Ctrl Pts',(-13.876852657608,14.0121326766855,0.));
#35269=CARTESIAN_POINT('Ctrl Pts',(-13.876852657608,14.0121326766855,18.));
#35270=CARTESIAN_POINT('Ctrl Pts',(-13.9485205009332,14.0487919508068,0.));
#35271=CARTESIAN_POINT('Ctrl Pts',(-13.9485205009332,14.0487919508068,18.));
#35272=CARTESIAN_POINT('Ctrl Pts',(-14.0209038736616,14.0845327205726,0.));
#35273=CARTESIAN_POINT('Ctrl Pts',(-14.0209038736616,14.0845327205726,18.));
#35274=CARTESIAN_POINT('Ctrl Pts',(-14.0938755647891,14.1194976094444,0.));
#35275=CARTESIAN_POINT('Ctrl Pts',(-14.0938755647891,14.1194976094444,18.));
#35276=CARTESIAN_POINT('Ctrl Pts',(-14.1673550455622,14.1537739659715,0.));
#35277=CARTESIAN_POINT('Ctrl Pts',(-14.1673550455622,14.1537739659715,18.));
#35278=CARTESIAN_POINT('Ctrl Pts',(-14.2413181097468,14.1873822640681,0.));
#35279=CARTESIAN_POINT('Ctrl Pts',(-14.2413181097468,14.1873822640681,18.));
#35280=CARTESIAN_POINT('Ctrl Pts',(-14.3157729256101,14.2203046917613,0.));
#35281=CARTESIAN_POINT('Ctrl Pts',(-14.3157729256101,14.2203046917613,18.));
#35282=CARTESIAN_POINT('Ctrl Pts',(-14.3907450096103,14.2525030666863,0.));
#35283=CARTESIAN_POINT('Ctrl Pts',(-14.3907450096103,14.2525030666863,18.));
#35284=CARTESIAN_POINT('Ctrl Pts',(-14.4662599802682,14.2839394106401,0.));
#35285=CARTESIAN_POINT('Ctrl Pts',(-14.4662599802682,14.2839394106401,18.));
#35286=CARTESIAN_POINT('Ctrl Pts',(-14.5423237181615,14.3145996213697,0.));
#35287=CARTESIAN_POINT('Ctrl Pts',(-14.5423237181615,14.3145996213697,18.));
#35288=CARTESIAN_POINT('Ctrl Pts',(-14.6189211183837,14.3444949335274,0.));
#35289=CARTESIAN_POINT('Ctrl Pts',(-14.6189211183837,14.3444949335274,18.));
#35290=CARTESIAN_POINT('Ctrl Pts',(-14.6960255561799,14.3736505809735,0.));
#35291=CARTESIAN_POINT('Ctrl Pts',(-14.6960255561799,14.3736505809735,18.));
#35292=CARTESIAN_POINT('Ctrl Pts',(-14.7736052248294,14.4020981965564,0.));
#35293=CARTESIAN_POINT('Ctrl Pts',(-14.7736052248294,14.4020981965564,18.));
#35294=CARTESIAN_POINT('Ctrl Pts',(-14.8516302160049,14.4298673266313,0.));
#35295=CARTESIAN_POINT('Ctrl Pts',(-14.8516302160049,14.4298673266313,18.));
#35296=CARTESIAN_POINT('Ctrl Pts',(-14.9300806580357,14.4569756801697,0.));
#35297=CARTESIAN_POINT('Ctrl Pts',(-14.9300806580357,14.4569756801697,18.));
#35298=CARTESIAN_POINT('Ctrl Pts',(-15.0089462280504,14.4834296977405,0.));
#35299=CARTESIAN_POINT('Ctrl Pts',(-15.0089462280504,14.4834296977405,18.));
#35300=CARTESIAN_POINT('Ctrl Pts',(-15.0882222764759,14.5092291736391,0.));
#35301=CARTESIAN_POINT('Ctrl Pts',(-15.0882222764759,14.5092291736391,18.));
#35302=CARTESIAN_POINT('Ctrl Pts',(-15.1679069808052,14.5343706477051,0.));
#35303=CARTESIAN_POINT('Ctrl Pts',(-15.1679069808052,14.5343706477051,18.));
#35304=CARTESIAN_POINT('Ctrl Pts',(-15.2479982823383,14.5588510579962,0.));
#35305=CARTESIAN_POINT('Ctrl Pts',(-15.2479982823383,14.5588510579962,18.));
#35306=CARTESIAN_POINT('Ctrl Pts',(-15.3284903715086,14.5826719336929,0.));
#35307=CARTESIAN_POINT('Ctrl Pts',(-15.3284903715086,14.5826719336929,18.));
#35308=CARTESIAN_POINT('Ctrl Pts',(-15.4093740621547,14.6058389416146,0.));
#35309=CARTESIAN_POINT('Ctrl Pts',(-15.4093740621547,14.6058389416146,18.));
#35310=CARTESIAN_POINT('Ctrl Pts',(-15.4906383406647,14.6283600295736,0.));
#35311=CARTESIAN_POINT('Ctrl Pts',(-15.4906383406647,14.6283600295736,18.));
#35312=CARTESIAN_POINT('Ctrl Pts',(-15.5722715494357,14.6502440080912,0.));
#35313=CARTESIAN_POINT('Ctrl Pts',(-15.5722715494357,14.6502440080912,18.));
#35314=CARTESIAN_POINT('Ctrl Pts',(-15.6542626345121,14.6714990558793,0.));
#35315=CARTESIAN_POINT('Ctrl Pts',(-15.6542626345121,14.6714990558793,18.));
#35316=CARTESIAN_POINT('Ctrl Pts',(-15.7366025822956,14.692131002056,0.));
#35317=CARTESIAN_POINT('Ctrl Pts',(-15.7366025822956,14.692131002056,18.));
#35318=CARTESIAN_POINT('Ctrl Pts',(-15.8192842036838,14.7121435744495,0.));
#35319=CARTESIAN_POINT('Ctrl Pts',(-15.8192842036838,14.7121435744495,18.));
#35320=CARTESIAN_POINT('Ctrl Pts',(-15.9023014613802,14.7315391924939,0.));
#35321=CARTESIAN_POINT('Ctrl Pts',(-15.9023014613802,14.7315391924939,18.));
#35322=CARTESIAN_POINT('Ctrl Pts',(-15.9856489347991,14.7503195973741,0.));
#35323=CARTESIAN_POINT('Ctrl Pts',(-15.9856489347991,14.7503195973741,18.));
#35324=CARTESIAN_POINT('Ctrl Pts',(-16.0693212651732,14.7684865075326,0.));
#35325=CARTESIAN_POINT('Ctrl Pts',(-16.0693212651732,14.7684865075326,18.));
#35326=CARTESIAN_POINT('Ctrl Pts',(-16.1533125058853,14.7860423865308,0.));
#35327=CARTESIAN_POINT('Ctrl Pts',(-16.1533125058853,14.7860423865308,18.));
#35328=CARTESIAN_POINT('Ctrl Pts',(-16.2376161919272,14.8029903659562,0.));
#35329=CARTESIAN_POINT('Ctrl Pts',(-16.2376161919272,14.8029903659562,18.));
#35330=CARTESIAN_POINT('Ctrl Pts',(-16.3222256264574,14.8193339134125,0.));
#35331=CARTESIAN_POINT('Ctrl Pts',(-16.3222256264574,14.8193339134125,18.));
#35332=CARTESIAN_POINT('Ctrl Pts',(-16.4071341001481,14.8350765822692,0.));
#35333=CARTESIAN_POINT('Ctrl Pts',(-16.4071341001481,14.8350765822692,18.));
#35334=CARTESIAN_POINT('Ctrl Pts',(-16.492335117066,14.8502217520165,0.));
#35335=CARTESIAN_POINT('Ctrl Pts',(-16.492335117066,14.8502217520165,18.));
#35336=CARTESIAN_POINT('Ctrl Pts',(-16.5778226646614,14.8647723257055,0.));
#35337=CARTESIAN_POINT('Ctrl Pts',(-16.5778226646614,14.8647723257055,18.));
#35338=CARTESIAN_POINT('Ctrl Pts',(-16.6635911790385,14.8787307479454,0.));
#35339=CARTESIAN_POINT('Ctrl Pts',(-16.6635911790385,14.8787307479454,18.));
#35340=CARTESIAN_POINT('Ctrl Pts',(-16.7496353900706,14.8920991518626,0.));
#35341=CARTESIAN_POINT('Ctrl Pts',(-16.7496353900706,14.8920991518626,18.));
#35342=CARTESIAN_POINT('Ctrl Pts',(-16.8359501981915,14.9048794721647,0.));
#35343=CARTESIAN_POINT('Ctrl Pts',(-16.8359501981915,14.9048794721647,18.));
#35344=CARTESIAN_POINT('Ctrl Pts',(-16.9225305499155,14.9170735658747,0.));
#35345=CARTESIAN_POINT('Ctrl Pts',(-16.9225305499155,14.9170735658747,18.));
#35346=CARTESIAN_POINT('Ctrl Pts',(-17.0093712776822,14.9286833603319,0.));
#35347=CARTESIAN_POINT('Ctrl Pts',(-17.0093712776822,14.9286833603319,18.));
#35348=CARTESIAN_POINT('Ctrl Pts',(-17.0964671184813,14.9397108660998,0.));
#35349=CARTESIAN_POINT('Ctrl Pts',(-17.0964671184813,14.9397108660998,18.));
#35350=CARTESIAN_POINT('Ctrl Pts',(-17.1838128327073,14.9501581118289,0.));
#35351=CARTESIAN_POINT('Ctrl Pts',(-17.1838128327073,14.9501581118289,18.));
#35352=CARTESIAN_POINT('Ctrl Pts',(-17.2714032968314,14.9600271060471,0.));
#35353=CARTESIAN_POINT('Ctrl Pts',(-17.2714032968314,14.9600271060471,18.));
#35354=CARTESIAN_POINT('Ctrl Pts',(-17.3592335908102,14.9693197947387,0.));
#35355=CARTESIAN_POINT('Ctrl Pts',(-17.3592335908102,14.9693197947387,18.));
#35356=CARTESIAN_POINT('Ctrl Pts',(-17.4472991215239,14.9780380183576,0.));
#35357=CARTESIAN_POINT('Ctrl Pts',(-17.4472991215239,14.9780380183576,18.));
#35358=CARTESIAN_POINT('Ctrl Pts',(-17.5355955872257,14.9861834999847,0.));
#35359=CARTESIAN_POINT('Ctrl Pts',(-17.5355955872257,14.9861834999847,18.));
#35360=CARTESIAN_POINT('Ctrl Pts',(-17.6241187988652,14.9937578646616,0.));
#35361=CARTESIAN_POINT('Ctrl Pts',(-17.6241187988652,14.9937578646616,18.));
#35362=CARTESIAN_POINT('Ctrl Pts',(-17.7128645299878,15.0007626541287,0.));
#35363=CARTESIAN_POINT('Ctrl Pts',(-17.7128645299878,15.0007626541287,18.));
#35364=CARTESIAN_POINT('Ctrl Pts',(-17.8018283748074,15.0071993464636,0.));
#35365=CARTESIAN_POINT('Ctrl Pts',(-17.8018283748074,15.0071993464636,18.));
#35366=CARTESIAN_POINT('Ctrl Pts',(-17.891005548971,15.0130693803259,0.));
#35367=CARTESIAN_POINT('Ctrl Pts',(-17.891005548971,15.0130693803259,18.));
#35368=CARTESIAN_POINT('Ctrl Pts',(-17.980390892286,15.0183741723687,0.));
#35369=CARTESIAN_POINT('Ctrl Pts',(-17.980390892286,15.0183741723687,18.));
#35370=CARTESIAN_POINT('Ctrl Pts',(-18.0699792164192,15.0231151183906,0.));
#35371=CARTESIAN_POINT('Ctrl Pts',(-18.0699792164192,15.0231151183906,18.));
#35372=CARTESIAN_POINT('Ctrl Pts',(-18.1597655779328,15.0272936035154,0.));
#35373=CARTESIAN_POINT('Ctrl Pts',(-18.1597655779328,15.0272936035154,18.));
#35374=CARTESIAN_POINT('Ctrl Pts',(-18.2497455679917,15.0309110092482,0.));
#35375=CARTESIAN_POINT('Ctrl Pts',(-18.2497455679917,15.0309110092482,18.));
#35376=CARTESIAN_POINT('Ctrl Pts',(-18.3399156227477,15.0339687345357,0.));
#35377=CARTESIAN_POINT('Ctrl Pts',(-18.3399156227477,15.0339687345357,18.));
#35378=CARTESIAN_POINT('Ctrl Pts',(-18.430273237144,15.0364681891201,0.));
#35379=CARTESIAN_POINT('Ctrl Pts',(-18.430273237144,15.0364681891201,18.));
#35380=CARTESIAN_POINT('Ctrl Pts',(-18.5208167514208,15.0384106640282,0.));
#35381=CARTESIAN_POINT('Ctrl Pts',(-18.5208167514208,15.0384106640282,18.));
#35382=CARTESIAN_POINT('Ctrl Pts',(-18.5933995108277,15.0395199113665,0.));
#35383=CARTESIAN_POINT('Ctrl Pts',(-18.5933995108277,15.0395199113665,18.));
#35384=CARTESIAN_POINT('Ctrl Pts',(-18.6479196005666,15.0401020105546,0.));
#35385=CARTESIAN_POINT('Ctrl Pts',(-18.6479196005666,15.0401020105546,18.));
#35386=CARTESIAN_POINT('Ctrl Pts',(-18.6843032127312,15.0403790752228,0.));
#35387=CARTESIAN_POINT('Ctrl Pts',(-18.6843032127312,15.0403790752228,18.));
#35388=CARTESIAN_POINT('Ctrl Pts',(-18.7025042402277,15.0404898571911,0.));
#35389=CARTESIAN_POINT('Ctrl Pts',(-18.7025042402277,15.0404898571911,18.));
#35390=CARTESIAN_POINT('Ctrl Pts',(-13.0897235660237,13.4858453790958,0.));
#35391=CARTESIAN_POINT('Ctrl Pts',(-13.1006438497967,13.4970961329957,0.));
#35392=CARTESIAN_POINT('Ctrl Pts',(-13.1228431405579,13.5191927531554,0.));
#35393=CARTESIAN_POINT('Ctrl Pts',(-13.1572182238498,13.5511230466604,0.));
#35394=CARTESIAN_POINT('Ctrl Pts',(-13.2050958591127,13.5913916488449,0.));
#35395=CARTESIAN_POINT('Ctrl Pts',(-13.267724591625,13.6386021757691,0.));
#35396=CARTESIAN_POINT('Ctrl Pts',(-13.332345249068,13.6835899659728,0.));
#35397=CARTESIAN_POINT('Ctrl Pts',(-13.3981837093918,13.7272351052346,0.));
#35398=CARTESIAN_POINT('Ctrl Pts',(-13.4646849459541,13.7701598398937,0.));
#35399=CARTESIAN_POINT('Ctrl Pts',(-13.5316488646659,13.8125718693898,0.));
#35400=CARTESIAN_POINT('Ctrl Pts',(-13.5991011046042,13.854416158639,0.));
#35401=CARTESIAN_POINT('Ctrl Pts',(-13.6672004242289,13.8954842290745,0.));
#35402=CARTESIAN_POINT('Ctrl Pts',(-13.7361389175879,13.9355316323567,0.));
#35403=CARTESIAN_POINT('Ctrl Pts',(-13.806028835706,13.9744114225699,0.));
#35404=CARTESIAN_POINT('Ctrl Pts',(-13.876852657608,14.0121326766855,0.));
#35405=CARTESIAN_POINT('Ctrl Pts',(-13.9485205009332,14.0487919508068,0.));
#35406=CARTESIAN_POINT('Ctrl Pts',(-14.0209038736616,14.0845327205726,0.));
#35407=CARTESIAN_POINT('Ctrl Pts',(-14.0938755647891,14.1194976094444,0.));
#35408=CARTESIAN_POINT('Ctrl Pts',(-14.1673550455622,14.1537739659715,0.));
#35409=CARTESIAN_POINT('Ctrl Pts',(-14.2413181097468,14.1873822640681,0.));
#35410=CARTESIAN_POINT('Ctrl Pts',(-14.3157729256101,14.2203046917613,0.));
#35411=CARTESIAN_POINT('Ctrl Pts',(-14.3907450096103,14.2525030666863,0.));
#35412=CARTESIAN_POINT('Ctrl Pts',(-14.4662599802682,14.2839394106401,0.));
#35413=CARTESIAN_POINT('Ctrl Pts',(-14.5423237181615,14.3145996213697,0.));
#35414=CARTESIAN_POINT('Ctrl Pts',(-14.6189211183837,14.3444949335274,0.));
#35415=CARTESIAN_POINT('Ctrl Pts',(-14.6960255561799,14.3736505809735,0.));
#35416=CARTESIAN_POINT('Ctrl Pts',(-14.7736052248294,14.4020981965564,0.));
#35417=CARTESIAN_POINT('Ctrl Pts',(-14.8516302160049,14.4298673266313,0.));
#35418=CARTESIAN_POINT('Ctrl Pts',(-14.9300806580357,14.4569756801697,0.));
#35419=CARTESIAN_POINT('Ctrl Pts',(-15.0089462280504,14.4834296977405,0.));
#35420=CARTESIAN_POINT('Ctrl Pts',(-15.0882222764759,14.5092291736391,0.));
#35421=CARTESIAN_POINT('Ctrl Pts',(-15.1679069808052,14.5343706477051,0.));
#35422=CARTESIAN_POINT('Ctrl Pts',(-15.2479982823383,14.5588510579962,0.));
#35423=CARTESIAN_POINT('Ctrl Pts',(-15.3284903715086,14.5826719336929,0.));
#35424=CARTESIAN_POINT('Ctrl Pts',(-15.4093740621547,14.6058389416146,0.));
#35425=CARTESIAN_POINT('Ctrl Pts',(-15.4906383406647,14.6283600295736,0.));
#35426=CARTESIAN_POINT('Ctrl Pts',(-15.5722715494357,14.6502440080912,0.));
#35427=CARTESIAN_POINT('Ctrl Pts',(-15.6542626345121,14.6714990558793,0.));
#35428=CARTESIAN_POINT('Ctrl Pts',(-15.7366025822956,14.692131002056,0.));
#35429=CARTESIAN_POINT('Ctrl Pts',(-15.8192842036838,14.7121435744495,0.));
#35430=CARTESIAN_POINT('Ctrl Pts',(-15.9023014613802,14.7315391924939,0.));
#35431=CARTESIAN_POINT('Ctrl Pts',(-15.9856489347991,14.7503195973741,0.));
#35432=CARTESIAN_POINT('Ctrl Pts',(-16.0693212651732,14.7684865075326,0.));
#35433=CARTESIAN_POINT('Ctrl Pts',(-16.1533125058853,14.7860423865308,0.));
#35434=CARTESIAN_POINT('Ctrl Pts',(-16.2376161919272,14.8029903659562,0.));
#35435=CARTESIAN_POINT('Ctrl Pts',(-16.3222256264574,14.8193339134125,0.));
#35436=CARTESIAN_POINT('Ctrl Pts',(-16.4071341001481,14.8350765822692,0.));
#35437=CARTESIAN_POINT('Ctrl Pts',(-16.492335117066,14.8502217520165,0.));
#35438=CARTESIAN_POINT('Ctrl Pts',(-16.5778226646614,14.8647723257055,0.));
#35439=CARTESIAN_POINT('Ctrl Pts',(-16.6635911790385,14.8787307479454,0.));
#35440=CARTESIAN_POINT('Ctrl Pts',(-16.7496353900706,14.8920991518626,0.));
#35441=CARTESIAN_POINT('Ctrl Pts',(-16.8359501981915,14.9048794721647,0.));
#35442=CARTESIAN_POINT('Ctrl Pts',(-16.9225305499155,14.9170735658747,0.));
#35443=CARTESIAN_POINT('Ctrl Pts',(-17.0093712776822,14.9286833603319,0.));
#35444=CARTESIAN_POINT('Ctrl Pts',(-17.0964671184813,14.9397108660998,0.));
#35445=CARTESIAN_POINT('Ctrl Pts',(-17.1838128327073,14.9501581118289,0.));
#35446=CARTESIAN_POINT('Ctrl Pts',(-17.2714032968314,14.9600271060471,0.));
#35447=CARTESIAN_POINT('Ctrl Pts',(-17.3592335908102,14.9693197947387,0.));
#35448=CARTESIAN_POINT('Ctrl Pts',(-17.4472991215239,14.9780380183576,0.));
#35449=CARTESIAN_POINT('Ctrl Pts',(-17.5355955872257,14.9861834999847,0.));
#35450=CARTESIAN_POINT('Ctrl Pts',(-17.6241187988652,14.9937578646616,0.));
#35451=CARTESIAN_POINT('Ctrl Pts',(-17.7128645299878,15.0007626541287,0.));
#35452=CARTESIAN_POINT('Ctrl Pts',(-17.8018283748074,15.0071993464636,0.));
#35453=CARTESIAN_POINT('Ctrl Pts',(-17.891005548971,15.0130693803259,0.));
#35454=CARTESIAN_POINT('Ctrl Pts',(-17.980390892286,15.0183741723687,0.));
#35455=CARTESIAN_POINT('Ctrl Pts',(-18.0699792164192,15.0231151183906,0.));
#35456=CARTESIAN_POINT('Ctrl Pts',(-18.1597655779328,15.0272936035154,0.));
#35457=CARTESIAN_POINT('Ctrl Pts',(-18.2497455679917,15.0309110092482,0.));
#35458=CARTESIAN_POINT('Ctrl Pts',(-18.3399156227477,15.0339687345357,0.));
#35459=CARTESIAN_POINT('Ctrl Pts',(-18.4483447600233,15.036968080037,0.));
#35460=CARTESIAN_POINT('Ctrl Pts',(-18.5389347492702,15.038771310026,0.));
#35461=CARTESIAN_POINT('Ctrl Pts',(-18.6115544313469,15.0397694451467,0.));
#35462=CARTESIAN_POINT('Ctrl Pts',(-18.6661021851765,15.0402682932586,0.));
#35463=CARTESIAN_POINT('Ctrl Pts',(-18.7025042402277,15.0404898571911,0.));
#35464=CARTESIAN_POINT('Ctrl Pts',(-13.0897235660237,13.4858453790958,15.));
#35465=CARTESIAN_POINT('Ctrl Pts',(-13.1006438497967,13.4970961329957,15.));
#35466=CARTESIAN_POINT('Ctrl Pts',(-13.1228431405579,13.5191927531554,15.));
#35467=CARTESIAN_POINT('Ctrl Pts',(-13.1572182238498,13.5511230466604,15.));
#35468=CARTESIAN_POINT('Ctrl Pts',(-13.2050958591127,13.5913916488449,15.));
#35469=CARTESIAN_POINT('Ctrl Pts',(-13.267724591625,13.6386021757691,15.));
#35470=CARTESIAN_POINT('Ctrl Pts',(-13.332345249068,13.6835899659728,15.));
#35471=CARTESIAN_POINT('Ctrl Pts',(-13.3981837093918,13.7272351052346,15.));
#35472=CARTESIAN_POINT('Ctrl Pts',(-13.4646849459541,13.7701598398937,15.));
#35473=CARTESIAN_POINT('Ctrl Pts',(-13.5316488646659,13.8125718693898,15.));
#35474=CARTESIAN_POINT('Ctrl Pts',(-13.5991011046042,13.854416158639,15.));
#35475=CARTESIAN_POINT('Ctrl Pts',(-13.6672004242289,13.8954842290745,15.));
#35476=CARTESIAN_POINT('Ctrl Pts',(-13.7361389175879,13.9355316323567,15.));
#35477=CARTESIAN_POINT('Ctrl Pts',(-13.806028835706,13.9744114225699,15.));
#35478=CARTESIAN_POINT('Ctrl Pts',(-13.876852657608,14.0121326766855,15.));
#35479=CARTESIAN_POINT('Ctrl Pts',(-13.9485205009332,14.0487919508068,15.));
#35480=CARTESIAN_POINT('Ctrl Pts',(-14.0209038736616,14.0845327205726,15.));
#35481=CARTESIAN_POINT('Ctrl Pts',(-14.0938755647891,14.1194976094444,15.));
#35482=CARTESIAN_POINT('Ctrl Pts',(-14.1673550455622,14.1537739659715,15.));
#35483=CARTESIAN_POINT('Ctrl Pts',(-14.2413181097468,14.1873822640681,15.));
#35484=CARTESIAN_POINT('Ctrl Pts',(-14.3157729256101,14.2203046917613,15.));
#35485=CARTESIAN_POINT('Ctrl Pts',(-14.3907450096103,14.2525030666863,15.));
#35486=CARTESIAN_POINT('Ctrl Pts',(-14.4662599802682,14.2839394106401,15.));
#35487=CARTESIAN_POINT('Ctrl Pts',(-14.5423237181615,14.3145996213697,15.));
#35488=CARTESIAN_POINT('Ctrl Pts',(-14.6189211183837,14.3444949335274,15.));
#35489=CARTESIAN_POINT('Ctrl Pts',(-14.6960255561799,14.3736505809735,15.));
#35490=CARTESIAN_POINT('Ctrl Pts',(-14.7736052248294,14.4020981965564,15.));
#35491=CARTESIAN_POINT('Ctrl Pts',(-14.8516302160049,14.4298673266313,15.));
#35492=CARTESIAN_POINT('Ctrl Pts',(-14.9300806580357,14.4569756801697,15.));
#35493=CARTESIAN_POINT('Ctrl Pts',(-15.0089462280504,14.4834296977405,15.));
#35494=CARTESIAN_POINT('Ctrl Pts',(-15.0882222764759,14.5092291736391,15.));
#35495=CARTESIAN_POINT('Ctrl Pts',(-15.1679069808052,14.5343706477051,15.));
#35496=CARTESIAN_POINT('Ctrl Pts',(-15.2479982823383,14.5588510579962,15.));
#35497=CARTESIAN_POINT('Ctrl Pts',(-15.3284903715086,14.5826719336929,15.));
#35498=CARTESIAN_POINT('Ctrl Pts',(-15.4093740621547,14.6058389416146,15.));
#35499=CARTESIAN_POINT('Ctrl Pts',(-15.4906383406647,14.6283600295736,15.));
#35500=CARTESIAN_POINT('Ctrl Pts',(-15.5722715494357,14.6502440080912,15.));
#35501=CARTESIAN_POINT('Ctrl Pts',(-15.6542626345121,14.6714990558793,15.));
#35502=CARTESIAN_POINT('Ctrl Pts',(-15.7366025822956,14.692131002056,15.));
#35503=CARTESIAN_POINT('Ctrl Pts',(-15.8192842036838,14.7121435744495,15.));
#35504=CARTESIAN_POINT('Ctrl Pts',(-15.9023014613802,14.7315391924939,15.));
#35505=CARTESIAN_POINT('Ctrl Pts',(-15.9856489347991,14.7503195973741,15.));
#35506=CARTESIAN_POINT('Ctrl Pts',(-16.0693212651732,14.7684865075326,15.));
#35507=CARTESIAN_POINT('Ctrl Pts',(-16.1533125058853,14.7860423865308,15.));
#35508=CARTESIAN_POINT('Ctrl Pts',(-16.2376161919272,14.8029903659562,15.));
#35509=CARTESIAN_POINT('Ctrl Pts',(-16.3222256264574,14.8193339134125,15.));
#35510=CARTESIAN_POINT('Ctrl Pts',(-16.4071341001481,14.8350765822692,15.));
#35511=CARTESIAN_POINT('Ctrl Pts',(-16.492335117066,14.8502217520165,15.));
#35512=CARTESIAN_POINT('Ctrl Pts',(-16.5778226646614,14.8647723257055,15.));
#35513=CARTESIAN_POINT('Ctrl Pts',(-16.6635911790385,14.8787307479454,15.));
#35514=CARTESIAN_POINT('Ctrl Pts',(-16.7496353900706,14.8920991518626,15.));
#35515=CARTESIAN_POINT('Ctrl Pts',(-16.8359501981915,14.9048794721647,15.));
#35516=CARTESIAN_POINT('Ctrl Pts',(-16.9225305499155,14.9170735658747,15.));
#35517=CARTESIAN_POINT('Ctrl Pts',(-17.0093712776822,14.9286833603319,15.));
#35518=CARTESIAN_POINT('Ctrl Pts',(-17.0964671184813,14.9397108660998,15.));
#35519=CARTESIAN_POINT('Ctrl Pts',(-17.1838128327073,14.9501581118289,15.));
#35520=CARTESIAN_POINT('Ctrl Pts',(-17.2714032968314,14.9600271060471,15.));
#35521=CARTESIAN_POINT('Ctrl Pts',(-17.3592335908102,14.9693197947387,15.));
#35522=CARTESIAN_POINT('Ctrl Pts',(-17.4472991215239,14.9780380183576,15.));
#35523=CARTESIAN_POINT('Ctrl Pts',(-17.5355955872257,14.9861834999847,15.));
#35524=CARTESIAN_POINT('Ctrl Pts',(-17.6241187988652,14.9937578646616,15.));
#35525=CARTESIAN_POINT('Ctrl Pts',(-17.7128645299878,15.0007626541287,15.));
#35526=CARTESIAN_POINT('Ctrl Pts',(-17.8018283748074,15.0071993464636,15.));
#35527=CARTESIAN_POINT('Ctrl Pts',(-17.891005548971,15.0130693803259,15.));
#35528=CARTESIAN_POINT('Ctrl Pts',(-17.980390892286,15.0183741723687,15.));
#35529=CARTESIAN_POINT('Ctrl Pts',(-18.0699792164192,15.0231151183906,15.));
#35530=CARTESIAN_POINT('Ctrl Pts',(-18.1597655779328,15.0272936035154,15.));
#35531=CARTESIAN_POINT('Ctrl Pts',(-18.2497455679917,15.0309110092482,15.));
#35532=CARTESIAN_POINT('Ctrl Pts',(-18.3399156227477,15.0339687345357,15.));
#35533=CARTESIAN_POINT('Ctrl Pts',(-18.4483447600233,15.036968080037,15.));
#35534=CARTESIAN_POINT('Ctrl Pts',(-18.5389347492702,15.038771310026,15.));
#35535=CARTESIAN_POINT('Ctrl Pts',(-18.6115544313469,15.0397694451467,15.));
#35536=CARTESIAN_POINT('Ctrl Pts',(-18.6661021851765,15.0402682932586,15.));
#35537=CARTESIAN_POINT('Ctrl Pts',(-18.7025042402277,15.0404898571911,15.));
#35538=CARTESIAN_POINT('Ctrl Pts',(-8.52496423935285,22.4349054983023,0.));
#35539=CARTESIAN_POINT('Ctrl Pts',(-8.52496423935285,22.4349054983023,18.));
#35540=CARTESIAN_POINT('Ctrl Pts',(-8.53048330625154,22.4175610589877,0.));
#35541=CARTESIAN_POINT('Ctrl Pts',(-8.53048330625154,22.4175610589877,18.));
#35542=CARTESIAN_POINT('Ctrl Pts',(-8.54146295656906,22.3828725698612,0.));
#35543=CARTESIAN_POINT('Ctrl Pts',(-8.54146295656906,22.3828725698612,18.));
#35544=CARTESIAN_POINT('Ctrl Pts',(-8.55775698160722,22.3308410047044,0.));
#35545=CARTESIAN_POINT('Ctrl Pts',(-8.55775698160722,22.3308410047044,18.));
#35546=CARTESIAN_POINT('Ctrl Pts',(-8.57913133085326,22.2614679221214,0.));
#35547=CARTESIAN_POINT('Ctrl Pts',(-8.57913133085326,22.2614679221214,18.));
#35548=CARTESIAN_POINT('Ctrl Pts',(-8.60526341207613,22.1747556651024,0.));
#35549=CARTESIAN_POINT('Ctrl Pts',(-8.60526341207613,22.1747556651024,18.));
#35550=CARTESIAN_POINT('Ctrl Pts',(-8.63080832792612,22.0880480931906,0.));
#35551=CARTESIAN_POINT('Ctrl Pts',(-8.63080832792612,22.0880480931906,18.));
#35552=CARTESIAN_POINT('Ctrl Pts',(-8.6557643376698,22.0013463859623,0.));
#35553=CARTESIAN_POINT('Ctrl Pts',(-8.6557643376698,22.0013463859623,18.));
#35554=CARTESIAN_POINT('Ctrl Pts',(-8.68012932645739,21.9146524902336,0.));
#35555=CARTESIAN_POINT('Ctrl Pts',(-8.68012932645739,21.9146524902336,18.));
#35556=CARTESIAN_POINT('Ctrl Pts',(-8.70390086252202,21.8279693631274,0.));
#35557=CARTESIAN_POINT('Ctrl Pts',(-8.70390086252202,21.8279693631274,18.));
#35558=CARTESIAN_POINT('Ctrl Pts',(-8.72707626956921,21.7413007707864,0.));
#35559=CARTESIAN_POINT('Ctrl Pts',(-8.72707626956921,21.7413007707864,18.));
#35560=CARTESIAN_POINT('Ctrl Pts',(-8.74965270266163,21.6546509866725,0.));
#35561=CARTESIAN_POINT('Ctrl Pts',(-8.74965270266163,21.6546509866725,18.));
#35562=CARTESIAN_POINT('Ctrl Pts',(-8.77162723103298,21.5680245138584,0.));
#35563=CARTESIAN_POINT('Ctrl Pts',(-8.77162723103298,21.5680245138584,18.));
#35564=CARTESIAN_POINT('Ctrl Pts',(-8.79299691277858,21.481425822209,0.));
#35565=CARTESIAN_POINT('Ctrl Pts',(-8.79299691277858,21.481425822209,18.));
#35566=CARTESIAN_POINT('Ctrl Pts',(-8.81375890120581,21.3948590173441,0.));
#35567=CARTESIAN_POINT('Ctrl Pts',(-8.81375890120581,21.3948590173441,18.));
#35568=CARTESIAN_POINT('Ctrl Pts',(-8.83391042911628,21.3083278326642,0.));
#35569=CARTESIAN_POINT('Ctrl Pts',(-8.83391042911628,21.3083278326642,18.));
#35570=CARTESIAN_POINT('Ctrl Pts',(-8.85344872418155,21.2218358113425,0.));
#35571=CARTESIAN_POINT('Ctrl Pts',(-8.85344872418155,21.2218358113425,18.));
#35572=CARTESIAN_POINT('Ctrl Pts',(-8.87237094640748,21.1353864352374,0.));
#35573=CARTESIAN_POINT('Ctrl Pts',(-8.87237094640748,21.1353864352374,18.));
#35574=CARTESIAN_POINT('Ctrl Pts',(-8.89067412773385,21.0489832630915,0.));
#35575=CARTESIAN_POINT('Ctrl Pts',(-8.89067412773385,21.0489832630915,18.));
#35576=CARTESIAN_POINT('Ctrl Pts',(-8.90835509843284,20.9626300944902,0.));
#35577=CARTESIAN_POINT('Ctrl Pts',(-8.90835509843284,20.9626300944902,18.));
#35578=CARTESIAN_POINT('Ctrl Pts',(-8.92541048738648,20.8763310073304,0.));
#35579=CARTESIAN_POINT('Ctrl Pts',(-8.92541048738648,20.8763310073304,18.));
#35580=CARTESIAN_POINT('Ctrl Pts',(-8.94183680111377,20.7900902537083,0.));
#35581=CARTESIAN_POINT('Ctrl Pts',(-8.94183680111377,20.7900902537083,18.));
#35582=CARTESIAN_POINT('Ctrl Pts',(-8.95763049112623,20.7039121898975,0.));
#35583=CARTESIAN_POINT('Ctrl Pts',(-8.95763049112623,20.7039121898975,18.));
#35584=CARTESIAN_POINT('Ctrl Pts',(-8.97278801890467,20.6178012000199,0.));
#35585=CARTESIAN_POINT('Ctrl Pts',(-8.97278801890467,20.6178012000199,18.));
#35586=CARTESIAN_POINT('Ctrl Pts',(-8.98730595457659,20.5317616031369,0.));
#35587=CARTESIAN_POINT('Ctrl Pts',(-8.98730595457659,20.5317616031369,18.));
#35588=CARTESIAN_POINT('Ctrl Pts',(-9.00118097039516,20.4457976315472,0.));
#35589=CARTESIAN_POINT('Ctrl Pts',(-9.00118097039516,20.4457976315472,18.));
#35590=CARTESIAN_POINT('Ctrl Pts',(-9.01440965049155,20.3599135373691,0.));
#35591=CARTESIAN_POINT('Ctrl Pts',(-9.01440965049155,20.3599135373691,18.));
#35592=CARTESIAN_POINT('Ctrl Pts',(-9.02698833758324,20.2741136736186,0.));
#35593=CARTESIAN_POINT('Ctrl Pts',(-9.02698833758324,20.2741136736186,18.));
#35594=CARTESIAN_POINT('Ctrl Pts',(-9.03891298737031,20.1884025764493,0.));
#35595=CARTESIAN_POINT('Ctrl Pts',(-9.03891298737031,20.1884025764493,18.));
#35596=CARTESIAN_POINT('Ctrl Pts',(-9.0501789809071,20.1027850670435,0.));
#35597=CARTESIAN_POINT('Ctrl Pts',(-9.0501789809071,20.1027850670435,18.));
#35598=CARTESIAN_POINT('Ctrl Pts',(-9.0607810967537,20.0172662790811,0.));
#35599=CARTESIAN_POINT('Ctrl Pts',(-9.0607810967537,20.0172662790811,18.));
#35600=CARTESIAN_POINT('Ctrl Pts',(-9.0707138821585,19.9318514954605,0.));
#35601=CARTESIAN_POINT('Ctrl Pts',(-9.0707138821585,19.9318514954605,18.));
#35602=CARTESIAN_POINT('Ctrl Pts',(-9.07997196979668,19.846546013708,0.));
#35603=CARTESIAN_POINT('Ctrl Pts',(-9.07997196979668,19.846546013708,18.));
#35604=CARTESIAN_POINT('Ctrl Pts',(-9.08855038355401,19.7613550146978,0.));
#35605=CARTESIAN_POINT('Ctrl Pts',(-9.08855038355401,19.7613550146978,18.));
#35606=CARTESIAN_POINT('Ctrl Pts',(-9.0964449428387,19.6762833927168,0.));
#35607=CARTESIAN_POINT('Ctrl Pts',(-9.0964449428387,19.6762833927168,18.));
#35608=CARTESIAN_POINT('Ctrl Pts',(-9.10365235736464,19.5913357132276,0.));
#35609=CARTESIAN_POINT('Ctrl Pts',(-9.10365235736464,19.5913357132276,18.));
#35610=CARTESIAN_POINT('Ctrl Pts',(-9.11016929611335,19.5065165934577,0.));
#35611=CARTESIAN_POINT('Ctrl Pts',(-9.11016929611335,19.5065165934577,18.));
#35612=CARTESIAN_POINT('Ctrl Pts',(-9.1159915924392,19.4218310275711,0.));
#35613=CARTESIAN_POINT('Ctrl Pts',(-9.1159915924392,19.4218310275711,18.));
#35614=CARTESIAN_POINT('Ctrl Pts',(-9.12111347941199,19.3372847008483,0.));
#35615=CARTESIAN_POINT('Ctrl Pts',(-9.12111347941199,19.3372847008483,18.));
#35616=CARTESIAN_POINT('Ctrl Pts',(-9.12552662785599,19.2528843844341,0.));
#35617=CARTESIAN_POINT('Ctrl Pts',(-9.12552662785599,19.2528843844341,18.));
#35618=CARTESIAN_POINT('Ctrl Pts',(-9.12921984349375,19.1686380639041,0.));
#35619=CARTESIAN_POINT('Ctrl Pts',(-9.12921984349375,19.1686380639041,18.));
#35620=CARTESIAN_POINT('Ctrl Pts',(-9.13218114462419,19.0845541036965,0.));
#35621=CARTESIAN_POINT('Ctrl Pts',(-9.13218114462419,19.0845541036965,18.));
#35622=CARTESIAN_POINT('Ctrl Pts',(-9.13439956903533,19.0006405223697,0.));
#35623=CARTESIAN_POINT('Ctrl Pts',(-9.13439956903533,19.0006405223697,18.));
#35624=CARTESIAN_POINT('Ctrl Pts',(-9.13586688858168,18.9169043053388,0.));
#35625=CARTESIAN_POINT('Ctrl Pts',(-9.13586688858168,18.9169043053388,18.));
#35626=CARTESIAN_POINT('Ctrl Pts',(-9.13657985367153,18.8333505052874,0.));
#35627=CARTESIAN_POINT('Ctrl Pts',(-9.13657985367153,18.8333505052874,18.));
#35628=CARTESIAN_POINT('Ctrl Pts',(-9.13654074021147,18.7499820263476,0.));
#35629=CARTESIAN_POINT('Ctrl Pts',(-9.13654074021147,18.7499820263476,18.));
#35630=CARTESIAN_POINT('Ctrl Pts',(-9.13575227582418,18.6668016710749,0.));
#35631=CARTESIAN_POINT('Ctrl Pts',(-9.13575227582418,18.6668016710749,18.));
#35632=CARTESIAN_POINT('Ctrl Pts',(-9.13421321934922,18.5838139250423,0.));
#35633=CARTESIAN_POINT('Ctrl Pts',(-9.13421321934922,18.5838139250423,18.));
#35634=CARTESIAN_POINT('Ctrl Pts',(-9.13191425549883,18.5010266156389,0.));
#35635=CARTESIAN_POINT('Ctrl Pts',(-9.13191425549883,18.5010266156389,18.));
#35636=CARTESIAN_POINT('Ctrl Pts',(-9.12883240135631,18.4184531695731,0.));
#35637=CARTESIAN_POINT('Ctrl Pts',(-9.12883240135631,18.4184531695731,18.));
#35638=CARTESIAN_POINT('Ctrl Pts',(-9.12493031448671,18.3361129010289,0.));
#35639=CARTESIAN_POINT('Ctrl Pts',(-9.12493031448671,18.3361129010289,18.));
#35640=CARTESIAN_POINT('Ctrl Pts',(-9.12016808144599,18.2540262849075,0.));
#35641=CARTESIAN_POINT('Ctrl Pts',(-9.12016808144599,18.2540262849075,18.));
#35642=CARTESIAN_POINT('Ctrl Pts',(-9.11451347590539,18.1722108451637,0.));
#35643=CARTESIAN_POINT('Ctrl Pts',(-9.11451347590539,18.1722108451637,18.));
#35644=CARTESIAN_POINT('Ctrl Pts',(-9.10795114540259,18.0906774757189,0.));
#35645=CARTESIAN_POINT('Ctrl Pts',(-9.10795114540259,18.0906774757189,18.));
#35646=CARTESIAN_POINT('Ctrl Pts',(-9.10049631917583,18.0094249416472,0.));
#35647=CARTESIAN_POINT('Ctrl Pts',(-9.10049631917583,18.0094249416472,18.));
#35648=CARTESIAN_POINT('Ctrl Pts',(-9.09219303320079,17.9284406141976,0.));
#35649=CARTESIAN_POINT('Ctrl Pts',(-9.09219303320079,17.9284406141976,18.));
#35650=CARTESIAN_POINT('Ctrl Pts',(-9.08308548608349,17.8477120247758,0.));
#35651=CARTESIAN_POINT('Ctrl Pts',(-9.08308548608349,17.8477120247758,18.));
#35652=CARTESIAN_POINT('Ctrl Pts',(-9.07319314215026,17.7672369091005,0.));
#35653=CARTESIAN_POINT('Ctrl Pts',(-9.07319314215026,17.7672369091005,18.));
#35654=CARTESIAN_POINT('Ctrl Pts',(-9.06248904941394,17.6870319618808,0.));
#35655=CARTESIAN_POINT('Ctrl Pts',(-9.06248904941394,17.6870319618808,18.));
#35656=CARTESIAN_POINT('Ctrl Pts',(-9.05086524971401,17.6071467783263,0.));
#35657=CARTESIAN_POINT('Ctrl Pts',(-9.05086524971401,17.6071467783263,18.));
#35658=CARTESIAN_POINT('Ctrl Pts',(-9.03814678971601,17.5276582702181,0.));
#35659=CARTESIAN_POINT('Ctrl Pts',(-9.03814678971601,17.5276582702181,18.));
#35660=CARTESIAN_POINT('Ctrl Pts',(-9.0241575097608,17.4486443043185,0.));
#35661=CARTESIAN_POINT('Ctrl Pts',(-9.0241575097608,17.4486443043185,18.));
#35662=CARTESIAN_POINT('Ctrl Pts',(-9.00877780436036,17.3701605263553,0.));
#35663=CARTESIAN_POINT('Ctrl Pts',(-9.00877780436036,17.3701605263553,18.));
#35664=CARTESIAN_POINT('Ctrl Pts',(-8.99199362652256,17.2922207948279,0.));
#35665=CARTESIAN_POINT('Ctrl Pts',(-8.99199362652256,17.2922207948279,18.));
#35666=CARTESIAN_POINT('Ctrl Pts',(-8.97397941759265,17.2147637614528,0.));
#35667=CARTESIAN_POINT('Ctrl Pts',(-8.97397941759265,17.2147637614528,18.));
#35668=CARTESIAN_POINT('Ctrl Pts',(-8.95502702208203,17.1376822726252,0.));
#35669=CARTESIAN_POINT('Ctrl Pts',(-8.95502702208203,17.1376822726252,18.));
#35670=CARTESIAN_POINT('Ctrl Pts',(-8.93538377395243,17.0608897634975,0.));
#35671=CARTESIAN_POINT('Ctrl Pts',(-8.93538377395243,17.0608897634975,18.));
#35672=CARTESIAN_POINT('Ctrl Pts',(-8.91510993758932,16.9843788566346,0.));
#35673=CARTESIAN_POINT('Ctrl Pts',(-8.91510993758932,16.9843788566346,18.));
#35674=CARTESIAN_POINT('Ctrl Pts',(-8.89394614661328,16.908275670167,0.));
#35675=CARTESIAN_POINT('Ctrl Pts',(-8.89394614661328,16.908275670167,18.));
#35676=CARTESIAN_POINT('Ctrl Pts',(-8.87112909692392,16.8329157811062,0.));
#35677=CARTESIAN_POINT('Ctrl Pts',(-8.87112909692392,16.8329157811062,18.));
#35678=CARTESIAN_POINT('Ctrl Pts',(-8.84558256033742,16.7587634618101,0.));
#35679=CARTESIAN_POINT('Ctrl Pts',(-8.84558256033742,16.7587634618101,18.));
#35680=CARTESIAN_POINT('Ctrl Pts',(-8.82207984677446,16.7007854423938,0.));
#35681=CARTESIAN_POINT('Ctrl Pts',(-8.82207984677446,16.7007854423938,18.));
#35682=CARTESIAN_POINT('Ctrl Pts',(-8.8023348179895,16.6582257921024,0.));
#35683=CARTESIAN_POINT('Ctrl Pts',(-8.8023348179895,16.6582257921024,18.));
#35684=CARTESIAN_POINT('Ctrl Pts',(-8.78817964150686,16.6302847808193,0.));
#35685=CARTESIAN_POINT('Ctrl Pts',(-8.78817964150686,16.6302847808193,18.));
#35686=CARTESIAN_POINT('Ctrl Pts',(-8.78085409196639,16.6164222996225,0.));
#35687=CARTESIAN_POINT('Ctrl Pts',(-8.78085409196639,16.6164222996225,18.));
#35688=CARTESIAN_POINT('',(-8.52496423935279,22.4349054983023,0.));
#35689=CARTESIAN_POINT('Ctrl Pts',(-8.78085409196639,16.6164222996225,0.));
#35690=CARTESIAN_POINT('Ctrl Pts',(-8.78817964150686,16.6302847808193,0.));
#35691=CARTESIAN_POINT('Ctrl Pts',(-8.8023348179895,16.6582257921024,0.));
#35692=CARTESIAN_POINT('Ctrl Pts',(-8.82207984677446,16.7007854423938,0.));
#35693=CARTESIAN_POINT('Ctrl Pts',(-8.84558256033742,16.7587634618101,0.));
#35694=CARTESIAN_POINT('Ctrl Pts',(-8.87112909692392,16.8329157811062,0.));
#35695=CARTESIAN_POINT('Ctrl Pts',(-8.89394614661328,16.908275670167,0.));
#35696=CARTESIAN_POINT('Ctrl Pts',(-8.91510993758932,16.9843788566346,0.));
#35697=CARTESIAN_POINT('Ctrl Pts',(-8.93538377395243,17.0608897634975,0.));
#35698=CARTESIAN_POINT('Ctrl Pts',(-8.95502702208203,17.1376822726252,0.));
#35699=CARTESIAN_POINT('Ctrl Pts',(-8.97397941759265,17.2147637614528,0.));
#35700=CARTESIAN_POINT('Ctrl Pts',(-8.99199362652256,17.2922207948279,0.));
#35701=CARTESIAN_POINT('Ctrl Pts',(-9.00877780436036,17.3701605263553,0.));
#35702=CARTESIAN_POINT('Ctrl Pts',(-9.0241575097608,17.4486443043185,0.));
#35703=CARTESIAN_POINT('Ctrl Pts',(-9.03814678971601,17.5276582702181,0.));
#35704=CARTESIAN_POINT('Ctrl Pts',(-9.05086524971401,17.6071467783263,0.));
#35705=CARTESIAN_POINT('Ctrl Pts',(-9.06248904941394,17.6870319618808,0.));
#35706=CARTESIAN_POINT('Ctrl Pts',(-9.07319314215026,17.7672369091005,0.));
#35707=CARTESIAN_POINT('Ctrl Pts',(-9.08308548608349,17.8477120247758,0.));
#35708=CARTESIAN_POINT('Ctrl Pts',(-9.09219303320079,17.9284406141976,0.));
#35709=CARTESIAN_POINT('Ctrl Pts',(-9.10049631917583,18.0094249416472,0.));
#35710=CARTESIAN_POINT('Ctrl Pts',(-9.10795114540259,18.0906774757189,0.));
#35711=CARTESIAN_POINT('Ctrl Pts',(-9.11451347590539,18.1722108451637,0.));
#35712=CARTESIAN_POINT('Ctrl Pts',(-9.12016808144599,18.2540262849075,0.));
#35713=CARTESIAN_POINT('Ctrl Pts',(-9.12493031448671,18.3361129010289,0.));
#35714=CARTESIAN_POINT('Ctrl Pts',(-9.12883240135631,18.4184531695731,0.));
#35715=CARTESIAN_POINT('Ctrl Pts',(-9.13191425549883,18.5010266156389,0.));
#35716=CARTESIAN_POINT('Ctrl Pts',(-9.13421321934922,18.5838139250423,0.));
#35717=CARTESIAN_POINT('Ctrl Pts',(-9.13575227582418,18.6668016710749,0.));
#35718=CARTESIAN_POINT('Ctrl Pts',(-9.13654074021147,18.7499820263476,0.));
#35719=CARTESIAN_POINT('Ctrl Pts',(-9.13657985367153,18.8333505052874,0.));
#35720=CARTESIAN_POINT('Ctrl Pts',(-9.13586688858168,18.9169043053388,0.));
#35721=CARTESIAN_POINT('Ctrl Pts',(-9.13439956903533,19.0006405223697,0.));
#35722=CARTESIAN_POINT('Ctrl Pts',(-9.13218114462419,19.0845541036965,0.));
#35723=CARTESIAN_POINT('Ctrl Pts',(-9.12921984349375,19.1686380639041,0.));
#35724=CARTESIAN_POINT('Ctrl Pts',(-9.12552662785599,19.2528843844341,0.));
#35725=CARTESIAN_POINT('Ctrl Pts',(-9.12111347941199,19.3372847008483,0.));
#35726=CARTESIAN_POINT('Ctrl Pts',(-9.1159915924392,19.4218310275711,0.));
#35727=CARTESIAN_POINT('Ctrl Pts',(-9.11016929611335,19.5065165934577,0.));
#35728=CARTESIAN_POINT('Ctrl Pts',(-9.10365235736464,19.5913357132276,0.));
#35729=CARTESIAN_POINT('Ctrl Pts',(-9.0964449428387,19.6762833927168,0.));
#35730=CARTESIAN_POINT('Ctrl Pts',(-9.08855038355401,19.7613550146978,0.));
#35731=CARTESIAN_POINT('Ctrl Pts',(-9.07997196979668,19.846546013708,0.));
#35732=CARTESIAN_POINT('Ctrl Pts',(-9.0707138821585,19.9318514954605,0.));
#35733=CARTESIAN_POINT('Ctrl Pts',(-9.0607810967537,20.0172662790811,0.));
#35734=CARTESIAN_POINT('Ctrl Pts',(-9.0501789809071,20.1027850670435,0.));
#35735=CARTESIAN_POINT('Ctrl Pts',(-9.03891298737031,20.1884025764493,0.));
#35736=CARTESIAN_POINT('Ctrl Pts',(-9.02698833758324,20.2741136736186,0.));
#35737=CARTESIAN_POINT('Ctrl Pts',(-9.01440965049155,20.3599135373691,0.));
#35738=CARTESIAN_POINT('Ctrl Pts',(-9.00118097039516,20.4457976315472,0.));
#35739=CARTESIAN_POINT('Ctrl Pts',(-8.98730595457659,20.5317616031369,0.));
#35740=CARTESIAN_POINT('Ctrl Pts',(-8.97278801890467,20.6178012000199,0.));
#35741=CARTESIAN_POINT('Ctrl Pts',(-8.95763049112623,20.7039121898975,0.));
#35742=CARTESIAN_POINT('Ctrl Pts',(-8.94183680111377,20.7900902537083,0.));
#35743=CARTESIAN_POINT('Ctrl Pts',(-8.92541048738648,20.8763310073304,0.));
#35744=CARTESIAN_POINT('Ctrl Pts',(-8.90835509843284,20.9626300944902,0.));
#35745=CARTESIAN_POINT('Ctrl Pts',(-8.89067412773385,21.0489832630915,0.));
#35746=CARTESIAN_POINT('Ctrl Pts',(-8.87237094640748,21.1353864352374,0.));
#35747=CARTESIAN_POINT('Ctrl Pts',(-8.85344872418155,21.2218358113425,0.));
#35748=CARTESIAN_POINT('Ctrl Pts',(-8.83391042911628,21.3083278326642,0.));
#35749=CARTESIAN_POINT('Ctrl Pts',(-8.81375890120581,21.3948590173441,0.));
#35750=CARTESIAN_POINT('Ctrl Pts',(-8.79299691277858,21.481425822209,0.));
#35751=CARTESIAN_POINT('Ctrl Pts',(-8.77162723103298,21.5680245138584,0.));
#35752=CARTESIAN_POINT('Ctrl Pts',(-8.74965270266163,21.6546509866725,0.));
#35753=CARTESIAN_POINT('Ctrl Pts',(-8.72707626956921,21.7413007707864,0.));
#35754=CARTESIAN_POINT('Ctrl Pts',(-8.70390086252202,21.8279693631274,0.));
#35755=CARTESIAN_POINT('Ctrl Pts',(-8.68012932645739,21.9146524902336,0.));
#35756=CARTESIAN_POINT('Ctrl Pts',(-8.6557643376698,22.0013463859623,0.));
#35757=CARTESIAN_POINT('Ctrl Pts',(-8.63080832792612,22.0880480931906,0.));
#35758=CARTESIAN_POINT('Ctrl Pts',(-8.60015442890613,22.1920971794848,0.));
#35759=CARTESIAN_POINT('Ctrl Pts',(-8.57387555634004,22.2788106077806,0.));
#35760=CARTESIAN_POINT('Ctrl Pts',(-8.55238412336295,22.3481844703457,0.));
#35761=CARTESIAN_POINT('Ctrl Pts',(-8.53600237317212,22.400216619619,0.));
#35762=CARTESIAN_POINT('Ctrl Pts',(-8.52496423935285,22.4349054983023,0.));
#35763=CARTESIAN_POINT('',(-8.52496423935279,22.4349054983023,15.));
#35764=CARTESIAN_POINT('Ctrl Pts',(-8.52496423935285,22.4349054983023,15.));
#35765=CARTESIAN_POINT('Ctrl Pts',(-8.53048330625154,22.4175610589877,15.));
#35766=CARTESIAN_POINT('Ctrl Pts',(-8.54146295656906,22.3828725698612,15.));
#35767=CARTESIAN_POINT('Ctrl Pts',(-8.55775698160722,22.3308410047044,15.));
#35768=CARTESIAN_POINT('Ctrl Pts',(-8.57913133085326,22.2614679221214,15.));
#35769=CARTESIAN_POINT('Ctrl Pts',(-8.60526341207613,22.1747556651024,15.));
#35770=CARTESIAN_POINT('Ctrl Pts',(-8.63080832792612,22.0880480931906,15.));
#35771=CARTESIAN_POINT('Ctrl Pts',(-8.6557643376698,22.0013463859623,15.));
#35772=CARTESIAN_POINT('Ctrl Pts',(-8.68012932645739,21.9146524902336,15.));
#35773=CARTESIAN_POINT('Ctrl Pts',(-8.70390086252202,21.8279693631274,15.));
#35774=CARTESIAN_POINT('Ctrl Pts',(-8.72707626956921,21.7413007707864,15.));
#35775=CARTESIAN_POINT('Ctrl Pts',(-8.74965270266163,21.6546509866725,15.));
#35776=CARTESIAN_POINT('Ctrl Pts',(-8.77162723103298,21.5680245138584,15.));
#35777=CARTESIAN_POINT('Ctrl Pts',(-8.79299691277858,21.481425822209,15.));
#35778=CARTESIAN_POINT('Ctrl Pts',(-8.81375890120581,21.3948590173441,15.));
#35779=CARTESIAN_POINT('Ctrl Pts',(-8.83391042911628,21.3083278326642,15.));
#35780=CARTESIAN_POINT('Ctrl Pts',(-8.85344872418155,21.2218358113425,15.));
#35781=CARTESIAN_POINT('Ctrl Pts',(-8.87237094640748,21.1353864352374,15.));
#35782=CARTESIAN_POINT('Ctrl Pts',(-8.89067412773385,21.0489832630915,15.));
#35783=CARTESIAN_POINT('Ctrl Pts',(-8.90835509843284,20.9626300944902,15.));
#35784=CARTESIAN_POINT('Ctrl Pts',(-8.92541048738648,20.8763310073304,15.));
#35785=CARTESIAN_POINT('Ctrl Pts',(-8.94183680111377,20.7900902537083,15.));
#35786=CARTESIAN_POINT('Ctrl Pts',(-8.95763049112623,20.7039121898975,15.));
#35787=CARTESIAN_POINT('Ctrl Pts',(-8.97278801890467,20.6178012000199,15.));
#35788=CARTESIAN_POINT('Ctrl Pts',(-8.98730595457659,20.5317616031369,15.));
#35789=CARTESIAN_POINT('Ctrl Pts',(-9.00118097039516,20.4457976315472,15.));
#35790=CARTESIAN_POINT('Ctrl Pts',(-9.01440965049155,20.3599135373691,15.));
#35791=CARTESIAN_POINT('Ctrl Pts',(-9.02698833758324,20.2741136736186,15.));
#35792=CARTESIAN_POINT('Ctrl Pts',(-9.03891298737031,20.1884025764493,15.));
#35793=CARTESIAN_POINT('Ctrl Pts',(-9.0501789809071,20.1027850670435,15.));
#35794=CARTESIAN_POINT('Ctrl Pts',(-9.0607810967537,20.0172662790811,15.));
#35795=CARTESIAN_POINT('Ctrl Pts',(-9.0707138821585,19.9318514954605,15.));
#35796=CARTESIAN_POINT('Ctrl Pts',(-9.07997196979668,19.846546013708,15.));
#35797=CARTESIAN_POINT('Ctrl Pts',(-9.08855038355401,19.7613550146978,15.));
#35798=CARTESIAN_POINT('Ctrl Pts',(-9.0964449428387,19.6762833927168,15.));
#35799=CARTESIAN_POINT('Ctrl Pts',(-9.10365235736464,19.5913357132276,15.));
#35800=CARTESIAN_POINT('Ctrl Pts',(-9.11016929611335,19.5065165934577,15.));
#35801=CARTESIAN_POINT('Ctrl Pts',(-9.1159915924392,19.4218310275711,15.));
#35802=CARTESIAN_POINT('Ctrl Pts',(-9.12111347941199,19.3372847008483,15.));
#35803=CARTESIAN_POINT('Ctrl Pts',(-9.12552662785599,19.2528843844341,15.));
#35804=CARTESIAN_POINT('Ctrl Pts',(-9.12921984349375,19.1686380639041,15.));
#35805=CARTESIAN_POINT('Ctrl Pts',(-9.13218114462419,19.0845541036965,15.));
#35806=CARTESIAN_POINT('Ctrl Pts',(-9.13439956903533,19.0006405223697,15.));
#35807=CARTESIAN_POINT('Ctrl Pts',(-9.13586688858168,18.9169043053388,15.));
#35808=CARTESIAN_POINT('Ctrl Pts',(-9.13657985367153,18.8333505052874,15.));
#35809=CARTESIAN_POINT('Ctrl Pts',(-9.13654074021147,18.7499820263476,15.));
#35810=CARTESIAN_POINT('Ctrl Pts',(-9.13575227582418,18.6668016710749,15.));
#35811=CARTESIAN_POINT('Ctrl Pts',(-9.13421321934922,18.5838139250423,15.));
#35812=CARTESIAN_POINT('Ctrl Pts',(-9.13191425549883,18.5010266156389,15.));
#35813=CARTESIAN_POINT('Ctrl Pts',(-9.12883240135631,18.4184531695731,15.));
#35814=CARTESIAN_POINT('Ctrl Pts',(-9.12493031448671,18.3361129010289,15.));
#35815=CARTESIAN_POINT('Ctrl Pts',(-9.12016808144599,18.2540262849075,15.));
#35816=CARTESIAN_POINT('Ctrl Pts',(-9.11451347590539,18.1722108451637,15.));
#35817=CARTESIAN_POINT('Ctrl Pts',(-9.10795114540259,18.0906774757189,15.));
#35818=CARTESIAN_POINT('Ctrl Pts',(-9.10049631917583,18.0094249416472,15.));
#35819=CARTESIAN_POINT('Ctrl Pts',(-9.09219303320079,17.9284406141976,15.));
#35820=CARTESIAN_POINT('Ctrl Pts',(-9.08308548608349,17.8477120247758,15.));
#35821=CARTESIAN_POINT('Ctrl Pts',(-9.07319314215026,17.7672369091005,15.));
#35822=CARTESIAN_POINT('Ctrl Pts',(-9.06248904941394,17.6870319618808,15.));
#35823=CARTESIAN_POINT('Ctrl Pts',(-9.05086524971401,17.6071467783263,15.));
#35824=CARTESIAN_POINT('Ctrl Pts',(-9.03814678971601,17.5276582702181,15.));
#35825=CARTESIAN_POINT('Ctrl Pts',(-9.0241575097608,17.4486443043185,15.));
#35826=CARTESIAN_POINT('Ctrl Pts',(-9.00877780436036,17.3701605263553,15.));
#35827=CARTESIAN_POINT('Ctrl Pts',(-8.99199362652256,17.2922207948279,15.));
#35828=CARTESIAN_POINT('Ctrl Pts',(-8.97397941759265,17.2147637614528,15.));
#35829=CARTESIAN_POINT('Ctrl Pts',(-8.95502702208203,17.1376822726252,15.));
#35830=CARTESIAN_POINT('Ctrl Pts',(-8.93538377395243,17.0608897634975,15.));
#35831=CARTESIAN_POINT('Ctrl Pts',(-8.91510993758932,16.9843788566346,15.));
#35832=CARTESIAN_POINT('Ctrl Pts',(-8.89394614661328,16.908275670167,15.));
#35833=CARTESIAN_POINT('Ctrl Pts',(-8.87112909692392,16.8329157811062,15.));
#35834=CARTESIAN_POINT('Ctrl Pts',(-8.84558256033742,16.7587634618101,15.));
#35835=CARTESIAN_POINT('Ctrl Pts',(-8.82207984677446,16.7007854423938,15.));
#35836=CARTESIAN_POINT('Ctrl Pts',(-8.8023348179895,16.6582257921024,15.));
#35837=CARTESIAN_POINT('Ctrl Pts',(-8.78817964150686,16.6302847808193,15.));
#35838=CARTESIAN_POINT('Ctrl Pts',(-8.78085409196639,16.6164222996225,15.));
#35839=CARTESIAN_POINT('',(-8.52496423935279,22.4349054983023,0.));
#35840=CARTESIAN_POINT('Origin',(-3.56140965415431E-14,1.09833465940894E-13,
0.));
#35841=CARTESIAN_POINT('',(-6.29006564240226,23.1610680715348,0.));
#35842=CARTESIAN_POINT('Origin',(-3.56140965415431E-14,1.09833465940894E-13,
0.));
#35843=CARTESIAN_POINT('',(-6.29006564240226,23.1610680715348,15.));
#35844=CARTESIAN_POINT('Origin',(-3.56140965415431E-14,1.09833465940894E-13,
15.));
#35845=CARTESIAN_POINT('',(-6.29006564240226,23.1610680715348,0.));
#35846=CARTESIAN_POINT('Ctrl Pts',(-2.66302778805429,18.6042245638953,0.));
#35847=CARTESIAN_POINT('Ctrl Pts',(-2.66302778805429,18.6042245638953,18.));
#35848=CARTESIAN_POINT('Ctrl Pts',(-2.66524945599054,18.6197453967525,0.));
#35849=CARTESIAN_POINT('Ctrl Pts',(-2.66524945599054,18.6197453967525,18.));
#35850=CARTESIAN_POINT('Ctrl Pts',(-2.67022099202408,18.6506703537007,0.));
#35851=CARTESIAN_POINT('Ctrl Pts',(-2.67022099202408,18.6506703537007,18.));
#35852=CARTESIAN_POINT('Ctrl Pts',(-2.67926286296661,18.696707670787,0.));
#35853=CARTESIAN_POINT('Ctrl Pts',(-2.67926286296661,18.696707670787,18.));
#35854=CARTESIAN_POINT('Ctrl Pts',(-2.69432739305027,18.7574274222161,0.));
#35855=CARTESIAN_POINT('Ctrl Pts',(-2.69432739305027,18.7574274222161,18.));
#35856=CARTESIAN_POINT('Ctrl Pts',(-2.71724545050994,18.8324337861517,0.));
#35857=CARTESIAN_POINT('Ctrl Pts',(-2.71724545050994,18.8324337861517,18.));
#35858=CARTESIAN_POINT('Ctrl Pts',(-2.74308150095404,18.9068127424043,0.));
#35859=CARTESIAN_POINT('Ctrl Pts',(-2.74308150095404,18.9068127424043,18.));
#35860=CARTESIAN_POINT('Ctrl Pts',(-2.77069196504715,18.980821277801,0.));
#35861=CARTESIAN_POINT('Ctrl Pts',(-2.77069196504715,18.980821277801,18.));
#35862=CARTESIAN_POINT('Ctrl Pts',(-2.79926206958176,19.0546365637297,0.));
#35863=CARTESIAN_POINT('Ctrl Pts',(-2.79926206958176,19.0546365637297,18.));
#35864=CARTESIAN_POINT('Ctrl Pts',(-2.828507852372,19.1283090202125,0.));
#35865=CARTESIAN_POINT('Ctrl Pts',(-2.828507852372,19.1283090202125,18.));
#35866=CARTESIAN_POINT('Ctrl Pts',(-2.85848240467741,19.2018091932025,0.));
#35867=CARTESIAN_POINT('Ctrl Pts',(-2.85848240467741,19.2018091932025,18.));
#35868=CARTESIAN_POINT('Ctrl Pts',(-2.88943670541708,19.2750617358775,0.));
#35869=CARTESIAN_POINT('Ctrl Pts',(-2.88943670541708,19.2750617358775,18.));
#35870=CARTESIAN_POINT('Ctrl Pts',(-2.92166984506916,19.3479817954251,0.));
#35871=CARTESIAN_POINT('Ctrl Pts',(-2.92166984506916,19.3479817954251,18.));
#35872=CARTESIAN_POINT('Ctrl Pts',(-2.95535900926266,19.420516469599,0.));
#35873=CARTESIAN_POINT('Ctrl Pts',(-2.95535900926266,19.420516469599,18.));
#35874=CARTESIAN_POINT('Ctrl Pts',(-2.99048468792079,19.4926628032527,0.));
#35875=CARTESIAN_POINT('Ctrl Pts',(-2.99048468792079,19.4926628032527,18.));
#35876=CARTESIAN_POINT('Ctrl Pts',(-3.02691741043284,19.5644460803884,0.));
#35877=CARTESIAN_POINT('Ctrl Pts',(-3.02691741043284,19.5644460803884,18.));
#35878=CARTESIAN_POINT('Ctrl Pts',(-3.06446889170638,19.635906849522,0.));
#35879=CARTESIAN_POINT('Ctrl Pts',(-3.06446889170638,19.635906849522,18.));
#35880=CARTESIAN_POINT('Ctrl Pts',(-3.10295238390997,19.7070857227052,0.));
#35881=CARTESIAN_POINT('Ctrl Pts',(-3.10295238390997,19.7070857227052,18.));
#35882=CARTESIAN_POINT('Ctrl Pts',(-3.1422513957243,19.7780060327854,0.));
#35883=CARTESIAN_POINT('Ctrl Pts',(-3.1422513957243,19.7780060327854,18.));
#35884=CARTESIAN_POINT('Ctrl Pts',(-3.18233430962982,19.8486701154397,0.));
#35885=CARTESIAN_POINT('Ctrl Pts',(-3.18233430962982,19.8486701154397,18.));
#35886=CARTESIAN_POINT('Ctrl Pts',(-3.22321820350857,19.9190683616661,0.));
#35887=CARTESIAN_POINT('Ctrl Pts',(-3.22321820350857,19.9190683616661,18.));
#35888=CARTESIAN_POINT('Ctrl Pts',(-3.26494616363974,19.9891848794807,0.));
#35889=CARTESIAN_POINT('Ctrl Pts',(-3.26494616363974,19.9891848794807,18.));
#35890=CARTESIAN_POINT('Ctrl Pts',(-3.30756123886962,20.0590040020603,0.));
#35891=CARTESIAN_POINT('Ctrl Pts',(-3.30756123886962,20.0590040020603,18.));
#35892=CARTESIAN_POINT('Ctrl Pts',(-3.351076475782,20.1285177769596,0.));
#35893=CARTESIAN_POINT('Ctrl Pts',(-3.351076475782,20.1285177769596,18.));
#35894=CARTESIAN_POINT('Ctrl Pts',(-3.39547305068767,20.1977264147619,0.));
#35895=CARTESIAN_POINT('Ctrl Pts',(-3.39547305068767,20.1977264147619,18.));
#35896=CARTESIAN_POINT('Ctrl Pts',(-3.44071459161672,20.2666346804507,0.));
#35897=CARTESIAN_POINT('Ctrl Pts',(-3.44071459161672,20.2666346804507,18.));
#35898=CARTESIAN_POINT('Ctrl Pts',(-3.48675677306966,20.3352494700167,0.));
#35899=CARTESIAN_POINT('Ctrl Pts',(-3.48675677306966,20.3352494700167,18.));
#35900=CARTESIAN_POINT('Ctrl Pts',(-3.53355803178954,20.4035771072894,0.));
#35901=CARTESIAN_POINT('Ctrl Pts',(-3.53355803178954,20.4035771072894,18.));
#35902=CARTESIAN_POINT('Ctrl Pts',(-3.58109188218494,20.4716202388531,0.));
#35903=CARTESIAN_POINT('Ctrl Pts',(-3.58109188218494,20.4716202388531,18.));
#35904=CARTESIAN_POINT('Ctrl Pts',(-3.62934618720589,20.5393780076056,0.));
#35905=CARTESIAN_POINT('Ctrl Pts',(-3.62934618720589,20.5393780076056,18.));
#35906=CARTESIAN_POINT('Ctrl Pts',(-3.67831730617887,20.6068475141781,0.));
#35907=CARTESIAN_POINT('Ctrl Pts',(-3.67831730617887,20.6068475141781,18.));
#35908=CARTESIAN_POINT('Ctrl Pts',(-3.72800579849619,20.6740248879992,0.));
#35909=CARTESIAN_POINT('Ctrl Pts',(-3.72800579849619,20.6740248879992,18.));
#35910=CARTESIAN_POINT('Ctrl Pts',(-3.77841179839888,20.740906441832,0.));
#35911=CARTESIAN_POINT('Ctrl Pts',(-3.77841179839888,20.740906441832,18.));
#35912=CARTESIAN_POINT('Ctrl Pts',(-3.82952970701915,20.8074899980321,0.));
#35913=CARTESIAN_POINT('Ctrl Pts',(-3.82952970701915,20.8074899980321,18.));
#35914=CARTESIAN_POINT('Ctrl Pts',(-3.88134876172354,20.8737747416623,0.));
#35915=CARTESIAN_POINT('Ctrl Pts',(-3.88134876172354,20.8737747416623,18.));
#35916=CARTESIAN_POINT('Ctrl Pts',(-3.93385538070582,20.9397606289993,0.));
#35917=CARTESIAN_POINT('Ctrl Pts',(-3.93385538070582,20.9397606289993,18.));
#35918=CARTESIAN_POINT('Ctrl Pts',(-3.98703495407281,21.0054479357374,0.));
#35919=CARTESIAN_POINT('Ctrl Pts',(-3.98703495407281,21.0054479357374,18.));
#35920=CARTESIAN_POINT('Ctrl Pts',(-4.04087373166023,21.0708367812416,0.));
#35921=CARTESIAN_POINT('Ctrl Pts',(-4.04087373166023,21.0708367812416,18.));
#35922=CARTESIAN_POINT('Ctrl Pts',(-4.09536099504429,21.1359265833073,0.));
#35923=CARTESIAN_POINT('Ctrl Pts',(-4.09536099504429,21.1359265833073,18.));
#35924=CARTESIAN_POINT('Ctrl Pts',(-4.15048873695645,21.2007161321625,0.));
#35925=CARTESIAN_POINT('Ctrl Pts',(-4.15048873695645,21.2007161321625,18.));
#35926=CARTESIAN_POINT('Ctrl Pts',(-4.20625065101369,21.2652038365365,0.));
#35927=CARTESIAN_POINT('Ctrl Pts',(-4.20625065101369,21.2652038365365,18.));
#35928=CARTESIAN_POINT('Ctrl Pts',(-4.26264132842711,21.3293879189372,0.));
#35929=CARTESIAN_POINT('Ctrl Pts',(-4.26264132842711,21.3293879189372,18.));
#35930=CARTESIAN_POINT('Ctrl Pts',(-4.31965542378783,21.3932666198096,0.));
#35931=CARTESIAN_POINT('Ctrl Pts',(-4.31965542378783,21.3932666198096,18.));
#35932=CARTESIAN_POINT('Ctrl Pts',(-4.37728667813637,21.4568384368826,0.));
#35933=CARTESIAN_POINT('Ctrl Pts',(-4.37728667813637,21.4568384368826,18.));
#35934=CARTESIAN_POINT('Ctrl Pts',(-4.43552802047029,21.5201021036274,0.));
#35935=CARTESIAN_POINT('Ctrl Pts',(-4.43552802047029,21.5201021036274,18.));
#35936=CARTESIAN_POINT('Ctrl Pts',(-4.49437199472474,21.5830564890896,0.));
#35937=CARTESIAN_POINT('Ctrl Pts',(-4.49437199472474,21.5830564890896,18.));
#35938=CARTESIAN_POINT('Ctrl Pts',(-4.55381108432127,21.6457005243617,0.));
#35939=CARTESIAN_POINT('Ctrl Pts',(-4.55381108432127,21.6457005243617,18.));
#35940=CARTESIAN_POINT('Ctrl Pts',(-4.6138380475249,21.7080331252945,0.));
#35941=CARTESIAN_POINT('Ctrl Pts',(-4.6138380475249,21.7080331252945,18.));
#35942=CARTESIAN_POINT('Ctrl Pts',(-4.67444631371023,21.770053106418,0.));
#35943=CARTESIAN_POINT('Ctrl Pts',(-4.67444631371023,21.770053106418,18.));
#35944=CARTESIAN_POINT('Ctrl Pts',(-4.73562994468575,21.8317591750867,0.));
#35945=CARTESIAN_POINT('Ctrl Pts',(-4.73562994468575,21.8317591750867,18.));
#35946=CARTESIAN_POINT('Ctrl Pts',(-4.7973834230091,21.8931499593332,0.));
#35947=CARTESIAN_POINT('Ctrl Pts',(-4.7973834230091,21.8931499593332,18.));
#35948=CARTESIAN_POINT('Ctrl Pts',(-4.85970148585195,21.954224026919,0.));
#35949=CARTESIAN_POINT('Ctrl Pts',(-4.85970148585195,21.954224026919,18.));
#35950=CARTESIAN_POINT('Ctrl Pts',(-4.92257895332779,22.0149799098431,0.));
#35951=CARTESIAN_POINT('Ctrl Pts',(-4.92257895332779,22.0149799098431,18.));
#35952=CARTESIAN_POINT('Ctrl Pts',(-4.98601051193086,22.0754161299398,0.));
#35953=CARTESIAN_POINT('Ctrl Pts',(-4.98601051193086,22.0754161299398,18.));
#35954=CARTESIAN_POINT('Ctrl Pts',(-5.04999072201681,22.1355312202693,0.));
#35955=CARTESIAN_POINT('Ctrl Pts',(-5.04999072201681,22.1355312202693,18.));
#35956=CARTESIAN_POINT('Ctrl Pts',(-5.11451415224483,22.1953237422816,0.));
#35957=CARTESIAN_POINT('Ctrl Pts',(-5.11451415224483,22.1953237422816,18.));
#35958=CARTESIAN_POINT('Ctrl Pts',(-5.17957547700992,22.2547923093751,0.));
#35959=CARTESIAN_POINT('Ctrl Pts',(-5.17957547700992,22.2547923093751,18.));
#35960=CARTESIAN_POINT('Ctrl Pts',(-5.24516957209272,22.3139356039553,0.));
#35961=CARTESIAN_POINT('Ctrl Pts',(-5.24516957209272,22.3139356039553,18.));
#35962=CARTESIAN_POINT('Ctrl Pts',(-5.31129163978934,22.3727524152125,0.));
#35963=CARTESIAN_POINT('Ctrl Pts',(-5.31129163978934,22.3727524152125,18.));
#35964=CARTESIAN_POINT('Ctrl Pts',(-5.37793718711213,22.4312416086453,0.));
#35965=CARTESIAN_POINT('Ctrl Pts',(-5.37793718711213,22.4312416086453,18.));
#35966=CARTESIAN_POINT('Ctrl Pts',(-5.44510186987254,22.4894020366778,0.));
#35967=CARTESIAN_POINT('Ctrl Pts',(-5.44510186987254,22.4894020366778,18.));
#35968=CARTESIAN_POINT('Ctrl Pts',(-5.51278136258486,22.5472324623564,0.));
#35969=CARTESIAN_POINT('Ctrl Pts',(-5.51278136258486,22.5472324623564,18.));
#35970=CARTESIAN_POINT('Ctrl Pts',(-5.58097123210075,22.6047314918151,0.));
#35971=CARTESIAN_POINT('Ctrl Pts',(-5.58097123210075,22.6047314918151,18.));
#35972=CARTESIAN_POINT('Ctrl Pts',(-5.64966676217478,22.6618974767817,0.));
#35973=CARTESIAN_POINT('Ctrl Pts',(-5.64966676217478,22.6618974767817,18.));
#35974=CARTESIAN_POINT('Ctrl Pts',(-5.71886294543539,22.7187285302677,0.));
#35975=CARTESIAN_POINT('Ctrl Pts',(-5.71886294543539,22.7187285302677,18.));
#35976=CARTESIAN_POINT('Ctrl Pts',(-5.7885547640031,22.7752227318719,0.));
#35977=CARTESIAN_POINT('Ctrl Pts',(-5.7885547640031,22.7752227318719,18.));
#35978=CARTESIAN_POINT('Ctrl Pts',(-5.85873740439746,22.8313782965033,0.));
#35979=CARTESIAN_POINT('Ctrl Pts',(-5.85873740439746,22.8313782965033,18.));
#35980=CARTESIAN_POINT('Ctrl Pts',(-5.92940648776744,22.8871937503747,0.));
#35981=CARTESIAN_POINT('Ctrl Pts',(-5.92940648776744,22.8871937503747,18.));
#35982=CARTESIAN_POINT('Ctrl Pts',(-6.00055830861927,22.9426681304804,0.));
#35983=CARTESIAN_POINT('Ctrl Pts',(-6.00055830861927,22.9426681304804,18.));
#35984=CARTESIAN_POINT('Ctrl Pts',(-6.07219001169363,22.9978011048904,0.));
#35985=CARTESIAN_POINT('Ctrl Pts',(-6.07219001169363,22.9978011048904,18.));
#35986=CARTESIAN_POINT('Ctrl Pts',(-6.14429949537005,23.0525927424848,0.));
#35987=CARTESIAN_POINT('Ctrl Pts',(-6.14429949537005,23.0525927424848,18.));
#35988=CARTESIAN_POINT('Ctrl Pts',(-6.20236818200218,23.0961532179825,0.));
#35989=CARTESIAN_POINT('Ctrl Pts',(-6.20236818200218,23.0961532179825,18.));
#35990=CARTESIAN_POINT('Ctrl Pts',(-6.24613371181767,23.1286702508203,0.));
#35991=CARTESIAN_POINT('Ctrl Pts',(-6.24613371181767,23.1286702508203,18.));
#35992=CARTESIAN_POINT('Ctrl Pts',(-6.27540581784971,23.1502801515009,0.));
#35993=CARTESIAN_POINT('Ctrl Pts',(-6.27540581784971,23.1502801515009,18.));
#35994=CARTESIAN_POINT('Ctrl Pts',(-6.29006564240226,23.1610680715348,0.));
#35995=CARTESIAN_POINT('Ctrl Pts',(-6.29006564240226,23.1610680715348,18.));
#35996=CARTESIAN_POINT('Ctrl Pts',(-2.66302778805429,18.6042245638953,0.));
#35997=CARTESIAN_POINT('Ctrl Pts',(-2.66524945599054,18.6197453967525,0.));
#35998=CARTESIAN_POINT('Ctrl Pts',(-2.67022099202408,18.6506703537007,0.));
#35999=CARTESIAN_POINT('Ctrl Pts',(-2.67926286296661,18.696707670787,0.));
#36000=CARTESIAN_POINT('Ctrl Pts',(-2.69432739305027,18.7574274222161,0.));
#36001=CARTESIAN_POINT('Ctrl Pts',(-2.71724545050994,18.8324337861517,0.));
#36002=CARTESIAN_POINT('Ctrl Pts',(-2.74308150095404,18.9068127424043,0.));
#36003=CARTESIAN_POINT('Ctrl Pts',(-2.77069196504715,18.980821277801,0.));
#36004=CARTESIAN_POINT('Ctrl Pts',(-2.79926206958176,19.0546365637297,0.));
#36005=CARTESIAN_POINT('Ctrl Pts',(-2.828507852372,19.1283090202125,0.));
#36006=CARTESIAN_POINT('Ctrl Pts',(-2.85848240467741,19.2018091932025,0.));
#36007=CARTESIAN_POINT('Ctrl Pts',(-2.88943670541708,19.2750617358775,0.));
#36008=CARTESIAN_POINT('Ctrl Pts',(-2.92166984506916,19.3479817954251,0.));
#36009=CARTESIAN_POINT('Ctrl Pts',(-2.95535900926266,19.420516469599,0.));
#36010=CARTESIAN_POINT('Ctrl Pts',(-2.99048468792079,19.4926628032527,0.));
#36011=CARTESIAN_POINT('Ctrl Pts',(-3.02691741043284,19.5644460803884,0.));
#36012=CARTESIAN_POINT('Ctrl Pts',(-3.06446889170638,19.635906849522,0.));
#36013=CARTESIAN_POINT('Ctrl Pts',(-3.10295238390997,19.7070857227052,0.));
#36014=CARTESIAN_POINT('Ctrl Pts',(-3.1422513957243,19.7780060327854,0.));
#36015=CARTESIAN_POINT('Ctrl Pts',(-3.18233430962982,19.8486701154397,0.));
#36016=CARTESIAN_POINT('Ctrl Pts',(-3.22321820350857,19.9190683616661,0.));
#36017=CARTESIAN_POINT('Ctrl Pts',(-3.26494616363974,19.9891848794807,0.));
#36018=CARTESIAN_POINT('Ctrl Pts',(-3.30756123886962,20.0590040020603,0.));
#36019=CARTESIAN_POINT('Ctrl Pts',(-3.351076475782,20.1285177769596,0.));
#36020=CARTESIAN_POINT('Ctrl Pts',(-3.39547305068767,20.1977264147619,0.));
#36021=CARTESIAN_POINT('Ctrl Pts',(-3.44071459161672,20.2666346804507,0.));
#36022=CARTESIAN_POINT('Ctrl Pts',(-3.48675677306966,20.3352494700167,0.));
#36023=CARTESIAN_POINT('Ctrl Pts',(-3.53355803178954,20.4035771072894,0.));
#36024=CARTESIAN_POINT('Ctrl Pts',(-3.58109188218494,20.4716202388531,0.));
#36025=CARTESIAN_POINT('Ctrl Pts',(-3.62934618720589,20.5393780076056,0.));
#36026=CARTESIAN_POINT('Ctrl Pts',(-3.67831730617887,20.6068475141781,0.));
#36027=CARTESIAN_POINT('Ctrl Pts',(-3.72800579849619,20.6740248879992,0.));
#36028=CARTESIAN_POINT('Ctrl Pts',(-3.77841179839888,20.740906441832,0.));
#36029=CARTESIAN_POINT('Ctrl Pts',(-3.82952970701915,20.8074899980321,0.));
#36030=CARTESIAN_POINT('Ctrl Pts',(-3.88134876172354,20.8737747416623,0.));
#36031=CARTESIAN_POINT('Ctrl Pts',(-3.93385538070582,20.9397606289993,0.));
#36032=CARTESIAN_POINT('Ctrl Pts',(-3.98703495407281,21.0054479357374,0.));
#36033=CARTESIAN_POINT('Ctrl Pts',(-4.04087373166023,21.0708367812416,0.));
#36034=CARTESIAN_POINT('Ctrl Pts',(-4.09536099504429,21.1359265833073,0.));
#36035=CARTESIAN_POINT('Ctrl Pts',(-4.15048873695645,21.2007161321625,0.));
#36036=CARTESIAN_POINT('Ctrl Pts',(-4.20625065101369,21.2652038365365,0.));
#36037=CARTESIAN_POINT('Ctrl Pts',(-4.26264132842711,21.3293879189372,0.));
#36038=CARTESIAN_POINT('Ctrl Pts',(-4.31965542378783,21.3932666198096,0.));
#36039=CARTESIAN_POINT('Ctrl Pts',(-4.37728667813637,21.4568384368826,0.));
#36040=CARTESIAN_POINT('Ctrl Pts',(-4.43552802047029,21.5201021036274,0.));
#36041=CARTESIAN_POINT('Ctrl Pts',(-4.49437199472474,21.5830564890896,0.));
#36042=CARTESIAN_POINT('Ctrl Pts',(-4.55381108432127,21.6457005243617,0.));
#36043=CARTESIAN_POINT('Ctrl Pts',(-4.6138380475249,21.7080331252945,0.));
#36044=CARTESIAN_POINT('Ctrl Pts',(-4.67444631371023,21.770053106418,0.));
#36045=CARTESIAN_POINT('Ctrl Pts',(-4.73562994468575,21.8317591750867,0.));
#36046=CARTESIAN_POINT('Ctrl Pts',(-4.7973834230091,21.8931499593332,0.));
#36047=CARTESIAN_POINT('Ctrl Pts',(-4.85970148585195,21.954224026919,0.));
#36048=CARTESIAN_POINT('Ctrl Pts',(-4.92257895332779,22.0149799098431,0.));
#36049=CARTESIAN_POINT('Ctrl Pts',(-4.98601051193086,22.0754161299398,0.));
#36050=CARTESIAN_POINT('Ctrl Pts',(-5.04999072201681,22.1355312202693,0.));
#36051=CARTESIAN_POINT('Ctrl Pts',(-5.11451415224483,22.1953237422816,0.));
#36052=CARTESIAN_POINT('Ctrl Pts',(-5.17957547700992,22.2547923093751,0.));
#36053=CARTESIAN_POINT('Ctrl Pts',(-5.24516957209272,22.3139356039553,0.));
#36054=CARTESIAN_POINT('Ctrl Pts',(-5.31129163978934,22.3727524152125,0.));
#36055=CARTESIAN_POINT('Ctrl Pts',(-5.37793718711213,22.4312416086453,0.));
#36056=CARTESIAN_POINT('Ctrl Pts',(-5.44510186987254,22.4894020366778,0.));
#36057=CARTESIAN_POINT('Ctrl Pts',(-5.51278136258486,22.5472324623564,0.));
#36058=CARTESIAN_POINT('Ctrl Pts',(-5.58097123210075,22.6047314918151,0.));
#36059=CARTESIAN_POINT('Ctrl Pts',(-5.64966676217478,22.6618974767817,0.));
#36060=CARTESIAN_POINT('Ctrl Pts',(-5.71886294543539,22.7187285302677,0.));
#36061=CARTESIAN_POINT('Ctrl Pts',(-5.7885547640031,22.7752227318719,0.));
#36062=CARTESIAN_POINT('Ctrl Pts',(-5.85873740439746,22.8313782965033,0.));
#36063=CARTESIAN_POINT('Ctrl Pts',(-5.92940648776744,22.8871937503747,0.));
#36064=CARTESIAN_POINT('Ctrl Pts',(-6.00055830861927,22.9426681304804,0.));
#36065=CARTESIAN_POINT('Ctrl Pts',(-6.0865163523085,23.0088276997724,0.));
#36066=CARTESIAN_POINT('Ctrl Pts',(-6.15874528113544,23.0635340031629,0.));
#36067=CARTESIAN_POINT('Ctrl Pts',(-6.21690914895776,23.107026289589,0.));
#36068=CARTESIAN_POINT('Ctrl Pts',(-6.26074599324763,23.1394922314359,0.));
#36069=CARTESIAN_POINT('Ctrl Pts',(-6.29006564240226,23.1610680715348,0.));
#36070=CARTESIAN_POINT('Ctrl Pts',(-2.66302778805429,18.6042245638953,15.));
#36071=CARTESIAN_POINT('Ctrl Pts',(-2.66524945599054,18.6197453967525,15.));
#36072=CARTESIAN_POINT('Ctrl Pts',(-2.67022099202408,18.6506703537007,15.));
#36073=CARTESIAN_POINT('Ctrl Pts',(-2.67926286296661,18.696707670787,15.));
#36074=CARTESIAN_POINT('Ctrl Pts',(-2.69432739305027,18.7574274222161,15.));
#36075=CARTESIAN_POINT('Ctrl Pts',(-2.71724545050994,18.8324337861517,15.));
#36076=CARTESIAN_POINT('Ctrl Pts',(-2.74308150095404,18.9068127424043,15.));
#36077=CARTESIAN_POINT('Ctrl Pts',(-2.77069196504715,18.980821277801,15.));
#36078=CARTESIAN_POINT('Ctrl Pts',(-2.79926206958176,19.0546365637297,15.));
#36079=CARTESIAN_POINT('Ctrl Pts',(-2.828507852372,19.1283090202125,15.));
#36080=CARTESIAN_POINT('Ctrl Pts',(-2.85848240467741,19.2018091932025,15.));
#36081=CARTESIAN_POINT('Ctrl Pts',(-2.88943670541708,19.2750617358775,15.));
#36082=CARTESIAN_POINT('Ctrl Pts',(-2.92166984506916,19.3479817954251,15.));
#36083=CARTESIAN_POINT('Ctrl Pts',(-2.95535900926266,19.420516469599,15.));
#36084=CARTESIAN_POINT('Ctrl Pts',(-2.99048468792079,19.4926628032527,15.));
#36085=CARTESIAN_POINT('Ctrl Pts',(-3.02691741043284,19.5644460803884,15.));
#36086=CARTESIAN_POINT('Ctrl Pts',(-3.06446889170638,19.635906849522,15.));
#36087=CARTESIAN_POINT('Ctrl Pts',(-3.10295238390997,19.7070857227052,15.));
#36088=CARTESIAN_POINT('Ctrl Pts',(-3.1422513957243,19.7780060327854,15.));
#36089=CARTESIAN_POINT('Ctrl Pts',(-3.18233430962982,19.8486701154397,15.));
#36090=CARTESIAN_POINT('Ctrl Pts',(-3.22321820350857,19.9190683616661,15.));
#36091=CARTESIAN_POINT('Ctrl Pts',(-3.26494616363974,19.9891848794807,15.));
#36092=CARTESIAN_POINT('Ctrl Pts',(-3.30756123886962,20.0590040020603,15.));
#36093=CARTESIAN_POINT('Ctrl Pts',(-3.351076475782,20.1285177769596,15.));
#36094=CARTESIAN_POINT('Ctrl Pts',(-3.39547305068767,20.1977264147619,15.));
#36095=CARTESIAN_POINT('Ctrl Pts',(-3.44071459161672,20.2666346804507,15.));
#36096=CARTESIAN_POINT('Ctrl Pts',(-3.48675677306966,20.3352494700167,15.));
#36097=CARTESIAN_POINT('Ctrl Pts',(-3.53355803178954,20.4035771072894,15.));
#36098=CARTESIAN_POINT('Ctrl Pts',(-3.58109188218494,20.4716202388531,15.));
#36099=CARTESIAN_POINT('Ctrl Pts',(-3.62934618720589,20.5393780076056,15.));
#36100=CARTESIAN_POINT('Ctrl Pts',(-3.67831730617887,20.6068475141781,15.));
#36101=CARTESIAN_POINT('Ctrl Pts',(-3.72800579849619,20.6740248879992,15.));
#36102=CARTESIAN_POINT('Ctrl Pts',(-3.77841179839888,20.740906441832,15.));
#36103=CARTESIAN_POINT('Ctrl Pts',(-3.82952970701915,20.8074899980321,15.));
#36104=CARTESIAN_POINT('Ctrl Pts',(-3.88134876172354,20.8737747416623,15.));
#36105=CARTESIAN_POINT('Ctrl Pts',(-3.93385538070582,20.9397606289993,15.));
#36106=CARTESIAN_POINT('Ctrl Pts',(-3.98703495407281,21.0054479357374,15.));
#36107=CARTESIAN_POINT('Ctrl Pts',(-4.04087373166023,21.0708367812416,15.));
#36108=CARTESIAN_POINT('Ctrl Pts',(-4.09536099504429,21.1359265833073,15.));
#36109=CARTESIAN_POINT('Ctrl Pts',(-4.15048873695645,21.2007161321625,15.));
#36110=CARTESIAN_POINT('Ctrl Pts',(-4.20625065101369,21.2652038365365,15.));
#36111=CARTESIAN_POINT('Ctrl Pts',(-4.26264132842711,21.3293879189372,15.));
#36112=CARTESIAN_POINT('Ctrl Pts',(-4.31965542378783,21.3932666198096,15.));
#36113=CARTESIAN_POINT('Ctrl Pts',(-4.37728667813637,21.4568384368826,15.));
#36114=CARTESIAN_POINT('Ctrl Pts',(-4.43552802047029,21.5201021036274,15.));
#36115=CARTESIAN_POINT('Ctrl Pts',(-4.49437199472474,21.5830564890896,15.));
#36116=CARTESIAN_POINT('Ctrl Pts',(-4.55381108432127,21.6457005243617,15.));
#36117=CARTESIAN_POINT('Ctrl Pts',(-4.6138380475249,21.7080331252945,15.));
#36118=CARTESIAN_POINT('Ctrl Pts',(-4.67444631371023,21.770053106418,15.));
#36119=CARTESIAN_POINT('Ctrl Pts',(-4.73562994468575,21.8317591750867,15.));
#36120=CARTESIAN_POINT('Ctrl Pts',(-4.7973834230091,21.8931499593332,15.));
#36121=CARTESIAN_POINT('Ctrl Pts',(-4.85970148585195,21.954224026919,15.));
#36122=CARTESIAN_POINT('Ctrl Pts',(-4.92257895332779,22.0149799098431,15.));
#36123=CARTESIAN_POINT('Ctrl Pts',(-4.98601051193086,22.0754161299398,15.));
#36124=CARTESIAN_POINT('Ctrl Pts',(-5.04999072201681,22.1355312202693,15.));
#36125=CARTESIAN_POINT('Ctrl Pts',(-5.11451415224483,22.1953237422816,15.));
#36126=CARTESIAN_POINT('Ctrl Pts',(-5.17957547700992,22.2547923093751,15.));
#36127=CARTESIAN_POINT('Ctrl Pts',(-5.24516957209272,22.3139356039553,15.));
#36128=CARTESIAN_POINT('Ctrl Pts',(-5.31129163978934,22.3727524152125,15.));
#36129=CARTESIAN_POINT('Ctrl Pts',(-5.37793718711213,22.4312416086453,15.));
#36130=CARTESIAN_POINT('Ctrl Pts',(-5.44510186987254,22.4894020366778,15.));
#36131=CARTESIAN_POINT('Ctrl Pts',(-5.51278136258486,22.5472324623564,15.));
#36132=CARTESIAN_POINT('Ctrl Pts',(-5.58097123210075,22.6047314918151,15.));
#36133=CARTESIAN_POINT('Ctrl Pts',(-5.64966676217478,22.6618974767817,15.));
#36134=CARTESIAN_POINT('Ctrl Pts',(-5.71886294543539,22.7187285302677,15.));
#36135=CARTESIAN_POINT('Ctrl Pts',(-5.7885547640031,22.7752227318719,15.));
#36136=CARTESIAN_POINT('Ctrl Pts',(-5.85873740439746,22.8313782965033,15.));
#36137=CARTESIAN_POINT('Ctrl Pts',(-5.92940648776744,22.8871937503747,15.));
#36138=CARTESIAN_POINT('Ctrl Pts',(-6.00055830861927,22.9426681304804,15.));
#36139=CARTESIAN_POINT('Ctrl Pts',(-6.0865163523085,23.0088276997724,15.));
#36140=CARTESIAN_POINT('Ctrl Pts',(-6.15874528113544,23.0635340031629,15.));
#36141=CARTESIAN_POINT('Ctrl Pts',(-6.21690914895776,23.107026289589,15.));
#36142=CARTESIAN_POINT('Ctrl Pts',(-6.26074599324763,23.1394922314359,15.));
#36143=CARTESIAN_POINT('Ctrl Pts',(-6.29006564240226,23.1610680715348,15.));
#36144=CARTESIAN_POINT('Ctrl Pts',(6.29006564240227,23.1610680715348,0.));
#36145=CARTESIAN_POINT('Ctrl Pts',(6.29006564240227,23.1610680715348,18.));
#36146=CARTESIAN_POINT('Ctrl Pts',(6.27540581784972,23.1502801515009,0.));
#36147=CARTESIAN_POINT('Ctrl Pts',(6.27540581784972,23.1502801515009,18.));
#36148=CARTESIAN_POINT('Ctrl Pts',(6.24613371181767,23.1286702508203,0.));
#36149=CARTESIAN_POINT('Ctrl Pts',(6.24613371181767,23.1286702508203,18.));
#36150=CARTESIAN_POINT('Ctrl Pts',(6.20236818200219,23.0961532179825,0.));
#36151=CARTESIAN_POINT('Ctrl Pts',(6.20236818200219,23.0961532179825,18.));
#36152=CARTESIAN_POINT('Ctrl Pts',(6.14429949537005,23.0525927424848,0.));
#36153=CARTESIAN_POINT('Ctrl Pts',(6.14429949537005,23.0525927424848,18.));
#36154=CARTESIAN_POINT('Ctrl Pts',(6.07219001169363,22.9978011048904,0.));
#36155=CARTESIAN_POINT('Ctrl Pts',(6.07219001169363,22.9978011048904,18.));
#36156=CARTESIAN_POINT('Ctrl Pts',(6.00055830861927,22.9426681304804,0.));
#36157=CARTESIAN_POINT('Ctrl Pts',(6.00055830861927,22.9426681304804,18.));
#36158=CARTESIAN_POINT('Ctrl Pts',(5.92940648776744,22.8871937503747,0.));
#36159=CARTESIAN_POINT('Ctrl Pts',(5.92940648776744,22.8871937503747,18.));
#36160=CARTESIAN_POINT('Ctrl Pts',(5.85873740439747,22.8313782965033,0.));
#36161=CARTESIAN_POINT('Ctrl Pts',(5.85873740439747,22.8313782965033,18.));
#36162=CARTESIAN_POINT('Ctrl Pts',(5.78855476400311,22.7752227318719,0.));
#36163=CARTESIAN_POINT('Ctrl Pts',(5.78855476400311,22.7752227318719,18.));
#36164=CARTESIAN_POINT('Ctrl Pts',(5.71886294543539,22.7187285302677,0.));
#36165=CARTESIAN_POINT('Ctrl Pts',(5.71886294543539,22.7187285302677,18.));
#36166=CARTESIAN_POINT('Ctrl Pts',(5.64966676217478,22.6618974767817,0.));
#36167=CARTESIAN_POINT('Ctrl Pts',(5.64966676217478,22.6618974767817,18.));
#36168=CARTESIAN_POINT('Ctrl Pts',(5.58097123210075,22.6047314918151,0.));
#36169=CARTESIAN_POINT('Ctrl Pts',(5.58097123210075,22.6047314918151,18.));
#36170=CARTESIAN_POINT('Ctrl Pts',(5.51278136258486,22.5472324623564,0.));
#36171=CARTESIAN_POINT('Ctrl Pts',(5.51278136258486,22.5472324623564,18.));
#36172=CARTESIAN_POINT('Ctrl Pts',(5.44510186987254,22.4894020366778,0.));
#36173=CARTESIAN_POINT('Ctrl Pts',(5.44510186987254,22.4894020366778,18.));
#36174=CARTESIAN_POINT('Ctrl Pts',(5.37793718711213,22.4312416086453,0.));
#36175=CARTESIAN_POINT('Ctrl Pts',(5.37793718711213,22.4312416086453,18.));
#36176=CARTESIAN_POINT('Ctrl Pts',(5.31129163978934,22.3727524152125,0.));
#36177=CARTESIAN_POINT('Ctrl Pts',(5.31129163978934,22.3727524152125,18.));
#36178=CARTESIAN_POINT('Ctrl Pts',(5.24516957209272,22.3139356039553,0.));
#36179=CARTESIAN_POINT('Ctrl Pts',(5.24516957209272,22.3139356039553,18.));
#36180=CARTESIAN_POINT('Ctrl Pts',(5.17957547700992,22.2547923093751,0.));
#36181=CARTESIAN_POINT('Ctrl Pts',(5.17957547700992,22.2547923093751,18.));
#36182=CARTESIAN_POINT('Ctrl Pts',(5.11451415224484,22.1953237422816,0.));
#36183=CARTESIAN_POINT('Ctrl Pts',(5.11451415224484,22.1953237422816,18.));
#36184=CARTESIAN_POINT('Ctrl Pts',(5.04999072201681,22.1355312202693,0.));
#36185=CARTESIAN_POINT('Ctrl Pts',(5.04999072201681,22.1355312202693,18.));
#36186=CARTESIAN_POINT('Ctrl Pts',(4.98601051193086,22.0754161299398,0.));
#36187=CARTESIAN_POINT('Ctrl Pts',(4.98601051193086,22.0754161299398,18.));
#36188=CARTESIAN_POINT('Ctrl Pts',(4.92257895332779,22.0149799098431,0.));
#36189=CARTESIAN_POINT('Ctrl Pts',(4.92257895332779,22.0149799098431,18.));
#36190=CARTESIAN_POINT('Ctrl Pts',(4.85970148585195,21.954224026919,0.));
#36191=CARTESIAN_POINT('Ctrl Pts',(4.85970148585195,21.954224026919,18.));
#36192=CARTESIAN_POINT('Ctrl Pts',(4.7973834230091,21.8931499593332,0.));
#36193=CARTESIAN_POINT('Ctrl Pts',(4.7973834230091,21.8931499593332,18.));
#36194=CARTESIAN_POINT('Ctrl Pts',(4.73562994468575,21.8317591750867,0.));
#36195=CARTESIAN_POINT('Ctrl Pts',(4.73562994468575,21.8317591750867,18.));
#36196=CARTESIAN_POINT('Ctrl Pts',(4.67444631371023,21.770053106418,0.));
#36197=CARTESIAN_POINT('Ctrl Pts',(4.67444631371023,21.770053106418,18.));
#36198=CARTESIAN_POINT('Ctrl Pts',(4.6138380475249,21.7080331252945,0.));
#36199=CARTESIAN_POINT('Ctrl Pts',(4.6138380475249,21.7080331252945,18.));
#36200=CARTESIAN_POINT('Ctrl Pts',(4.55381108432127,21.6457005243617,0.));
#36201=CARTESIAN_POINT('Ctrl Pts',(4.55381108432127,21.6457005243617,18.));
#36202=CARTESIAN_POINT('Ctrl Pts',(4.49437199472474,21.5830564890896,0.));
#36203=CARTESIAN_POINT('Ctrl Pts',(4.49437199472474,21.5830564890896,18.));
#36204=CARTESIAN_POINT('Ctrl Pts',(4.43552802047029,21.5201021036274,0.));
#36205=CARTESIAN_POINT('Ctrl Pts',(4.43552802047029,21.5201021036274,18.));
#36206=CARTESIAN_POINT('Ctrl Pts',(4.37728667813637,21.4568384368826,0.));
#36207=CARTESIAN_POINT('Ctrl Pts',(4.37728667813637,21.4568384368826,18.));
#36208=CARTESIAN_POINT('Ctrl Pts',(4.31965542378783,21.3932666198096,0.));
#36209=CARTESIAN_POINT('Ctrl Pts',(4.31965542378783,21.3932666198096,18.));
#36210=CARTESIAN_POINT('Ctrl Pts',(4.26264132842711,21.3293879189372,0.));
#36211=CARTESIAN_POINT('Ctrl Pts',(4.26264132842711,21.3293879189372,18.));
#36212=CARTESIAN_POINT('Ctrl Pts',(4.20625065101369,21.2652038365365,0.));
#36213=CARTESIAN_POINT('Ctrl Pts',(4.20625065101369,21.2652038365365,18.));
#36214=CARTESIAN_POINT('Ctrl Pts',(4.15048873695645,21.2007161321625,0.));
#36215=CARTESIAN_POINT('Ctrl Pts',(4.15048873695645,21.2007161321625,18.));
#36216=CARTESIAN_POINT('Ctrl Pts',(4.09536099504429,21.1359265833073,0.));
#36217=CARTESIAN_POINT('Ctrl Pts',(4.09536099504429,21.1359265833073,18.));
#36218=CARTESIAN_POINT('Ctrl Pts',(4.04087373166023,21.0708367812416,0.));
#36219=CARTESIAN_POINT('Ctrl Pts',(4.04087373166023,21.0708367812416,18.));
#36220=CARTESIAN_POINT('Ctrl Pts',(3.98703495407281,21.0054479357374,0.));
#36221=CARTESIAN_POINT('Ctrl Pts',(3.98703495407281,21.0054479357374,18.));
#36222=CARTESIAN_POINT('Ctrl Pts',(3.93385538070582,20.9397606289993,0.));
#36223=CARTESIAN_POINT('Ctrl Pts',(3.93385538070582,20.9397606289993,18.));
#36224=CARTESIAN_POINT('Ctrl Pts',(3.88134876172354,20.8737747416623,0.));
#36225=CARTESIAN_POINT('Ctrl Pts',(3.88134876172354,20.8737747416623,18.));
#36226=CARTESIAN_POINT('Ctrl Pts',(3.82952970701916,20.8074899980321,0.));
#36227=CARTESIAN_POINT('Ctrl Pts',(3.82952970701916,20.8074899980321,18.));
#36228=CARTESIAN_POINT('Ctrl Pts',(3.77841179839888,20.740906441832,0.));
#36229=CARTESIAN_POINT('Ctrl Pts',(3.77841179839888,20.740906441832,18.));
#36230=CARTESIAN_POINT('Ctrl Pts',(3.7280057984962,20.6740248879992,0.));
#36231=CARTESIAN_POINT('Ctrl Pts',(3.7280057984962,20.6740248879992,18.));
#36232=CARTESIAN_POINT('Ctrl Pts',(3.67831730617888,20.6068475141781,0.));
#36233=CARTESIAN_POINT('Ctrl Pts',(3.67831730617888,20.6068475141781,18.));
#36234=CARTESIAN_POINT('Ctrl Pts',(3.6293461872059,20.5393780076056,0.));
#36235=CARTESIAN_POINT('Ctrl Pts',(3.6293461872059,20.5393780076056,18.));
#36236=CARTESIAN_POINT('Ctrl Pts',(3.58109188218494,20.4716202388531,0.));
#36237=CARTESIAN_POINT('Ctrl Pts',(3.58109188218494,20.4716202388531,18.));
#36238=CARTESIAN_POINT('Ctrl Pts',(3.53355803178955,20.4035771072894,0.));
#36239=CARTESIAN_POINT('Ctrl Pts',(3.53355803178955,20.4035771072894,18.));
#36240=CARTESIAN_POINT('Ctrl Pts',(3.48675677306966,20.3352494700167,0.));
#36241=CARTESIAN_POINT('Ctrl Pts',(3.48675677306966,20.3352494700167,18.));
#36242=CARTESIAN_POINT('Ctrl Pts',(3.44071459161672,20.2666346804507,0.));
#36243=CARTESIAN_POINT('Ctrl Pts',(3.44071459161672,20.2666346804507,18.));
#36244=CARTESIAN_POINT('Ctrl Pts',(3.39547305068768,20.1977264147619,0.));
#36245=CARTESIAN_POINT('Ctrl Pts',(3.39547305068768,20.1977264147619,18.));
#36246=CARTESIAN_POINT('Ctrl Pts',(3.35107647578201,20.1285177769596,0.));
#36247=CARTESIAN_POINT('Ctrl Pts',(3.35107647578201,20.1285177769596,18.));
#36248=CARTESIAN_POINT('Ctrl Pts',(3.30756123886962,20.0590040020604,0.));
#36249=CARTESIAN_POINT('Ctrl Pts',(3.30756123886962,20.0590040020604,18.));
#36250=CARTESIAN_POINT('Ctrl Pts',(3.26494616363974,19.9891848794807,0.));
#36251=CARTESIAN_POINT('Ctrl Pts',(3.26494616363974,19.9891848794807,18.));
#36252=CARTESIAN_POINT('Ctrl Pts',(3.22321820350857,19.9190683616661,0.));
#36253=CARTESIAN_POINT('Ctrl Pts',(3.22321820350857,19.9190683616661,18.));
#36254=CARTESIAN_POINT('Ctrl Pts',(3.18233430962982,19.8486701154397,0.));
#36255=CARTESIAN_POINT('Ctrl Pts',(3.18233430962982,19.8486701154397,18.));
#36256=CARTESIAN_POINT('Ctrl Pts',(3.14225139572431,19.7780060327854,0.));
#36257=CARTESIAN_POINT('Ctrl Pts',(3.14225139572431,19.7780060327854,18.));
#36258=CARTESIAN_POINT('Ctrl Pts',(3.10295238390997,19.7070857227052,0.));
#36259=CARTESIAN_POINT('Ctrl Pts',(3.10295238390997,19.7070857227052,18.));
#36260=CARTESIAN_POINT('Ctrl Pts',(3.06446889170638,19.635906849522,0.));
#36261=CARTESIAN_POINT('Ctrl Pts',(3.06446889170638,19.635906849522,18.));
#36262=CARTESIAN_POINT('Ctrl Pts',(3.02691741043284,19.5644460803884,0.));
#36263=CARTESIAN_POINT('Ctrl Pts',(3.02691741043284,19.5644460803884,18.));
#36264=CARTESIAN_POINT('Ctrl Pts',(2.99048468792079,19.4926628032527,0.));
#36265=CARTESIAN_POINT('Ctrl Pts',(2.99048468792079,19.4926628032527,18.));
#36266=CARTESIAN_POINT('Ctrl Pts',(2.95535900926266,19.420516469599,0.));
#36267=CARTESIAN_POINT('Ctrl Pts',(2.95535900926266,19.420516469599,18.));
#36268=CARTESIAN_POINT('Ctrl Pts',(2.92166984506916,19.3479817954251,0.));
#36269=CARTESIAN_POINT('Ctrl Pts',(2.92166984506916,19.3479817954251,18.));
#36270=CARTESIAN_POINT('Ctrl Pts',(2.88943670541709,19.2750617358775,0.));
#36271=CARTESIAN_POINT('Ctrl Pts',(2.88943670541709,19.2750617358775,18.));
#36272=CARTESIAN_POINT('Ctrl Pts',(2.85848240467741,19.2018091932025,0.));
#36273=CARTESIAN_POINT('Ctrl Pts',(2.85848240467741,19.2018091932025,18.));
#36274=CARTESIAN_POINT('Ctrl Pts',(2.828507852372,19.1283090202125,0.));
#36275=CARTESIAN_POINT('Ctrl Pts',(2.828507852372,19.1283090202125,18.));
#36276=CARTESIAN_POINT('Ctrl Pts',(2.79926206958176,19.0546365637297,0.));
#36277=CARTESIAN_POINT('Ctrl Pts',(2.79926206958176,19.0546365637297,18.));
#36278=CARTESIAN_POINT('Ctrl Pts',(2.77069196504715,18.980821277801,0.));
#36279=CARTESIAN_POINT('Ctrl Pts',(2.77069196504715,18.980821277801,18.));
#36280=CARTESIAN_POINT('Ctrl Pts',(2.74308150095405,18.9068127424043,0.));
#36281=CARTESIAN_POINT('Ctrl Pts',(2.74308150095405,18.9068127424043,18.));
#36282=CARTESIAN_POINT('Ctrl Pts',(2.71724545050995,18.8324337861517,0.));
#36283=CARTESIAN_POINT('Ctrl Pts',(2.71724545050995,18.8324337861517,18.));
#36284=CARTESIAN_POINT('Ctrl Pts',(2.69432739305028,18.7574274222161,0.));
#36285=CARTESIAN_POINT('Ctrl Pts',(2.69432739305028,18.7574274222161,18.));
#36286=CARTESIAN_POINT('Ctrl Pts',(2.67926286296661,18.696707670787,0.));
#36287=CARTESIAN_POINT('Ctrl Pts',(2.67926286296661,18.696707670787,18.));
#36288=CARTESIAN_POINT('Ctrl Pts',(2.67022099202409,18.6506703537007,0.));
#36289=CARTESIAN_POINT('Ctrl Pts',(2.67022099202409,18.6506703537007,18.));
#36290=CARTESIAN_POINT('Ctrl Pts',(2.66524945599055,18.6197453967525,0.));
#36291=CARTESIAN_POINT('Ctrl Pts',(2.66524945599055,18.6197453967525,18.));
#36292=CARTESIAN_POINT('Ctrl Pts',(2.66302778805429,18.6042245638953,0.));
#36293=CARTESIAN_POINT('Ctrl Pts',(2.66302778805429,18.6042245638953,18.));
#36294=CARTESIAN_POINT('',(6.29006564240232,23.1610680715348,0.));
#36295=CARTESIAN_POINT('Ctrl Pts',(2.66302778805429,18.6042245638953,0.));
#36296=CARTESIAN_POINT('Ctrl Pts',(2.66524945599055,18.6197453967525,0.));
#36297=CARTESIAN_POINT('Ctrl Pts',(2.67022099202409,18.6506703537007,0.));
#36298=CARTESIAN_POINT('Ctrl Pts',(2.67926286296661,18.696707670787,0.));
#36299=CARTESIAN_POINT('Ctrl Pts',(2.69432739305028,18.7574274222161,0.));
#36300=CARTESIAN_POINT('Ctrl Pts',(2.71724545050995,18.8324337861517,0.));
#36301=CARTESIAN_POINT('Ctrl Pts',(2.74308150095405,18.9068127424043,0.));
#36302=CARTESIAN_POINT('Ctrl Pts',(2.77069196504715,18.980821277801,0.));
#36303=CARTESIAN_POINT('Ctrl Pts',(2.79926206958176,19.0546365637297,0.));
#36304=CARTESIAN_POINT('Ctrl Pts',(2.828507852372,19.1283090202125,0.));
#36305=CARTESIAN_POINT('Ctrl Pts',(2.85848240467741,19.2018091932025,0.));
#36306=CARTESIAN_POINT('Ctrl Pts',(2.88943670541709,19.2750617358775,0.));
#36307=CARTESIAN_POINT('Ctrl Pts',(2.92166984506916,19.3479817954251,0.));
#36308=CARTESIAN_POINT('Ctrl Pts',(2.95535900926266,19.420516469599,0.));
#36309=CARTESIAN_POINT('Ctrl Pts',(2.99048468792079,19.4926628032527,0.));
#36310=CARTESIAN_POINT('Ctrl Pts',(3.02691741043284,19.5644460803884,0.));
#36311=CARTESIAN_POINT('Ctrl Pts',(3.06446889170638,19.635906849522,0.));
#36312=CARTESIAN_POINT('Ctrl Pts',(3.10295238390997,19.7070857227052,0.));
#36313=CARTESIAN_POINT('Ctrl Pts',(3.14225139572431,19.7780060327854,0.));
#36314=CARTESIAN_POINT('Ctrl Pts',(3.18233430962982,19.8486701154397,0.));
#36315=CARTESIAN_POINT('Ctrl Pts',(3.22321820350857,19.9190683616661,0.));
#36316=CARTESIAN_POINT('Ctrl Pts',(3.26494616363974,19.9891848794807,0.));
#36317=CARTESIAN_POINT('Ctrl Pts',(3.30756123886962,20.0590040020604,0.));
#36318=CARTESIAN_POINT('Ctrl Pts',(3.35107647578201,20.1285177769596,0.));
#36319=CARTESIAN_POINT('Ctrl Pts',(3.39547305068768,20.1977264147619,0.));
#36320=CARTESIAN_POINT('Ctrl Pts',(3.44071459161672,20.2666346804507,0.));
#36321=CARTESIAN_POINT('Ctrl Pts',(3.48675677306966,20.3352494700167,0.));
#36322=CARTESIAN_POINT('Ctrl Pts',(3.53355803178955,20.4035771072894,0.));
#36323=CARTESIAN_POINT('Ctrl Pts',(3.58109188218494,20.4716202388531,0.));
#36324=CARTESIAN_POINT('Ctrl Pts',(3.6293461872059,20.5393780076056,0.));
#36325=CARTESIAN_POINT('Ctrl Pts',(3.67831730617888,20.6068475141781,0.));
#36326=CARTESIAN_POINT('Ctrl Pts',(3.7280057984962,20.6740248879992,0.));
#36327=CARTESIAN_POINT('Ctrl Pts',(3.77841179839888,20.740906441832,0.));
#36328=CARTESIAN_POINT('Ctrl Pts',(3.82952970701916,20.8074899980321,0.));
#36329=CARTESIAN_POINT('Ctrl Pts',(3.88134876172354,20.8737747416623,0.));
#36330=CARTESIAN_POINT('Ctrl Pts',(3.93385538070582,20.9397606289993,0.));
#36331=CARTESIAN_POINT('Ctrl Pts',(3.98703495407281,21.0054479357374,0.));
#36332=CARTESIAN_POINT('Ctrl Pts',(4.04087373166023,21.0708367812416,0.));
#36333=CARTESIAN_POINT('Ctrl Pts',(4.09536099504429,21.1359265833073,0.));
#36334=CARTESIAN_POINT('Ctrl Pts',(4.15048873695645,21.2007161321625,0.));
#36335=CARTESIAN_POINT('Ctrl Pts',(4.20625065101369,21.2652038365365,0.));
#36336=CARTESIAN_POINT('Ctrl Pts',(4.26264132842711,21.3293879189372,0.));
#36337=CARTESIAN_POINT('Ctrl Pts',(4.31965542378783,21.3932666198096,0.));
#36338=CARTESIAN_POINT('Ctrl Pts',(4.37728667813637,21.4568384368826,0.));
#36339=CARTESIAN_POINT('Ctrl Pts',(4.43552802047029,21.5201021036274,0.));
#36340=CARTESIAN_POINT('Ctrl Pts',(4.49437199472474,21.5830564890896,0.));
#36341=CARTESIAN_POINT('Ctrl Pts',(4.55381108432127,21.6457005243617,0.));
#36342=CARTESIAN_POINT('Ctrl Pts',(4.6138380475249,21.7080331252945,0.));
#36343=CARTESIAN_POINT('Ctrl Pts',(4.67444631371023,21.770053106418,0.));
#36344=CARTESIAN_POINT('Ctrl Pts',(4.73562994468575,21.8317591750867,0.));
#36345=CARTESIAN_POINT('Ctrl Pts',(4.7973834230091,21.8931499593332,0.));
#36346=CARTESIAN_POINT('Ctrl Pts',(4.85970148585195,21.954224026919,0.));
#36347=CARTESIAN_POINT('Ctrl Pts',(4.92257895332779,22.0149799098431,0.));
#36348=CARTESIAN_POINT('Ctrl Pts',(4.98601051193086,22.0754161299398,0.));
#36349=CARTESIAN_POINT('Ctrl Pts',(5.04999072201681,22.1355312202693,0.));
#36350=CARTESIAN_POINT('Ctrl Pts',(5.11451415224484,22.1953237422816,0.));
#36351=CARTESIAN_POINT('Ctrl Pts',(5.17957547700992,22.2547923093751,0.));
#36352=CARTESIAN_POINT('Ctrl Pts',(5.24516957209272,22.3139356039553,0.));
#36353=CARTESIAN_POINT('Ctrl Pts',(5.31129163978934,22.3727524152125,0.));
#36354=CARTESIAN_POINT('Ctrl Pts',(5.37793718711213,22.4312416086453,0.));
#36355=CARTESIAN_POINT('Ctrl Pts',(5.44510186987254,22.4894020366778,0.));
#36356=CARTESIAN_POINT('Ctrl Pts',(5.51278136258486,22.5472324623564,0.));
#36357=CARTESIAN_POINT('Ctrl Pts',(5.58097123210075,22.6047314918151,0.));
#36358=CARTESIAN_POINT('Ctrl Pts',(5.64966676217478,22.6618974767817,0.));
#36359=CARTESIAN_POINT('Ctrl Pts',(5.71886294543539,22.7187285302677,0.));
#36360=CARTESIAN_POINT('Ctrl Pts',(5.78855476400311,22.7752227318719,0.));
#36361=CARTESIAN_POINT('Ctrl Pts',(5.85873740439747,22.8313782965033,0.));
#36362=CARTESIAN_POINT('Ctrl Pts',(5.92940648776744,22.8871937503747,0.));
#36363=CARTESIAN_POINT('Ctrl Pts',(6.00055830861927,22.9426681304804,0.));
#36364=CARTESIAN_POINT('Ctrl Pts',(6.0865163523085,23.0088276997724,0.));
#36365=CARTESIAN_POINT('Ctrl Pts',(6.15874528113544,23.0635340031629,0.));
#36366=CARTESIAN_POINT('Ctrl Pts',(6.21690914895778,23.107026289589,0.));
#36367=CARTESIAN_POINT('Ctrl Pts',(6.26074599324762,23.1394922314359,0.));
#36368=CARTESIAN_POINT('Ctrl Pts',(6.29006564240227,23.1610680715348,0.));
#36369=CARTESIAN_POINT('',(6.29006564240232,23.1610680715348,15.));
#36370=CARTESIAN_POINT('Ctrl Pts',(6.29006564240227,23.1610680715348,15.));
#36371=CARTESIAN_POINT('Ctrl Pts',(6.27540581784972,23.1502801515009,15.));
#36372=CARTESIAN_POINT('Ctrl Pts',(6.24613371181767,23.1286702508203,15.));
#36373=CARTESIAN_POINT('Ctrl Pts',(6.20236818200219,23.0961532179825,15.));
#36374=CARTESIAN_POINT('Ctrl Pts',(6.14429949537005,23.0525927424848,15.));
#36375=CARTESIAN_POINT('Ctrl Pts',(6.07219001169363,22.9978011048904,15.));
#36376=CARTESIAN_POINT('Ctrl Pts',(6.00055830861927,22.9426681304804,15.));
#36377=CARTESIAN_POINT('Ctrl Pts',(5.92940648776744,22.8871937503747,15.));
#36378=CARTESIAN_POINT('Ctrl Pts',(5.85873740439747,22.8313782965033,15.));
#36379=CARTESIAN_POINT('Ctrl Pts',(5.78855476400311,22.7752227318719,15.));
#36380=CARTESIAN_POINT('Ctrl Pts',(5.71886294543539,22.7187285302677,15.));
#36381=CARTESIAN_POINT('Ctrl Pts',(5.64966676217478,22.6618974767817,15.));
#36382=CARTESIAN_POINT('Ctrl Pts',(5.58097123210075,22.6047314918151,15.));
#36383=CARTESIAN_POINT('Ctrl Pts',(5.51278136258486,22.5472324623564,15.));
#36384=CARTESIAN_POINT('Ctrl Pts',(5.44510186987254,22.4894020366778,15.));
#36385=CARTESIAN_POINT('Ctrl Pts',(5.37793718711213,22.4312416086453,15.));
#36386=CARTESIAN_POINT('Ctrl Pts',(5.31129163978934,22.3727524152125,15.));
#36387=CARTESIAN_POINT('Ctrl Pts',(5.24516957209272,22.3139356039553,15.));
#36388=CARTESIAN_POINT('Ctrl Pts',(5.17957547700992,22.2547923093751,15.));
#36389=CARTESIAN_POINT('Ctrl Pts',(5.11451415224484,22.1953237422816,15.));
#36390=CARTESIAN_POINT('Ctrl Pts',(5.04999072201681,22.1355312202693,15.));
#36391=CARTESIAN_POINT('Ctrl Pts',(4.98601051193086,22.0754161299398,15.));
#36392=CARTESIAN_POINT('Ctrl Pts',(4.92257895332779,22.0149799098431,15.));
#36393=CARTESIAN_POINT('Ctrl Pts',(4.85970148585195,21.954224026919,15.));
#36394=CARTESIAN_POINT('Ctrl Pts',(4.7973834230091,21.8931499593332,15.));
#36395=CARTESIAN_POINT('Ctrl Pts',(4.73562994468575,21.8317591750867,15.));
#36396=CARTESIAN_POINT('Ctrl Pts',(4.67444631371023,21.770053106418,15.));
#36397=CARTESIAN_POINT('Ctrl Pts',(4.6138380475249,21.7080331252945,15.));
#36398=CARTESIAN_POINT('Ctrl Pts',(4.55381108432127,21.6457005243617,15.));
#36399=CARTESIAN_POINT('Ctrl Pts',(4.49437199472474,21.5830564890896,15.));
#36400=CARTESIAN_POINT('Ctrl Pts',(4.43552802047029,21.5201021036274,15.));
#36401=CARTESIAN_POINT('Ctrl Pts',(4.37728667813637,21.4568384368826,15.));
#36402=CARTESIAN_POINT('Ctrl Pts',(4.31965542378783,21.3932666198096,15.));
#36403=CARTESIAN_POINT('Ctrl Pts',(4.26264132842711,21.3293879189372,15.));
#36404=CARTESIAN_POINT('Ctrl Pts',(4.20625065101369,21.2652038365365,15.));
#36405=CARTESIAN_POINT('Ctrl Pts',(4.15048873695645,21.2007161321625,15.));
#36406=CARTESIAN_POINT('Ctrl Pts',(4.09536099504429,21.1359265833073,15.));
#36407=CARTESIAN_POINT('Ctrl Pts',(4.04087373166023,21.0708367812416,15.));
#36408=CARTESIAN_POINT('Ctrl Pts',(3.98703495407281,21.0054479357374,15.));
#36409=CARTESIAN_POINT('Ctrl Pts',(3.93385538070582,20.9397606289993,15.));
#36410=CARTESIAN_POINT('Ctrl Pts',(3.88134876172354,20.8737747416623,15.));
#36411=CARTESIAN_POINT('Ctrl Pts',(3.82952970701916,20.8074899980321,15.));
#36412=CARTESIAN_POINT('Ctrl Pts',(3.77841179839888,20.740906441832,15.));
#36413=CARTESIAN_POINT('Ctrl Pts',(3.7280057984962,20.6740248879992,15.));
#36414=CARTESIAN_POINT('Ctrl Pts',(3.67831730617888,20.6068475141781,15.));
#36415=CARTESIAN_POINT('Ctrl Pts',(3.6293461872059,20.5393780076056,15.));
#36416=CARTESIAN_POINT('Ctrl Pts',(3.58109188218494,20.4716202388531,15.));
#36417=CARTESIAN_POINT('Ctrl Pts',(3.53355803178955,20.4035771072894,15.));
#36418=CARTESIAN_POINT('Ctrl Pts',(3.48675677306966,20.3352494700167,15.));
#36419=CARTESIAN_POINT('Ctrl Pts',(3.44071459161672,20.2666346804507,15.));
#36420=CARTESIAN_POINT('Ctrl Pts',(3.39547305068768,20.1977264147619,15.));
#36421=CARTESIAN_POINT('Ctrl Pts',(3.35107647578201,20.1285177769596,15.));
#36422=CARTESIAN_POINT('Ctrl Pts',(3.30756123886962,20.0590040020604,15.));
#36423=CARTESIAN_POINT('Ctrl Pts',(3.26494616363974,19.9891848794807,15.));
#36424=CARTESIAN_POINT('Ctrl Pts',(3.22321820350857,19.9190683616661,15.));
#36425=CARTESIAN_POINT('Ctrl Pts',(3.18233430962982,19.8486701154397,15.));
#36426=CARTESIAN_POINT('Ctrl Pts',(3.14225139572431,19.7780060327854,15.));
#36427=CARTESIAN_POINT('Ctrl Pts',(3.10295238390997,19.7070857227052,15.));
#36428=CARTESIAN_POINT('Ctrl Pts',(3.06446889170638,19.635906849522,15.));
#36429=CARTESIAN_POINT('Ctrl Pts',(3.02691741043284,19.5644460803884,15.));
#36430=CARTESIAN_POINT('Ctrl Pts',(2.99048468792079,19.4926628032527,15.));
#36431=CARTESIAN_POINT('Ctrl Pts',(2.95535900926266,19.420516469599,15.));
#36432=CARTESIAN_POINT('Ctrl Pts',(2.92166984506916,19.3479817954251,15.));
#36433=CARTESIAN_POINT('Ctrl Pts',(2.88943670541709,19.2750617358775,15.));
#36434=CARTESIAN_POINT('Ctrl Pts',(2.85848240467741,19.2018091932025,15.));
#36435=CARTESIAN_POINT('Ctrl Pts',(2.828507852372,19.1283090202125,15.));
#36436=CARTESIAN_POINT('Ctrl Pts',(2.79926206958176,19.0546365637297,15.));
#36437=CARTESIAN_POINT('Ctrl Pts',(2.77069196504715,18.980821277801,15.));
#36438=CARTESIAN_POINT('Ctrl Pts',(2.74308150095405,18.9068127424043,15.));
#36439=CARTESIAN_POINT('Ctrl Pts',(2.71724545050995,18.8324337861517,15.));
#36440=CARTESIAN_POINT('Ctrl Pts',(2.69432739305028,18.7574274222161,15.));
#36441=CARTESIAN_POINT('Ctrl Pts',(2.67926286296661,18.696707670787,15.));
#36442=CARTESIAN_POINT('Ctrl Pts',(2.67022099202409,18.6506703537007,15.));
#36443=CARTESIAN_POINT('Ctrl Pts',(2.66524945599055,18.6197453967525,15.));
#36444=CARTESIAN_POINT('Ctrl Pts',(2.66302778805429,18.6042245638953,15.));
#36445=CARTESIAN_POINT('',(6.29006564240232,23.1610680715348,0.));
#36446=CARTESIAN_POINT('Origin',(3.57460821468069E-14,1.09790581218125E-13,
0.));
#36447=CARTESIAN_POINT('',(8.52496423935284,22.4349054983023,0.));
#36448=CARTESIAN_POINT('Origin',(3.57460821468069E-14,1.09790581218125E-13,
0.));
#36449=CARTESIAN_POINT('',(8.52496423935284,22.4349054983023,15.));
#36450=CARTESIAN_POINT('Origin',(3.57460821468069E-14,1.09790581218125E-13,
15.));
#36451=CARTESIAN_POINT('',(8.52496423935284,22.4349054983023,0.));
#36452=CARTESIAN_POINT('Ctrl Pts',(8.78085409196639,16.6164222996225,0.));
#36453=CARTESIAN_POINT('Ctrl Pts',(8.78085409196639,16.6164222996225,18.));
#36454=CARTESIAN_POINT('Ctrl Pts',(8.78817964150686,16.6302847808193,0.));
#36455=CARTESIAN_POINT('Ctrl Pts',(8.78817964150686,16.6302847808193,18.));
#36456=CARTESIAN_POINT('Ctrl Pts',(8.80233481798951,16.6582257921024,0.));
#36457=CARTESIAN_POINT('Ctrl Pts',(8.80233481798951,16.6582257921024,18.));
#36458=CARTESIAN_POINT('Ctrl Pts',(8.82207984677447,16.7007854423938,0.));
#36459=CARTESIAN_POINT('Ctrl Pts',(8.82207984677447,16.7007854423938,18.));
#36460=CARTESIAN_POINT('Ctrl Pts',(8.84558256033742,16.7587634618101,0.));
#36461=CARTESIAN_POINT('Ctrl Pts',(8.84558256033742,16.7587634618101,18.));
#36462=CARTESIAN_POINT('Ctrl Pts',(8.87112909692392,16.8329157811062,0.));
#36463=CARTESIAN_POINT('Ctrl Pts',(8.87112909692392,16.8329157811062,18.));
#36464=CARTESIAN_POINT('Ctrl Pts',(8.89394614661328,16.908275670167,0.));
#36465=CARTESIAN_POINT('Ctrl Pts',(8.89394614661328,16.908275670167,18.));
#36466=CARTESIAN_POINT('Ctrl Pts',(8.91510993758932,16.9843788566346,0.));
#36467=CARTESIAN_POINT('Ctrl Pts',(8.91510993758932,16.9843788566346,18.));
#36468=CARTESIAN_POINT('Ctrl Pts',(8.93538377395243,17.0608897634975,0.));
#36469=CARTESIAN_POINT('Ctrl Pts',(8.93538377395243,17.0608897634975,18.));
#36470=CARTESIAN_POINT('Ctrl Pts',(8.95502702208203,17.1376822726252,0.));
#36471=CARTESIAN_POINT('Ctrl Pts',(8.95502702208203,17.1376822726252,18.));
#36472=CARTESIAN_POINT('Ctrl Pts',(8.97397941759265,17.2147637614528,0.));
#36473=CARTESIAN_POINT('Ctrl Pts',(8.97397941759265,17.2147637614528,18.));
#36474=CARTESIAN_POINT('Ctrl Pts',(8.99199362652257,17.2922207948279,0.));
#36475=CARTESIAN_POINT('Ctrl Pts',(8.99199362652257,17.2922207948279,18.));
#36476=CARTESIAN_POINT('Ctrl Pts',(9.00877780436037,17.3701605263553,0.));
#36477=CARTESIAN_POINT('Ctrl Pts',(9.00877780436037,17.3701605263553,18.));
#36478=CARTESIAN_POINT('Ctrl Pts',(9.0241575097608,17.4486443043185,0.));
#36479=CARTESIAN_POINT('Ctrl Pts',(9.0241575097608,17.4486443043185,18.));
#36480=CARTESIAN_POINT('Ctrl Pts',(9.03814678971601,17.5276582702181,0.));
#36481=CARTESIAN_POINT('Ctrl Pts',(9.03814678971601,17.5276582702181,18.));
#36482=CARTESIAN_POINT('Ctrl Pts',(9.05086524971401,17.6071467783263,0.));
#36483=CARTESIAN_POINT('Ctrl Pts',(9.05086524971401,17.6071467783263,18.));
#36484=CARTESIAN_POINT('Ctrl Pts',(9.06248904941395,17.6870319618808,0.));
#36485=CARTESIAN_POINT('Ctrl Pts',(9.06248904941395,17.6870319618808,18.));
#36486=CARTESIAN_POINT('Ctrl Pts',(9.07319314215026,17.7672369091005,0.));
#36487=CARTESIAN_POINT('Ctrl Pts',(9.07319314215026,17.7672369091005,18.));
#36488=CARTESIAN_POINT('Ctrl Pts',(9.08308548608349,17.8477120247758,0.));
#36489=CARTESIAN_POINT('Ctrl Pts',(9.08308548608349,17.8477120247758,18.));
#36490=CARTESIAN_POINT('Ctrl Pts',(9.09219303320079,17.9284406141976,0.));
#36491=CARTESIAN_POINT('Ctrl Pts',(9.09219303320079,17.9284406141976,18.));
#36492=CARTESIAN_POINT('Ctrl Pts',(9.10049631917583,18.0094249416472,0.));
#36493=CARTESIAN_POINT('Ctrl Pts',(9.10049631917583,18.0094249416472,18.));
#36494=CARTESIAN_POINT('Ctrl Pts',(9.10795114540259,18.0906774757189,0.));
#36495=CARTESIAN_POINT('Ctrl Pts',(9.10795114540259,18.0906774757189,18.));
#36496=CARTESIAN_POINT('Ctrl Pts',(9.11451347590539,18.1722108451637,0.));
#36497=CARTESIAN_POINT('Ctrl Pts',(9.11451347590539,18.1722108451637,18.));
#36498=CARTESIAN_POINT('Ctrl Pts',(9.12016808144599,18.2540262849075,0.));
#36499=CARTESIAN_POINT('Ctrl Pts',(9.12016808144599,18.2540262849075,18.));
#36500=CARTESIAN_POINT('Ctrl Pts',(9.12493031448671,18.3361129010289,0.));
#36501=CARTESIAN_POINT('Ctrl Pts',(9.12493031448671,18.3361129010289,18.));
#36502=CARTESIAN_POINT('Ctrl Pts',(9.12883240135631,18.4184531695731,0.));
#36503=CARTESIAN_POINT('Ctrl Pts',(9.12883240135631,18.4184531695731,18.));
#36504=CARTESIAN_POINT('Ctrl Pts',(9.13191425549883,18.5010266156389,0.));
#36505=CARTESIAN_POINT('Ctrl Pts',(9.13191425549883,18.5010266156389,18.));
#36506=CARTESIAN_POINT('Ctrl Pts',(9.13421321934922,18.5838139250423,0.));
#36507=CARTESIAN_POINT('Ctrl Pts',(9.13421321934922,18.5838139250423,18.));
#36508=CARTESIAN_POINT('Ctrl Pts',(9.13575227582418,18.6668016710749,0.));
#36509=CARTESIAN_POINT('Ctrl Pts',(9.13575227582418,18.6668016710749,18.));
#36510=CARTESIAN_POINT('Ctrl Pts',(9.13654074021147,18.7499820263476,0.));
#36511=CARTESIAN_POINT('Ctrl Pts',(9.13654074021147,18.7499820263476,18.));
#36512=CARTESIAN_POINT('Ctrl Pts',(9.13657985367154,18.8333505052874,0.));
#36513=CARTESIAN_POINT('Ctrl Pts',(9.13657985367154,18.8333505052874,18.));
#36514=CARTESIAN_POINT('Ctrl Pts',(9.13586688858169,18.9169043053388,0.));
#36515=CARTESIAN_POINT('Ctrl Pts',(9.13586688858169,18.9169043053388,18.));
#36516=CARTESIAN_POINT('Ctrl Pts',(9.13439956903533,19.0006405223697,0.));
#36517=CARTESIAN_POINT('Ctrl Pts',(9.13439956903533,19.0006405223697,18.));
#36518=CARTESIAN_POINT('Ctrl Pts',(9.13218114462419,19.0845541036965,0.));
#36519=CARTESIAN_POINT('Ctrl Pts',(9.13218114462419,19.0845541036965,18.));
#36520=CARTESIAN_POINT('Ctrl Pts',(9.12921984349375,19.1686380639041,0.));
#36521=CARTESIAN_POINT('Ctrl Pts',(9.12921984349375,19.1686380639041,18.));
#36522=CARTESIAN_POINT('Ctrl Pts',(9.125526627856,19.2528843844341,0.));
#36523=CARTESIAN_POINT('Ctrl Pts',(9.125526627856,19.2528843844341,18.));
#36524=CARTESIAN_POINT('Ctrl Pts',(9.121113479412,19.3372847008483,0.));
#36525=CARTESIAN_POINT('Ctrl Pts',(9.121113479412,19.3372847008483,18.));
#36526=CARTESIAN_POINT('Ctrl Pts',(9.1159915924392,19.4218310275711,0.));
#36527=CARTESIAN_POINT('Ctrl Pts',(9.1159915924392,19.4218310275711,18.));
#36528=CARTESIAN_POINT('Ctrl Pts',(9.11016929611336,19.5065165934577,0.));
#36529=CARTESIAN_POINT('Ctrl Pts',(9.11016929611336,19.5065165934577,18.));
#36530=CARTESIAN_POINT('Ctrl Pts',(9.10365235736465,19.5913357132276,0.));
#36531=CARTESIAN_POINT('Ctrl Pts',(9.10365235736465,19.5913357132276,18.));
#36532=CARTESIAN_POINT('Ctrl Pts',(9.0964449428387,19.6762833927168,0.));
#36533=CARTESIAN_POINT('Ctrl Pts',(9.0964449428387,19.6762833927168,18.));
#36534=CARTESIAN_POINT('Ctrl Pts',(9.08855038355402,19.7613550146978,0.));
#36535=CARTESIAN_POINT('Ctrl Pts',(9.08855038355402,19.7613550146978,18.));
#36536=CARTESIAN_POINT('Ctrl Pts',(9.07997196979668,19.846546013708,0.));
#36537=CARTESIAN_POINT('Ctrl Pts',(9.07997196979668,19.846546013708,18.));
#36538=CARTESIAN_POINT('Ctrl Pts',(9.0707138821585,19.9318514954605,0.));
#36539=CARTESIAN_POINT('Ctrl Pts',(9.0707138821585,19.9318514954605,18.));
#36540=CARTESIAN_POINT('Ctrl Pts',(9.0607810967537,20.0172662790811,0.));
#36541=CARTESIAN_POINT('Ctrl Pts',(9.0607810967537,20.0172662790811,18.));
#36542=CARTESIAN_POINT('Ctrl Pts',(9.0501789809071,20.1027850670435,0.));
#36543=CARTESIAN_POINT('Ctrl Pts',(9.0501789809071,20.1027850670435,18.));
#36544=CARTESIAN_POINT('Ctrl Pts',(9.03891298737031,20.1884025764493,0.));
#36545=CARTESIAN_POINT('Ctrl Pts',(9.03891298737031,20.1884025764493,18.));
#36546=CARTESIAN_POINT('Ctrl Pts',(9.02698833758324,20.2741136736186,0.));
#36547=CARTESIAN_POINT('Ctrl Pts',(9.02698833758324,20.2741136736186,18.));
#36548=CARTESIAN_POINT('Ctrl Pts',(9.01440965049155,20.3599135373691,0.));
#36549=CARTESIAN_POINT('Ctrl Pts',(9.01440965049155,20.3599135373691,18.));
#36550=CARTESIAN_POINT('Ctrl Pts',(9.00118097039517,20.4457976315472,0.));
#36551=CARTESIAN_POINT('Ctrl Pts',(9.00118097039517,20.4457976315472,18.));
#36552=CARTESIAN_POINT('Ctrl Pts',(8.98730595457659,20.5317616031369,0.));
#36553=CARTESIAN_POINT('Ctrl Pts',(8.98730595457659,20.5317616031369,18.));
#36554=CARTESIAN_POINT('Ctrl Pts',(8.97278801890468,20.6178012000199,0.));
#36555=CARTESIAN_POINT('Ctrl Pts',(8.97278801890468,20.6178012000199,18.));
#36556=CARTESIAN_POINT('Ctrl Pts',(8.95763049112623,20.7039121898975,0.));
#36557=CARTESIAN_POINT('Ctrl Pts',(8.95763049112623,20.7039121898975,18.));
#36558=CARTESIAN_POINT('Ctrl Pts',(8.94183680111377,20.7900902537083,0.));
#36559=CARTESIAN_POINT('Ctrl Pts',(8.94183680111377,20.7900902537083,18.));
#36560=CARTESIAN_POINT('Ctrl Pts',(8.92541048738648,20.8763310073304,0.));
#36561=CARTESIAN_POINT('Ctrl Pts',(8.92541048738648,20.8763310073304,18.));
#36562=CARTESIAN_POINT('Ctrl Pts',(8.90835509843285,20.9626300944902,0.));
#36563=CARTESIAN_POINT('Ctrl Pts',(8.90835509843285,20.9626300944902,18.));
#36564=CARTESIAN_POINT('Ctrl Pts',(8.89067412773385,21.0489832630915,0.));
#36565=CARTESIAN_POINT('Ctrl Pts',(8.89067412773385,21.0489832630915,18.));
#36566=CARTESIAN_POINT('Ctrl Pts',(8.87237094640748,21.1353864352374,0.));
#36567=CARTESIAN_POINT('Ctrl Pts',(8.87237094640748,21.1353864352374,18.));
#36568=CARTESIAN_POINT('Ctrl Pts',(8.85344872418155,21.2218358113425,0.));
#36569=CARTESIAN_POINT('Ctrl Pts',(8.85344872418155,21.2218358113425,18.));
#36570=CARTESIAN_POINT('Ctrl Pts',(8.83391042911628,21.3083278326642,0.));
#36571=CARTESIAN_POINT('Ctrl Pts',(8.83391042911628,21.3083278326642,18.));
#36572=CARTESIAN_POINT('Ctrl Pts',(8.81375890120581,21.3948590173441,0.));
#36573=CARTESIAN_POINT('Ctrl Pts',(8.81375890120581,21.3948590173441,18.));
#36574=CARTESIAN_POINT('Ctrl Pts',(8.79299691277858,21.481425822209,0.));
#36575=CARTESIAN_POINT('Ctrl Pts',(8.79299691277858,21.481425822209,18.));
#36576=CARTESIAN_POINT('Ctrl Pts',(8.77162723103298,21.5680245138584,0.));
#36577=CARTESIAN_POINT('Ctrl Pts',(8.77162723103298,21.5680245138584,18.));
#36578=CARTESIAN_POINT('Ctrl Pts',(8.74965270266163,21.6546509866725,0.));
#36579=CARTESIAN_POINT('Ctrl Pts',(8.74965270266163,21.6546509866725,18.));
#36580=CARTESIAN_POINT('Ctrl Pts',(8.72707626956922,21.7413007707864,0.));
#36581=CARTESIAN_POINT('Ctrl Pts',(8.72707626956922,21.7413007707864,18.));
#36582=CARTESIAN_POINT('Ctrl Pts',(8.70390086252203,21.8279693631274,0.));
#36583=CARTESIAN_POINT('Ctrl Pts',(8.70390086252203,21.8279693631274,18.));
#36584=CARTESIAN_POINT('Ctrl Pts',(8.68012932645739,21.9146524902336,0.));
#36585=CARTESIAN_POINT('Ctrl Pts',(8.68012932645739,21.9146524902336,18.));
#36586=CARTESIAN_POINT('Ctrl Pts',(8.6557643376698,22.0013463859623,0.));
#36587=CARTESIAN_POINT('Ctrl Pts',(8.6557643376698,22.0013463859623,18.));
#36588=CARTESIAN_POINT('Ctrl Pts',(8.63080832792612,22.0880480931906,0.));
#36589=CARTESIAN_POINT('Ctrl Pts',(8.63080832792612,22.0880480931906,18.));
#36590=CARTESIAN_POINT('Ctrl Pts',(8.60526341207614,22.1747556651024,0.));
#36591=CARTESIAN_POINT('Ctrl Pts',(8.60526341207614,22.1747556651024,18.));
#36592=CARTESIAN_POINT('Ctrl Pts',(8.57913133085326,22.2614679221213,0.));
#36593=CARTESIAN_POINT('Ctrl Pts',(8.57913133085326,22.2614679221213,18.));
#36594=CARTESIAN_POINT('Ctrl Pts',(8.55775698160722,22.3308410047044,0.));
#36595=CARTESIAN_POINT('Ctrl Pts',(8.55775698160722,22.3308410047044,18.));
#36596=CARTESIAN_POINT('Ctrl Pts',(8.54146295656907,22.3828725698612,0.));
#36597=CARTESIAN_POINT('Ctrl Pts',(8.54146295656907,22.3828725698612,18.));
#36598=CARTESIAN_POINT('Ctrl Pts',(8.53048330625155,22.4175610589877,0.));
#36599=CARTESIAN_POINT('Ctrl Pts',(8.53048330625155,22.4175610589877,18.));
#36600=CARTESIAN_POINT('Ctrl Pts',(8.52496423935285,22.4349054983023,0.));
#36601=CARTESIAN_POINT('Ctrl Pts',(8.52496423935285,22.4349054983023,18.));
#36602=CARTESIAN_POINT('Ctrl Pts',(8.78085409196639,16.6164222996225,0.));
#36603=CARTESIAN_POINT('Ctrl Pts',(8.78817964150686,16.6302847808193,0.));
#36604=CARTESIAN_POINT('Ctrl Pts',(8.80233481798951,16.6582257921024,0.));
#36605=CARTESIAN_POINT('Ctrl Pts',(8.82207984677447,16.7007854423938,0.));
#36606=CARTESIAN_POINT('Ctrl Pts',(8.84558256033742,16.7587634618101,0.));
#36607=CARTESIAN_POINT('Ctrl Pts',(8.87112909692392,16.8329157811062,0.));
#36608=CARTESIAN_POINT('Ctrl Pts',(8.89394614661328,16.908275670167,0.));
#36609=CARTESIAN_POINT('Ctrl Pts',(8.91510993758932,16.9843788566346,0.));
#36610=CARTESIAN_POINT('Ctrl Pts',(8.93538377395243,17.0608897634975,0.));
#36611=CARTESIAN_POINT('Ctrl Pts',(8.95502702208203,17.1376822726252,0.));
#36612=CARTESIAN_POINT('Ctrl Pts',(8.97397941759265,17.2147637614528,0.));
#36613=CARTESIAN_POINT('Ctrl Pts',(8.99199362652257,17.2922207948279,0.));
#36614=CARTESIAN_POINT('Ctrl Pts',(9.00877780436037,17.3701605263553,0.));
#36615=CARTESIAN_POINT('Ctrl Pts',(9.0241575097608,17.4486443043185,0.));
#36616=CARTESIAN_POINT('Ctrl Pts',(9.03814678971601,17.5276582702181,0.));
#36617=CARTESIAN_POINT('Ctrl Pts',(9.05086524971401,17.6071467783263,0.));
#36618=CARTESIAN_POINT('Ctrl Pts',(9.06248904941395,17.6870319618808,0.));
#36619=CARTESIAN_POINT('Ctrl Pts',(9.07319314215026,17.7672369091005,0.));
#36620=CARTESIAN_POINT('Ctrl Pts',(9.08308548608349,17.8477120247758,0.));
#36621=CARTESIAN_POINT('Ctrl Pts',(9.09219303320079,17.9284406141976,0.));
#36622=CARTESIAN_POINT('Ctrl Pts',(9.10049631917583,18.0094249416472,0.));
#36623=CARTESIAN_POINT('Ctrl Pts',(9.10795114540259,18.0906774757189,0.));
#36624=CARTESIAN_POINT('Ctrl Pts',(9.11451347590539,18.1722108451637,0.));
#36625=CARTESIAN_POINT('Ctrl Pts',(9.12016808144599,18.2540262849075,0.));
#36626=CARTESIAN_POINT('Ctrl Pts',(9.12493031448671,18.3361129010289,0.));
#36627=CARTESIAN_POINT('Ctrl Pts',(9.12883240135631,18.4184531695731,0.));
#36628=CARTESIAN_POINT('Ctrl Pts',(9.13191425549883,18.5010266156389,0.));
#36629=CARTESIAN_POINT('Ctrl Pts',(9.13421321934922,18.5838139250423,0.));
#36630=CARTESIAN_POINT('Ctrl Pts',(9.13575227582418,18.6668016710749,0.));
#36631=CARTESIAN_POINT('Ctrl Pts',(9.13654074021147,18.7499820263476,0.));
#36632=CARTESIAN_POINT('Ctrl Pts',(9.13657985367154,18.8333505052874,0.));
#36633=CARTESIAN_POINT('Ctrl Pts',(9.13586688858169,18.9169043053388,0.));
#36634=CARTESIAN_POINT('Ctrl Pts',(9.13439956903533,19.0006405223697,0.));
#36635=CARTESIAN_POINT('Ctrl Pts',(9.13218114462419,19.0845541036965,0.));
#36636=CARTESIAN_POINT('Ctrl Pts',(9.12921984349375,19.1686380639041,0.));
#36637=CARTESIAN_POINT('Ctrl Pts',(9.125526627856,19.2528843844341,0.));
#36638=CARTESIAN_POINT('Ctrl Pts',(9.121113479412,19.3372847008483,0.));
#36639=CARTESIAN_POINT('Ctrl Pts',(9.1159915924392,19.4218310275711,0.));
#36640=CARTESIAN_POINT('Ctrl Pts',(9.11016929611336,19.5065165934577,0.));
#36641=CARTESIAN_POINT('Ctrl Pts',(9.10365235736465,19.5913357132276,0.));
#36642=CARTESIAN_POINT('Ctrl Pts',(9.0964449428387,19.6762833927168,0.));
#36643=CARTESIAN_POINT('Ctrl Pts',(9.08855038355402,19.7613550146978,0.));
#36644=CARTESIAN_POINT('Ctrl Pts',(9.07997196979668,19.846546013708,0.));
#36645=CARTESIAN_POINT('Ctrl Pts',(9.0707138821585,19.9318514954605,0.));
#36646=CARTESIAN_POINT('Ctrl Pts',(9.0607810967537,20.0172662790811,0.));
#36647=CARTESIAN_POINT('Ctrl Pts',(9.0501789809071,20.1027850670435,0.));
#36648=CARTESIAN_POINT('Ctrl Pts',(9.03891298737031,20.1884025764493,0.));
#36649=CARTESIAN_POINT('Ctrl Pts',(9.02698833758324,20.2741136736186,0.));
#36650=CARTESIAN_POINT('Ctrl Pts',(9.01440965049155,20.3599135373691,0.));
#36651=CARTESIAN_POINT('Ctrl Pts',(9.00118097039517,20.4457976315472,0.));
#36652=CARTESIAN_POINT('Ctrl Pts',(8.98730595457659,20.5317616031369,0.));
#36653=CARTESIAN_POINT('Ctrl Pts',(8.97278801890468,20.6178012000199,0.));
#36654=CARTESIAN_POINT('Ctrl Pts',(8.95763049112623,20.7039121898975,0.));
#36655=CARTESIAN_POINT('Ctrl Pts',(8.94183680111377,20.7900902537083,0.));
#36656=CARTESIAN_POINT('Ctrl Pts',(8.92541048738648,20.8763310073304,0.));
#36657=CARTESIAN_POINT('Ctrl Pts',(8.90835509843285,20.9626300944902,0.));
#36658=CARTESIAN_POINT('Ctrl Pts',(8.89067412773385,21.0489832630915,0.));
#36659=CARTESIAN_POINT('Ctrl Pts',(8.87237094640748,21.1353864352374,0.));
#36660=CARTESIAN_POINT('Ctrl Pts',(8.85344872418155,21.2218358113425,0.));
#36661=CARTESIAN_POINT('Ctrl Pts',(8.83391042911628,21.3083278326642,0.));
#36662=CARTESIAN_POINT('Ctrl Pts',(8.81375890120581,21.3948590173441,0.));
#36663=CARTESIAN_POINT('Ctrl Pts',(8.79299691277858,21.481425822209,0.));
#36664=CARTESIAN_POINT('Ctrl Pts',(8.77162723103298,21.5680245138584,0.));
#36665=CARTESIAN_POINT('Ctrl Pts',(8.74965270266163,21.6546509866725,0.));
#36666=CARTESIAN_POINT('Ctrl Pts',(8.72707626956922,21.7413007707864,0.));
#36667=CARTESIAN_POINT('Ctrl Pts',(8.70390086252203,21.8279693631274,0.));
#36668=CARTESIAN_POINT('Ctrl Pts',(8.68012932645739,21.9146524902336,0.));
#36669=CARTESIAN_POINT('Ctrl Pts',(8.6557643376698,22.0013463859623,0.));
#36670=CARTESIAN_POINT('Ctrl Pts',(8.63080832792612,22.0880480931906,0.));
#36671=CARTESIAN_POINT('Ctrl Pts',(8.60015442890614,22.1920971794848,0.));
#36672=CARTESIAN_POINT('Ctrl Pts',(8.57387555634004,22.2788106077804,0.));
#36673=CARTESIAN_POINT('Ctrl Pts',(8.55238412336295,22.3481844703457,0.));
#36674=CARTESIAN_POINT('Ctrl Pts',(8.53600237317213,22.4002166196189,0.));
#36675=CARTESIAN_POINT('Ctrl Pts',(8.52496423935285,22.4349054983023,0.));
#36676=CARTESIAN_POINT('Ctrl Pts',(8.78085409196639,16.6164222996225,15.));
#36677=CARTESIAN_POINT('Ctrl Pts',(8.78817964150686,16.6302847808193,15.));
#36678=CARTESIAN_POINT('Ctrl Pts',(8.80233481798951,16.6582257921024,15.));
#36679=CARTESIAN_POINT('Ctrl Pts',(8.82207984677447,16.7007854423938,15.));
#36680=CARTESIAN_POINT('Ctrl Pts',(8.84558256033742,16.7587634618101,15.));
#36681=CARTESIAN_POINT('Ctrl Pts',(8.87112909692392,16.8329157811062,15.));
#36682=CARTESIAN_POINT('Ctrl Pts',(8.89394614661328,16.908275670167,15.));
#36683=CARTESIAN_POINT('Ctrl Pts',(8.91510993758932,16.9843788566346,15.));
#36684=CARTESIAN_POINT('Ctrl Pts',(8.93538377395243,17.0608897634975,15.));
#36685=CARTESIAN_POINT('Ctrl Pts',(8.95502702208203,17.1376822726252,15.));
#36686=CARTESIAN_POINT('Ctrl Pts',(8.97397941759265,17.2147637614528,15.));
#36687=CARTESIAN_POINT('Ctrl Pts',(8.99199362652257,17.2922207948279,15.));
#36688=CARTESIAN_POINT('Ctrl Pts',(9.00877780436037,17.3701605263553,15.));
#36689=CARTESIAN_POINT('Ctrl Pts',(9.0241575097608,17.4486443043185,15.));
#36690=CARTESIAN_POINT('Ctrl Pts',(9.03814678971601,17.5276582702181,15.));
#36691=CARTESIAN_POINT('Ctrl Pts',(9.05086524971401,17.6071467783263,15.));
#36692=CARTESIAN_POINT('Ctrl Pts',(9.06248904941395,17.6870319618808,15.));
#36693=CARTESIAN_POINT('Ctrl Pts',(9.07319314215026,17.7672369091005,15.));
#36694=CARTESIAN_POINT('Ctrl Pts',(9.08308548608349,17.8477120247758,15.));
#36695=CARTESIAN_POINT('Ctrl Pts',(9.09219303320079,17.9284406141976,15.));
#36696=CARTESIAN_POINT('Ctrl Pts',(9.10049631917583,18.0094249416472,15.));
#36697=CARTESIAN_POINT('Ctrl Pts',(9.10795114540259,18.0906774757189,15.));
#36698=CARTESIAN_POINT('Ctrl Pts',(9.11451347590539,18.1722108451637,15.));
#36699=CARTESIAN_POINT('Ctrl Pts',(9.12016808144599,18.2540262849075,15.));
#36700=CARTESIAN_POINT('Ctrl Pts',(9.12493031448671,18.3361129010289,15.));
#36701=CARTESIAN_POINT('Ctrl Pts',(9.12883240135631,18.4184531695731,15.));
#36702=CARTESIAN_POINT('Ctrl Pts',(9.13191425549883,18.5010266156389,15.));
#36703=CARTESIAN_POINT('Ctrl Pts',(9.13421321934922,18.5838139250423,15.));
#36704=CARTESIAN_POINT('Ctrl Pts',(9.13575227582418,18.6668016710749,15.));
#36705=CARTESIAN_POINT('Ctrl Pts',(9.13654074021147,18.7499820263476,15.));
#36706=CARTESIAN_POINT('Ctrl Pts',(9.13657985367154,18.8333505052874,15.));
#36707=CARTESIAN_POINT('Ctrl Pts',(9.13586688858169,18.9169043053388,15.));
#36708=CARTESIAN_POINT('Ctrl Pts',(9.13439956903533,19.0006405223697,15.));
#36709=CARTESIAN_POINT('Ctrl Pts',(9.13218114462419,19.0845541036965,15.));
#36710=CARTESIAN_POINT('Ctrl Pts',(9.12921984349375,19.1686380639041,15.));
#36711=CARTESIAN_POINT('Ctrl Pts',(9.125526627856,19.2528843844341,15.));
#36712=CARTESIAN_POINT('Ctrl Pts',(9.121113479412,19.3372847008483,15.));
#36713=CARTESIAN_POINT('Ctrl Pts',(9.1159915924392,19.4218310275711,15.));
#36714=CARTESIAN_POINT('Ctrl Pts',(9.11016929611336,19.5065165934577,15.));
#36715=CARTESIAN_POINT('Ctrl Pts',(9.10365235736465,19.5913357132276,15.));
#36716=CARTESIAN_POINT('Ctrl Pts',(9.0964449428387,19.6762833927168,15.));
#36717=CARTESIAN_POINT('Ctrl Pts',(9.08855038355402,19.7613550146978,15.));
#36718=CARTESIAN_POINT('Ctrl Pts',(9.07997196979668,19.846546013708,15.));
#36719=CARTESIAN_POINT('Ctrl Pts',(9.0707138821585,19.9318514954605,15.));
#36720=CARTESIAN_POINT('Ctrl Pts',(9.0607810967537,20.0172662790811,15.));
#36721=CARTESIAN_POINT('Ctrl Pts',(9.0501789809071,20.1027850670435,15.));
#36722=CARTESIAN_POINT('Ctrl Pts',(9.03891298737031,20.1884025764493,15.));
#36723=CARTESIAN_POINT('Ctrl Pts',(9.02698833758324,20.2741136736186,15.));
#36724=CARTESIAN_POINT('Ctrl Pts',(9.01440965049155,20.3599135373691,15.));
#36725=CARTESIAN_POINT('Ctrl Pts',(9.00118097039517,20.4457976315472,15.));
#36726=CARTESIAN_POINT('Ctrl Pts',(8.98730595457659,20.5317616031369,15.));
#36727=CARTESIAN_POINT('Ctrl Pts',(8.97278801890468,20.6178012000199,15.));
#36728=CARTESIAN_POINT('Ctrl Pts',(8.95763049112623,20.7039121898975,15.));
#36729=CARTESIAN_POINT('Ctrl Pts',(8.94183680111377,20.7900902537083,15.));
#36730=CARTESIAN_POINT('Ctrl Pts',(8.92541048738648,20.8763310073304,15.));
#36731=CARTESIAN_POINT('Ctrl Pts',(8.90835509843285,20.9626300944902,15.));
#36732=CARTESIAN_POINT('Ctrl Pts',(8.89067412773385,21.0489832630915,15.));
#36733=CARTESIAN_POINT('Ctrl Pts',(8.87237094640748,21.1353864352374,15.));
#36734=CARTESIAN_POINT('Ctrl Pts',(8.85344872418155,21.2218358113425,15.));
#36735=CARTESIAN_POINT('Ctrl Pts',(8.83391042911628,21.3083278326642,15.));
#36736=CARTESIAN_POINT('Ctrl Pts',(8.81375890120581,21.3948590173441,15.));
#36737=CARTESIAN_POINT('Ctrl Pts',(8.79299691277858,21.481425822209,15.));
#36738=CARTESIAN_POINT('Ctrl Pts',(8.77162723103298,21.5680245138584,15.));
#36739=CARTESIAN_POINT('Ctrl Pts',(8.74965270266163,21.6546509866725,15.));
#36740=CARTESIAN_POINT('Ctrl Pts',(8.72707626956922,21.7413007707864,15.));
#36741=CARTESIAN_POINT('Ctrl Pts',(8.70390086252203,21.8279693631274,15.));
#36742=CARTESIAN_POINT('Ctrl Pts',(8.68012932645739,21.9146524902336,15.));
#36743=CARTESIAN_POINT('Ctrl Pts',(8.6557643376698,22.0013463859623,15.));
#36744=CARTESIAN_POINT('Ctrl Pts',(8.63080832792612,22.0880480931906,15.));
#36745=CARTESIAN_POINT('Ctrl Pts',(8.60015442890614,22.1920971794848,15.));
#36746=CARTESIAN_POINT('Ctrl Pts',(8.57387555634004,22.2788106077804,15.));
#36747=CARTESIAN_POINT('Ctrl Pts',(8.55238412336295,22.3481844703457,15.));
#36748=CARTESIAN_POINT('Ctrl Pts',(8.53600237317213,22.4002166196189,15.));
#36749=CARTESIAN_POINT('Ctrl Pts',(8.52496423935285,22.4349054983023,15.));
#36750=CARTESIAN_POINT('Ctrl Pts',(18.7025042402277,15.040489857191,0.));
#36751=CARTESIAN_POINT('Ctrl Pts',(18.7025042402277,15.040489857191,18.));
#36752=CARTESIAN_POINT('Ctrl Pts',(18.6843032127312,15.0403790752228,0.));
#36753=CARTESIAN_POINT('Ctrl Pts',(18.6843032127312,15.0403790752228,18.));
#36754=CARTESIAN_POINT('Ctrl Pts',(18.6479196005666,15.0401020105546,0.));
#36755=CARTESIAN_POINT('Ctrl Pts',(18.6479196005666,15.0401020105546,18.));
#36756=CARTESIAN_POINT('Ctrl Pts',(18.5933995108277,15.0395199113665,0.));
#36757=CARTESIAN_POINT('Ctrl Pts',(18.5933995108277,15.0395199113665,18.));
#36758=CARTESIAN_POINT('Ctrl Pts',(18.5208167514208,15.0384106640282,0.));
#36759=CARTESIAN_POINT('Ctrl Pts',(18.5208167514208,15.0384106640282,18.));
#36760=CARTESIAN_POINT('Ctrl Pts',(18.4302732371441,15.0364681891201,0.));
#36761=CARTESIAN_POINT('Ctrl Pts',(18.4302732371441,15.0364681891201,18.));
#36762=CARTESIAN_POINT('Ctrl Pts',(18.3399156227477,15.0339687345357,0.));
#36763=CARTESIAN_POINT('Ctrl Pts',(18.3399156227477,15.0339687345357,18.));
#36764=CARTESIAN_POINT('Ctrl Pts',(18.2497455679917,15.0309110092482,0.));
#36765=CARTESIAN_POINT('Ctrl Pts',(18.2497455679917,15.0309110092482,18.));
#36766=CARTESIAN_POINT('Ctrl Pts',(18.1597655779328,15.0272936035154,0.));
#36767=CARTESIAN_POINT('Ctrl Pts',(18.1597655779328,15.0272936035154,18.));
#36768=CARTESIAN_POINT('Ctrl Pts',(18.0699792164192,15.0231151183906,0.));
#36769=CARTESIAN_POINT('Ctrl Pts',(18.0699792164192,15.0231151183906,18.));
#36770=CARTESIAN_POINT('Ctrl Pts',(17.980390892286,15.0183741723687,0.));
#36771=CARTESIAN_POINT('Ctrl Pts',(17.980390892286,15.0183741723687,18.));
#36772=CARTESIAN_POINT('Ctrl Pts',(17.891005548971,15.0130693803259,0.));
#36773=CARTESIAN_POINT('Ctrl Pts',(17.891005548971,15.0130693803259,18.));
#36774=CARTESIAN_POINT('Ctrl Pts',(17.8018283748074,15.0071993464636,0.));
#36775=CARTESIAN_POINT('Ctrl Pts',(17.8018283748074,15.0071993464636,18.));
#36776=CARTESIAN_POINT('Ctrl Pts',(17.7128645299878,15.0007626541286,0.));
#36777=CARTESIAN_POINT('Ctrl Pts',(17.7128645299878,15.0007626541286,18.));
#36778=CARTESIAN_POINT('Ctrl Pts',(17.6241187988652,14.9937578646616,0.));
#36779=CARTESIAN_POINT('Ctrl Pts',(17.6241187988652,14.9937578646616,18.));
#36780=CARTESIAN_POINT('Ctrl Pts',(17.5355955872257,14.9861834999847,0.));
#36781=CARTESIAN_POINT('Ctrl Pts',(17.5355955872257,14.9861834999847,18.));
#36782=CARTESIAN_POINT('Ctrl Pts',(17.4472991215239,14.9780380183576,0.));
#36783=CARTESIAN_POINT('Ctrl Pts',(17.4472991215239,14.9780380183576,18.));
#36784=CARTESIAN_POINT('Ctrl Pts',(17.3592335908103,14.9693197947387,0.));
#36785=CARTESIAN_POINT('Ctrl Pts',(17.3592335908103,14.9693197947387,18.));
#36786=CARTESIAN_POINT('Ctrl Pts',(17.2714032968314,14.9600271060471,0.));
#36787=CARTESIAN_POINT('Ctrl Pts',(17.2714032968314,14.9600271060471,18.));
#36788=CARTESIAN_POINT('Ctrl Pts',(17.1838128327073,14.9501581118289,0.));
#36789=CARTESIAN_POINT('Ctrl Pts',(17.1838128327073,14.9501581118289,18.));
#36790=CARTESIAN_POINT('Ctrl Pts',(17.0964671184813,14.9397108660998,0.));
#36791=CARTESIAN_POINT('Ctrl Pts',(17.0964671184813,14.9397108660998,18.));
#36792=CARTESIAN_POINT('Ctrl Pts',(17.0093712776822,14.9286833603319,0.));
#36793=CARTESIAN_POINT('Ctrl Pts',(17.0093712776822,14.9286833603319,18.));
#36794=CARTESIAN_POINT('Ctrl Pts',(16.9225305499155,14.9170735658747,0.));
#36795=CARTESIAN_POINT('Ctrl Pts',(16.9225305499155,14.9170735658747,18.));
#36796=CARTESIAN_POINT('Ctrl Pts',(16.8359501981915,14.9048794721647,0.));
#36797=CARTESIAN_POINT('Ctrl Pts',(16.8359501981915,14.9048794721647,18.));
#36798=CARTESIAN_POINT('Ctrl Pts',(16.7496353900706,14.8920991518626,0.));
#36799=CARTESIAN_POINT('Ctrl Pts',(16.7496353900706,14.8920991518626,18.));
#36800=CARTESIAN_POINT('Ctrl Pts',(16.6635911790385,14.8787307479454,0.));
#36801=CARTESIAN_POINT('Ctrl Pts',(16.6635911790385,14.8787307479454,18.));
#36802=CARTESIAN_POINT('Ctrl Pts',(16.5778226646614,14.8647723257055,0.));
#36803=CARTESIAN_POINT('Ctrl Pts',(16.5778226646614,14.8647723257055,18.));
#36804=CARTESIAN_POINT('Ctrl Pts',(16.492335117066,14.8502217520165,0.));
#36805=CARTESIAN_POINT('Ctrl Pts',(16.492335117066,14.8502217520165,18.));
#36806=CARTESIAN_POINT('Ctrl Pts',(16.4071341001481,14.8350765822692,0.));
#36807=CARTESIAN_POINT('Ctrl Pts',(16.4071341001481,14.8350765822692,18.));
#36808=CARTESIAN_POINT('Ctrl Pts',(16.3222256264574,14.8193339134125,0.));
#36809=CARTESIAN_POINT('Ctrl Pts',(16.3222256264574,14.8193339134125,18.));
#36810=CARTESIAN_POINT('Ctrl Pts',(16.2376161919272,14.8029903659562,0.));
#36811=CARTESIAN_POINT('Ctrl Pts',(16.2376161919272,14.8029903659562,18.));
#36812=CARTESIAN_POINT('Ctrl Pts',(16.1533125058853,14.7860423865308,0.));
#36813=CARTESIAN_POINT('Ctrl Pts',(16.1533125058853,14.7860423865308,18.));
#36814=CARTESIAN_POINT('Ctrl Pts',(16.0693212651732,14.7684865075326,0.));
#36815=CARTESIAN_POINT('Ctrl Pts',(16.0693212651732,14.7684865075326,18.));
#36816=CARTESIAN_POINT('Ctrl Pts',(15.9856489347991,14.7503195973741,0.));
#36817=CARTESIAN_POINT('Ctrl Pts',(15.9856489347991,14.7503195973741,18.));
#36818=CARTESIAN_POINT('Ctrl Pts',(15.9023014613802,14.7315391924939,0.));
#36819=CARTESIAN_POINT('Ctrl Pts',(15.9023014613802,14.7315391924939,18.));
#36820=CARTESIAN_POINT('Ctrl Pts',(15.8192842036838,14.7121435744495,0.));
#36821=CARTESIAN_POINT('Ctrl Pts',(15.8192842036838,14.7121435744495,18.));
#36822=CARTESIAN_POINT('Ctrl Pts',(15.7366025822956,14.692131002056,0.));
#36823=CARTESIAN_POINT('Ctrl Pts',(15.7366025822956,14.692131002056,18.));
#36824=CARTESIAN_POINT('Ctrl Pts',(15.6542626345121,14.6714990558793,0.));
#36825=CARTESIAN_POINT('Ctrl Pts',(15.6542626345121,14.6714990558793,18.));
#36826=CARTESIAN_POINT('Ctrl Pts',(15.5722715494357,14.6502440080911,0.));
#36827=CARTESIAN_POINT('Ctrl Pts',(15.5722715494357,14.6502440080911,18.));
#36828=CARTESIAN_POINT('Ctrl Pts',(15.4906383406647,14.6283600295736,0.));
#36829=CARTESIAN_POINT('Ctrl Pts',(15.4906383406647,14.6283600295736,18.));
#36830=CARTESIAN_POINT('Ctrl Pts',(15.4093740621548,14.6058389416146,0.));
#36831=CARTESIAN_POINT('Ctrl Pts',(15.4093740621548,14.6058389416146,18.));
#36832=CARTESIAN_POINT('Ctrl Pts',(15.3284903715086,14.5826719336929,0.));
#36833=CARTESIAN_POINT('Ctrl Pts',(15.3284903715086,14.5826719336929,18.));
#36834=CARTESIAN_POINT('Ctrl Pts',(15.2479982823383,14.5588510579962,0.));
#36835=CARTESIAN_POINT('Ctrl Pts',(15.2479982823383,14.5588510579962,18.));
#36836=CARTESIAN_POINT('Ctrl Pts',(15.1679069808052,14.534370647705,0.));
#36837=CARTESIAN_POINT('Ctrl Pts',(15.1679069808052,14.534370647705,18.));
#36838=CARTESIAN_POINT('Ctrl Pts',(15.0882222764759,14.5092291736391,0.));
#36839=CARTESIAN_POINT('Ctrl Pts',(15.0882222764759,14.5092291736391,18.));
#36840=CARTESIAN_POINT('Ctrl Pts',(15.0089462280505,14.4834296977405,0.));
#36841=CARTESIAN_POINT('Ctrl Pts',(15.0089462280505,14.4834296977405,18.));
#36842=CARTESIAN_POINT('Ctrl Pts',(14.9300806580357,14.4569756801697,0.));
#36843=CARTESIAN_POINT('Ctrl Pts',(14.9300806580357,14.4569756801697,18.));
#36844=CARTESIAN_POINT('Ctrl Pts',(14.8516302160049,14.4298673266313,0.));
#36845=CARTESIAN_POINT('Ctrl Pts',(14.8516302160049,14.4298673266313,18.));
#36846=CARTESIAN_POINT('Ctrl Pts',(14.7736052248294,14.4020981965564,0.));
#36847=CARTESIAN_POINT('Ctrl Pts',(14.7736052248294,14.4020981965564,18.));
#36848=CARTESIAN_POINT('Ctrl Pts',(14.6960255561799,14.3736505809735,0.));
#36849=CARTESIAN_POINT('Ctrl Pts',(14.6960255561799,14.3736505809735,18.));
#36850=CARTESIAN_POINT('Ctrl Pts',(14.6189211183837,14.3444949335274,0.));
#36851=CARTESIAN_POINT('Ctrl Pts',(14.6189211183837,14.3444949335274,18.));
#36852=CARTESIAN_POINT('Ctrl Pts',(14.5423237181615,14.3145996213697,0.));
#36853=CARTESIAN_POINT('Ctrl Pts',(14.5423237181615,14.3145996213697,18.));
#36854=CARTESIAN_POINT('Ctrl Pts',(14.4662599802682,14.2839394106401,0.));
#36855=CARTESIAN_POINT('Ctrl Pts',(14.4662599802682,14.2839394106401,18.));
#36856=CARTESIAN_POINT('Ctrl Pts',(14.3907450096103,14.2525030666863,0.));
#36857=CARTESIAN_POINT('Ctrl Pts',(14.3907450096103,14.2525030666863,18.));
#36858=CARTESIAN_POINT('Ctrl Pts',(14.3157729256101,14.2203046917613,0.));
#36859=CARTESIAN_POINT('Ctrl Pts',(14.3157729256101,14.2203046917613,18.));
#36860=CARTESIAN_POINT('Ctrl Pts',(14.2413181097468,14.1873822640681,0.));
#36861=CARTESIAN_POINT('Ctrl Pts',(14.2413181097468,14.1873822640681,18.));
#36862=CARTESIAN_POINT('Ctrl Pts',(14.1673550455622,14.1537739659715,0.));
#36863=CARTESIAN_POINT('Ctrl Pts',(14.1673550455622,14.1537739659715,18.));
#36864=CARTESIAN_POINT('Ctrl Pts',(14.0938755647891,14.1194976094444,0.));
#36865=CARTESIAN_POINT('Ctrl Pts',(14.0938755647891,14.1194976094444,18.));
#36866=CARTESIAN_POINT('Ctrl Pts',(14.0209038736616,14.0845327205726,0.));
#36867=CARTESIAN_POINT('Ctrl Pts',(14.0209038736616,14.0845327205726,18.));
#36868=CARTESIAN_POINT('Ctrl Pts',(13.9485205009332,14.0487919508068,0.));
#36869=CARTESIAN_POINT('Ctrl Pts',(13.9485205009332,14.0487919508068,18.));
#36870=CARTESIAN_POINT('Ctrl Pts',(13.876852657608,14.0121326766855,0.));
#36871=CARTESIAN_POINT('Ctrl Pts',(13.876852657608,14.0121326766855,18.));
#36872=CARTESIAN_POINT('Ctrl Pts',(13.806028835706,13.9744114225699,0.));
#36873=CARTESIAN_POINT('Ctrl Pts',(13.806028835706,13.9744114225699,18.));
#36874=CARTESIAN_POINT('Ctrl Pts',(13.7361389175879,13.9355316323567,0.));
#36875=CARTESIAN_POINT('Ctrl Pts',(13.7361389175879,13.9355316323567,18.));
#36876=CARTESIAN_POINT('Ctrl Pts',(13.6672004242289,13.8954842290745,0.));
#36877=CARTESIAN_POINT('Ctrl Pts',(13.6672004242289,13.8954842290745,18.));
#36878=CARTESIAN_POINT('Ctrl Pts',(13.5991011046042,13.854416158639,0.));
#36879=CARTESIAN_POINT('Ctrl Pts',(13.5991011046042,13.854416158639,18.));
#36880=CARTESIAN_POINT('Ctrl Pts',(13.5316488646659,13.8125718693898,0.));
#36881=CARTESIAN_POINT('Ctrl Pts',(13.5316488646659,13.8125718693898,18.));
#36882=CARTESIAN_POINT('Ctrl Pts',(13.4646849459541,13.7701598398937,0.));
#36883=CARTESIAN_POINT('Ctrl Pts',(13.4646849459541,13.7701598398937,18.));
#36884=CARTESIAN_POINT('Ctrl Pts',(13.3981837093919,13.7272351052346,0.));
#36885=CARTESIAN_POINT('Ctrl Pts',(13.3981837093919,13.7272351052346,18.));
#36886=CARTESIAN_POINT('Ctrl Pts',(13.332345249068,13.6835899659728,0.));
#36887=CARTESIAN_POINT('Ctrl Pts',(13.332345249068,13.6835899659728,18.));
#36888=CARTESIAN_POINT('Ctrl Pts',(13.267724591625,13.6386021757691,0.));
#36889=CARTESIAN_POINT('Ctrl Pts',(13.267724591625,13.6386021757691,18.));
#36890=CARTESIAN_POINT('Ctrl Pts',(13.2050958591127,13.5913916488449,0.));
#36891=CARTESIAN_POINT('Ctrl Pts',(13.2050958591127,13.5913916488449,18.));
#36892=CARTESIAN_POINT('Ctrl Pts',(13.1572182238498,13.5511230466604,0.));
#36893=CARTESIAN_POINT('Ctrl Pts',(13.1572182238498,13.5511230466604,18.));
#36894=CARTESIAN_POINT('Ctrl Pts',(13.1228431405579,13.5191927531554,0.));
#36895=CARTESIAN_POINT('Ctrl Pts',(13.1228431405579,13.5191927531554,18.));
#36896=CARTESIAN_POINT('Ctrl Pts',(13.1006438497967,13.4970961329957,0.));
#36897=CARTESIAN_POINT('Ctrl Pts',(13.1006438497967,13.4970961329957,18.));
#36898=CARTESIAN_POINT('Ctrl Pts',(13.0897235660237,13.4858453790958,0.));
#36899=CARTESIAN_POINT('Ctrl Pts',(13.0897235660237,13.4858453790958,18.));
#36900=CARTESIAN_POINT('',(18.7025042402277,15.040489857191,0.));
#36901=CARTESIAN_POINT('Ctrl Pts',(13.0897235660237,13.4858453790958,0.));
#36902=CARTESIAN_POINT('Ctrl Pts',(13.1006438497967,13.4970961329957,0.));
#36903=CARTESIAN_POINT('Ctrl Pts',(13.1228431405579,13.5191927531554,0.));
#36904=CARTESIAN_POINT('Ctrl Pts',(13.1572182238498,13.5511230466604,0.));
#36905=CARTESIAN_POINT('Ctrl Pts',(13.2050958591127,13.5913916488449,0.));
#36906=CARTESIAN_POINT('Ctrl Pts',(13.267724591625,13.6386021757691,0.));
#36907=CARTESIAN_POINT('Ctrl Pts',(13.332345249068,13.6835899659728,0.));
#36908=CARTESIAN_POINT('Ctrl Pts',(13.3981837093919,13.7272351052346,0.));
#36909=CARTESIAN_POINT('Ctrl Pts',(13.4646849459541,13.7701598398937,0.));
#36910=CARTESIAN_POINT('Ctrl Pts',(13.5316488646659,13.8125718693898,0.));
#36911=CARTESIAN_POINT('Ctrl Pts',(13.5991011046042,13.854416158639,0.));
#36912=CARTESIAN_POINT('Ctrl Pts',(13.6672004242289,13.8954842290745,0.));
#36913=CARTESIAN_POINT('Ctrl Pts',(13.7361389175879,13.9355316323567,0.));
#36914=CARTESIAN_POINT('Ctrl Pts',(13.806028835706,13.9744114225699,0.));
#36915=CARTESIAN_POINT('Ctrl Pts',(13.876852657608,14.0121326766855,0.));
#36916=CARTESIAN_POINT('Ctrl Pts',(13.9485205009332,14.0487919508068,0.));
#36917=CARTESIAN_POINT('Ctrl Pts',(14.0209038736616,14.0845327205726,0.));
#36918=CARTESIAN_POINT('Ctrl Pts',(14.0938755647891,14.1194976094444,0.));
#36919=CARTESIAN_POINT('Ctrl Pts',(14.1673550455622,14.1537739659715,0.));
#36920=CARTESIAN_POINT('Ctrl Pts',(14.2413181097468,14.1873822640681,0.));
#36921=CARTESIAN_POINT('Ctrl Pts',(14.3157729256101,14.2203046917613,0.));
#36922=CARTESIAN_POINT('Ctrl Pts',(14.3907450096103,14.2525030666863,0.));
#36923=CARTESIAN_POINT('Ctrl Pts',(14.4662599802682,14.2839394106401,0.));
#36924=CARTESIAN_POINT('Ctrl Pts',(14.5423237181615,14.3145996213697,0.));
#36925=CARTESIAN_POINT('Ctrl Pts',(14.6189211183837,14.3444949335274,0.));
#36926=CARTESIAN_POINT('Ctrl Pts',(14.6960255561799,14.3736505809735,0.));
#36927=CARTESIAN_POINT('Ctrl Pts',(14.7736052248294,14.4020981965564,0.));
#36928=CARTESIAN_POINT('Ctrl Pts',(14.8516302160049,14.4298673266313,0.));
#36929=CARTESIAN_POINT('Ctrl Pts',(14.9300806580357,14.4569756801697,0.));
#36930=CARTESIAN_POINT('Ctrl Pts',(15.0089462280505,14.4834296977405,0.));
#36931=CARTESIAN_POINT('Ctrl Pts',(15.0882222764759,14.5092291736391,0.));
#36932=CARTESIAN_POINT('Ctrl Pts',(15.1679069808052,14.534370647705,0.));
#36933=CARTESIAN_POINT('Ctrl Pts',(15.2479982823383,14.5588510579962,0.));
#36934=CARTESIAN_POINT('Ctrl Pts',(15.3284903715086,14.5826719336929,0.));
#36935=CARTESIAN_POINT('Ctrl Pts',(15.4093740621548,14.6058389416146,0.));
#36936=CARTESIAN_POINT('Ctrl Pts',(15.4906383406647,14.6283600295736,0.));
#36937=CARTESIAN_POINT('Ctrl Pts',(15.5722715494357,14.6502440080911,0.));
#36938=CARTESIAN_POINT('Ctrl Pts',(15.6542626345121,14.6714990558793,0.));
#36939=CARTESIAN_POINT('Ctrl Pts',(15.7366025822956,14.692131002056,0.));
#36940=CARTESIAN_POINT('Ctrl Pts',(15.8192842036838,14.7121435744495,0.));
#36941=CARTESIAN_POINT('Ctrl Pts',(15.9023014613802,14.7315391924939,0.));
#36942=CARTESIAN_POINT('Ctrl Pts',(15.9856489347991,14.7503195973741,0.));
#36943=CARTESIAN_POINT('Ctrl Pts',(16.0693212651732,14.7684865075326,0.));
#36944=CARTESIAN_POINT('Ctrl Pts',(16.1533125058853,14.7860423865308,0.));
#36945=CARTESIAN_POINT('Ctrl Pts',(16.2376161919272,14.8029903659562,0.));
#36946=CARTESIAN_POINT('Ctrl Pts',(16.3222256264574,14.8193339134125,0.));
#36947=CARTESIAN_POINT('Ctrl Pts',(16.4071341001481,14.8350765822692,0.));
#36948=CARTESIAN_POINT('Ctrl Pts',(16.492335117066,14.8502217520165,0.));
#36949=CARTESIAN_POINT('Ctrl Pts',(16.5778226646614,14.8647723257055,0.));
#36950=CARTESIAN_POINT('Ctrl Pts',(16.6635911790385,14.8787307479454,0.));
#36951=CARTESIAN_POINT('Ctrl Pts',(16.7496353900706,14.8920991518626,0.));
#36952=CARTESIAN_POINT('Ctrl Pts',(16.8359501981915,14.9048794721647,0.));
#36953=CARTESIAN_POINT('Ctrl Pts',(16.9225305499155,14.9170735658747,0.));
#36954=CARTESIAN_POINT('Ctrl Pts',(17.0093712776822,14.9286833603319,0.));
#36955=CARTESIAN_POINT('Ctrl Pts',(17.0964671184813,14.9397108660998,0.));
#36956=CARTESIAN_POINT('Ctrl Pts',(17.1838128327073,14.9501581118289,0.));
#36957=CARTESIAN_POINT('Ctrl Pts',(17.2714032968314,14.9600271060471,0.));
#36958=CARTESIAN_POINT('Ctrl Pts',(17.3592335908103,14.9693197947387,0.));
#36959=CARTESIAN_POINT('Ctrl Pts',(17.4472991215239,14.9780380183576,0.));
#36960=CARTESIAN_POINT('Ctrl Pts',(17.5355955872257,14.9861834999847,0.));
#36961=CARTESIAN_POINT('Ctrl Pts',(17.6241187988652,14.9937578646616,0.));
#36962=CARTESIAN_POINT('Ctrl Pts',(17.7128645299878,15.0007626541286,0.));
#36963=CARTESIAN_POINT('Ctrl Pts',(17.8018283748074,15.0071993464636,0.));
#36964=CARTESIAN_POINT('Ctrl Pts',(17.891005548971,15.0130693803259,0.));
#36965=CARTESIAN_POINT('Ctrl Pts',(17.980390892286,15.0183741723687,0.));
#36966=CARTESIAN_POINT('Ctrl Pts',(18.0699792164192,15.0231151183906,0.));
#36967=CARTESIAN_POINT('Ctrl Pts',(18.1597655779328,15.0272936035154,0.));
#36968=CARTESIAN_POINT('Ctrl Pts',(18.2497455679917,15.0309110092482,0.));
#36969=CARTESIAN_POINT('Ctrl Pts',(18.3399156227477,15.0339687345357,0.));
#36970=CARTESIAN_POINT('Ctrl Pts',(18.4483447600234,15.036968080037,0.));
#36971=CARTESIAN_POINT('Ctrl Pts',(18.5389347492702,15.038771310026,0.));
#36972=CARTESIAN_POINT('Ctrl Pts',(18.6115544313469,15.0397694451467,0.));
#36973=CARTESIAN_POINT('Ctrl Pts',(18.6661021851765,15.0402682932586,0.));
#36974=CARTESIAN_POINT('Ctrl Pts',(18.7025042402277,15.040489857191,0.));
#36975=CARTESIAN_POINT('',(18.7025042402277,15.040489857191,15.));
#36976=CARTESIAN_POINT('Ctrl Pts',(18.7025042402277,15.040489857191,15.));
#36977=CARTESIAN_POINT('Ctrl Pts',(18.6843032127312,15.0403790752228,15.));
#36978=CARTESIAN_POINT('Ctrl Pts',(18.6479196005666,15.0401020105546,15.));
#36979=CARTESIAN_POINT('Ctrl Pts',(18.5933995108277,15.0395199113665,15.));
#36980=CARTESIAN_POINT('Ctrl Pts',(18.5208167514208,15.0384106640282,15.));
#36981=CARTESIAN_POINT('Ctrl Pts',(18.4302732371441,15.0364681891201,15.));
#36982=CARTESIAN_POINT('Ctrl Pts',(18.3399156227477,15.0339687345357,15.));
#36983=CARTESIAN_POINT('Ctrl Pts',(18.2497455679917,15.0309110092482,15.));
#36984=CARTESIAN_POINT('Ctrl Pts',(18.1597655779328,15.0272936035154,15.));
#36985=CARTESIAN_POINT('Ctrl Pts',(18.0699792164192,15.0231151183906,15.));
#36986=CARTESIAN_POINT('Ctrl Pts',(17.980390892286,15.0183741723687,15.));
#36987=CARTESIAN_POINT('Ctrl Pts',(17.891005548971,15.0130693803259,15.));
#36988=CARTESIAN_POINT('Ctrl Pts',(17.8018283748074,15.0071993464636,15.));
#36989=CARTESIAN_POINT('Ctrl Pts',(17.7128645299878,15.0007626541286,15.));
#36990=CARTESIAN_POINT('Ctrl Pts',(17.6241187988652,14.9937578646616,15.));
#36991=CARTESIAN_POINT('Ctrl Pts',(17.5355955872257,14.9861834999847,15.));
#36992=CARTESIAN_POINT('Ctrl Pts',(17.4472991215239,14.9780380183576,15.));
#36993=CARTESIAN_POINT('Ctrl Pts',(17.3592335908103,14.9693197947387,15.));
#36994=CARTESIAN_POINT('Ctrl Pts',(17.2714032968314,14.9600271060471,15.));
#36995=CARTESIAN_POINT('Ctrl Pts',(17.1838128327073,14.9501581118289,15.));
#36996=CARTESIAN_POINT('Ctrl Pts',(17.0964671184813,14.9397108660998,15.));
#36997=CARTESIAN_POINT('Ctrl Pts',(17.0093712776822,14.9286833603319,15.));
#36998=CARTESIAN_POINT('Ctrl Pts',(16.9225305499155,14.9170735658747,15.));
#36999=CARTESIAN_POINT('Ctrl Pts',(16.8359501981915,14.9048794721647,15.));
#37000=CARTESIAN_POINT('Ctrl Pts',(16.7496353900706,14.8920991518626,15.));
#37001=CARTESIAN_POINT('Ctrl Pts',(16.6635911790385,14.8787307479454,15.));
#37002=CARTESIAN_POINT('Ctrl Pts',(16.5778226646614,14.8647723257055,15.));
#37003=CARTESIAN_POINT('Ctrl Pts',(16.492335117066,14.8502217520165,15.));
#37004=CARTESIAN_POINT('Ctrl Pts',(16.4071341001481,14.8350765822692,15.));
#37005=CARTESIAN_POINT('Ctrl Pts',(16.3222256264574,14.8193339134125,15.));
#37006=CARTESIAN_POINT('Ctrl Pts',(16.2376161919272,14.8029903659562,15.));
#37007=CARTESIAN_POINT('Ctrl Pts',(16.1533125058853,14.7860423865308,15.));
#37008=CARTESIAN_POINT('Ctrl Pts',(16.0693212651732,14.7684865075326,15.));
#37009=CARTESIAN_POINT('Ctrl Pts',(15.9856489347991,14.7503195973741,15.));
#37010=CARTESIAN_POINT('Ctrl Pts',(15.9023014613802,14.7315391924939,15.));
#37011=CARTESIAN_POINT('Ctrl Pts',(15.8192842036838,14.7121435744495,15.));
#37012=CARTESIAN_POINT('Ctrl Pts',(15.7366025822956,14.692131002056,15.));
#37013=CARTESIAN_POINT('Ctrl Pts',(15.6542626345121,14.6714990558793,15.));
#37014=CARTESIAN_POINT('Ctrl Pts',(15.5722715494357,14.6502440080911,15.));
#37015=CARTESIAN_POINT('Ctrl Pts',(15.4906383406647,14.6283600295736,15.));
#37016=CARTESIAN_POINT('Ctrl Pts',(15.4093740621548,14.6058389416146,15.));
#37017=CARTESIAN_POINT('Ctrl Pts',(15.3284903715086,14.5826719336929,15.));
#37018=CARTESIAN_POINT('Ctrl Pts',(15.2479982823383,14.5588510579962,15.));
#37019=CARTESIAN_POINT('Ctrl Pts',(15.1679069808052,14.534370647705,15.));
#37020=CARTESIAN_POINT('Ctrl Pts',(15.0882222764759,14.5092291736391,15.));
#37021=CARTESIAN_POINT('Ctrl Pts',(15.0089462280505,14.4834296977405,15.));
#37022=CARTESIAN_POINT('Ctrl Pts',(14.9300806580357,14.4569756801697,15.));
#37023=CARTESIAN_POINT('Ctrl Pts',(14.8516302160049,14.4298673266313,15.));
#37024=CARTESIAN_POINT('Ctrl Pts',(14.7736052248294,14.4020981965564,15.));
#37025=CARTESIAN_POINT('Ctrl Pts',(14.6960255561799,14.3736505809735,15.));
#37026=CARTESIAN_POINT('Ctrl Pts',(14.6189211183837,14.3444949335274,15.));
#37027=CARTESIAN_POINT('Ctrl Pts',(14.5423237181615,14.3145996213697,15.));
#37028=CARTESIAN_POINT('Ctrl Pts',(14.4662599802682,14.2839394106401,15.));
#37029=CARTESIAN_POINT('Ctrl Pts',(14.3907450096103,14.2525030666863,15.));
#37030=CARTESIAN_POINT('Ctrl Pts',(14.3157729256101,14.2203046917613,15.));
#37031=CARTESIAN_POINT('Ctrl Pts',(14.2413181097468,14.1873822640681,15.));
#37032=CARTESIAN_POINT('Ctrl Pts',(14.1673550455622,14.1537739659715,15.));
#37033=CARTESIAN_POINT('Ctrl Pts',(14.0938755647891,14.1194976094444,15.));
#37034=CARTESIAN_POINT('Ctrl Pts',(14.0209038736616,14.0845327205726,15.));
#37035=CARTESIAN_POINT('Ctrl Pts',(13.9485205009332,14.0487919508068,15.));
#37036=CARTESIAN_POINT('Ctrl Pts',(13.876852657608,14.0121326766855,15.));
#37037=CARTESIAN_POINT('Ctrl Pts',(13.806028835706,13.9744114225699,15.));
#37038=CARTESIAN_POINT('Ctrl Pts',(13.7361389175879,13.9355316323567,15.));
#37039=CARTESIAN_POINT('Ctrl Pts',(13.6672004242289,13.8954842290745,15.));
#37040=CARTESIAN_POINT('Ctrl Pts',(13.5991011046042,13.854416158639,15.));
#37041=CARTESIAN_POINT('Ctrl Pts',(13.5316488646659,13.8125718693898,15.));
#37042=CARTESIAN_POINT('Ctrl Pts',(13.4646849459541,13.7701598398937,15.));
#37043=CARTESIAN_POINT('Ctrl Pts',(13.3981837093919,13.7272351052346,15.));
#37044=CARTESIAN_POINT('Ctrl Pts',(13.332345249068,13.6835899659728,15.));
#37045=CARTESIAN_POINT('Ctrl Pts',(13.267724591625,13.6386021757691,15.));
#37046=CARTESIAN_POINT('Ctrl Pts',(13.2050958591127,13.5913916488449,15.));
#37047=CARTESIAN_POINT('Ctrl Pts',(13.1572182238498,13.5511230466604,15.));
#37048=CARTESIAN_POINT('Ctrl Pts',(13.1228431405579,13.5191927531554,15.));
#37049=CARTESIAN_POINT('Ctrl Pts',(13.1006438497967,13.4970961329957,15.));
#37050=CARTESIAN_POINT('Ctrl Pts',(13.0897235660237,13.4858453790958,15.));
#37051=CARTESIAN_POINT('',(18.7025042402277,15.040489857191,0.));
#37052=CARTESIAN_POINT('Origin',(9.34524724197225E-14,6.78114261146376E-14,
0.));
#37053=CARTESIAN_POINT('',(20.0837475345526,13.1393715591102,0.));
#37054=CARTESIAN_POINT('Origin',(9.34524724197225E-14,6.78114261146376E-14,
0.));
#37055=CARTESIAN_POINT('',(20.0837475345526,13.1393715591102,15.));
#37056=CARTESIAN_POINT('Origin',(9.34524724197225E-14,6.78114261146376E-14,
15.));
#37057=CARTESIAN_POINT('',(20.0837475345526,13.1393715591102,0.));
#37058=CARTESIAN_POINT('Ctrl Pts',(16.8707481591095,8.28171148831561,0.));
#37059=CARTESIAN_POINT('Ctrl Pts',(16.8707481591095,8.28171148831561,18.));
#37060=CARTESIAN_POINT('Ctrl Pts',(16.8848228151885,8.28862062120315,0.));
#37061=CARTESIAN_POINT('Ctrl Pts',(16.8848228151885,8.28862062120315,18.));
#37062=CARTESIAN_POINT('Ctrl Pts',(16.9126979078877,8.30290517019115,0.));
#37063=CARTESIAN_POINT('Ctrl Pts',(16.9126979078877,8.30290517019115,18.));
#37064=CARTESIAN_POINT('Ctrl Pts',(16.9536879065132,8.32573081382562,0.));
#37065=CARTESIAN_POINT('Ctrl Pts',(16.9536879065132,8.32573081382562,18.));
#37066=CARTESIAN_POINT('Ctrl Pts',(17.0067806259695,8.35882146841243,0.));
#37067=CARTESIAN_POINT('Ctrl Pts',(17.0067806259695,8.35882146841243,18.));
#37068=CARTESIAN_POINT('Ctrl Pts',(17.071033847921,8.40379607744266,0.));
#37069=CARTESIAN_POINT('Ctrl Pts',(17.071033847921,8.40379607744266,18.));
#37070=CARTESIAN_POINT('Ctrl Pts',(17.1337886602855,8.45135198307876,0.));
#37071=CARTESIAN_POINT('Ctrl Pts',(17.1337886602855,8.45135198307876,18.));
#37072=CARTESIAN_POINT('Ctrl Pts',(17.1956428575086,8.50048099003882,0.));
#37073=CARTESIAN_POINT('Ctrl Pts',(17.1956428575086,8.50048099003882,18.));
#37074=CARTESIAN_POINT('Ctrl Pts',(17.2570167183611,8.55046295192433,0.));
#37075=CARTESIAN_POINT('Ctrl Pts',(17.2570167183611,8.55046295192433,18.));
#37076=CARTESIAN_POINT('Ctrl Pts',(17.3180459442745,8.60104338529165,0.));
#37077=CARTESIAN_POINT('Ctrl Pts',(17.3180459442745,8.60104338529165,18.));
#37078=CARTESIAN_POINT('Ctrl Pts',(17.3786861166843,8.65226368112816,0.));
#37079=CARTESIAN_POINT('Ctrl Pts',(17.3786861166843,8.65226368112816,18.));
#37080=CARTESIAN_POINT('Ctrl Pts',(17.438788019753,8.70433925112174,0.));
#37081=CARTESIAN_POINT('Ctrl Pts',(17.438788019753,8.70433925112174,18.));
#37082=CARTESIAN_POINT('Ctrl Pts',(17.4981785296199,8.75752832625954,0.));
#37083=CARTESIAN_POINT('Ctrl Pts',(17.4981785296199,8.75752832625954,18.));
#37084=CARTESIAN_POINT('Ctrl Pts',(17.5567525798882,8.8119830723955,0.));
#37085=CARTESIAN_POINT('Ctrl Pts',(17.5567525798882,8.8119830723955,18.));
#37086=CARTESIAN_POINT('Ctrl Pts',(17.614513388992,8.86768402115343,0.));
#37087=CARTESIAN_POINT('Ctrl Pts',(17.614513388992,8.86768402115343,18.));
#37088=CARTESIAN_POINT('Ctrl Pts',(17.6715250120654,8.92451585185175,0.));
#37089=CARTESIAN_POINT('Ctrl Pts',(17.6715250120654,8.92451585185175,18.));
#37090=CARTESIAN_POINT('Ctrl Pts',(17.7278841963319,8.98231202490685,0.));
#37091=CARTESIAN_POINT('Ctrl Pts',(17.7278841963319,8.98231202490685,18.));
#37092=CARTESIAN_POINT('Ctrl Pts',(17.7836872744016,9.04090748239097,0.));
#37093=CARTESIAN_POINT('Ctrl Pts',(17.7836872744016,9.04090748239097,18.));
#37094=CARTESIAN_POINT('Ctrl Pts',(17.8389924349283,9.10019864472208,0.));
#37095=CARTESIAN_POINT('Ctrl Pts',(17.8389924349283,9.10019864472208,18.));
#37096=CARTESIAN_POINT('Ctrl Pts',(17.8938116696237,9.16015616361609,0.));
#37097=CARTESIAN_POINT('Ctrl Pts',(17.8938116696237,9.16015616361609,18.));
#37098=CARTESIAN_POINT('Ctrl Pts',(17.9481305624284,9.22079331175917,0.));
#37099=CARTESIAN_POINT('Ctrl Pts',(17.9481305624284,9.22079331175917,18.));
#37100=CARTESIAN_POINT('Ctrl Pts',(18.0019206847747,9.2821461557447,0.));
#37101=CARTESIAN_POINT('Ctrl Pts',(18.0019206847747,9.2821461557447,18.));
#37102=CARTESIAN_POINT('Ctrl Pts',(18.0551538338035,9.34425079614396,0.));
#37103=CARTESIAN_POINT('Ctrl Pts',(18.0551538338035,9.34425079614396,18.));
#37104=CARTESIAN_POINT('Ctrl Pts',(18.1078184146735,9.40711718355464,0.));
#37105=CARTESIAN_POINT('Ctrl Pts',(18.1078184146735,9.40711718355464,18.));
#37106=CARTESIAN_POINT('Ctrl Pts',(18.1599204445014,9.47072748065831,0.));
#37107=CARTESIAN_POINT('Ctrl Pts',(18.1599204445014,9.47072748065831,18.));
#37108=CARTESIAN_POINT('Ctrl Pts',(18.2114756946126,9.53504856811685,0.));
#37109=CARTESIAN_POINT('Ctrl Pts',(18.2114756946126,9.53504856811685,18.));
#37110=CARTESIAN_POINT('Ctrl Pts',(18.2625044208165,9.60004042085347,0.));
#37111=CARTESIAN_POINT('Ctrl Pts',(18.2625044208165,9.60004042085347,18.));
#37112=CARTESIAN_POINT('Ctrl Pts',(18.3130254811852,9.66566546403259,0.));
#37113=CARTESIAN_POINT('Ctrl Pts',(18.3130254811852,9.66566546403259,18.));
#37114=CARTESIAN_POINT('Ctrl Pts',(18.3630495772677,9.73189932619939,0.));
#37115=CARTESIAN_POINT('Ctrl Pts',(18.3630495772677,9.73189932619939,18.));
#37116=CARTESIAN_POINT('Ctrl Pts',(18.4125796444662,9.79873019947433,0.));
#37117=CARTESIAN_POINT('Ctrl Pts',(18.4125796444662,9.79873019947433,18.));
#37118=CARTESIAN_POINT('Ctrl Pts',(18.461614050347,9.86615372541684,0.));
#37119=CARTESIAN_POINT('Ctrl Pts',(18.461614050347,9.86615372541684,18.));
#37120=CARTESIAN_POINT('Ctrl Pts',(18.5101489409161,9.93416923996828,0.));
#37121=CARTESIAN_POINT('Ctrl Pts',(18.5101489409161,9.93416923996828,18.));
#37122=CARTESIAN_POINT('Ctrl Pts',(18.5581807679204,10.0027757313807,0.));
#37123=CARTESIAN_POINT('Ctrl Pts',(18.5581807679204,10.0027757313807,18.));
#37124=CARTESIAN_POINT('Ctrl Pts',(18.605709190442,10.0719672018851,0.));
#37125=CARTESIAN_POINT('Ctrl Pts',(18.605709190442,10.0719672018851,18.));
#37126=CARTESIAN_POINT('Ctrl Pts',(18.6527367592664,10.1417331637795,0.));
#37127=CARTESIAN_POINT('Ctrl Pts',(18.6527367592664,10.1417331637795,18.));
#37128=CARTESIAN_POINT('Ctrl Pts',(18.699267629819,10.2120606864872,0.));
#37129=CARTESIAN_POINT('Ctrl Pts',(18.699267629819,10.2120606864872,18.));
#37130=CARTESIAN_POINT('Ctrl Pts',(18.7453065790062,10.2829359603685,0.));
#37131=CARTESIAN_POINT('Ctrl Pts',(18.7453065790062,10.2829359603685,18.));
#37132=CARTESIAN_POINT('Ctrl Pts',(18.7908579693851,10.3543459451258,0.));
#37133=CARTESIAN_POINT('Ctrl Pts',(18.7908579693851,10.3543459451258,18.));
#37134=CARTESIAN_POINT('Ctrl Pts',(18.8359245594214,10.4262802670211,0.));
#37135=CARTESIAN_POINT('Ctrl Pts',(18.8359245594214,10.4262802670211,18.));
#37136=CARTESIAN_POINT('Ctrl Pts',(18.8805076729356,10.4987309368494,0.));
#37137=CARTESIAN_POINT('Ctrl Pts',(18.8805076729356,10.4987309368494,18.));
#37138=CARTESIAN_POINT('Ctrl Pts',(18.9246077453188,10.5716914651544,0.));
#37139=CARTESIAN_POINT('Ctrl Pts',(18.9246077453188,10.5716914651544,18.));
#37140=CARTESIAN_POINT('Ctrl Pts',(18.9682247574834,10.6451561585969,0.));
#37141=CARTESIAN_POINT('Ctrl Pts',(18.9682247574834,10.6451561585969,18.));
#37142=CARTESIAN_POINT('Ctrl Pts',(19.0113586878152,10.7191193896586,0.));
#37143=CARTESIAN_POINT('Ctrl Pts',(19.0113586878152,10.7191193896586,18.));
#37144=CARTESIAN_POINT('Ctrl Pts',(19.0540100416943,10.7935747414879,0.));
#37145=CARTESIAN_POINT('Ctrl Pts',(19.0540100416943,10.7935747414879,18.));
#37146=CARTESIAN_POINT('Ctrl Pts',(19.0961797996403,10.868515097783,0.));
#37147=CARTESIAN_POINT('Ctrl Pts',(19.0961797996403,10.868515097783,18.));
#37148=CARTESIAN_POINT('Ctrl Pts',(19.1378691901023,10.9439330179206,0.));
#37149=CARTESIAN_POINT('Ctrl Pts',(19.1378691901023,10.9439330179206,18.));
#37150=CARTESIAN_POINT('Ctrl Pts',(19.1790795192393,11.0198210228993,0.));
#37151=CARTESIAN_POINT('Ctrl Pts',(19.1790795192393,11.0198210228993,18.));
#37152=CARTESIAN_POINT('Ctrl Pts',(19.2198119937835,11.0961718903994,0.));
#37153=CARTESIAN_POINT('Ctrl Pts',(19.2198119937835,11.0961718903994,18.));
#37154=CARTESIAN_POINT('Ctrl Pts',(19.2600675167206,11.1729790050543,0.));
#37155=CARTESIAN_POINT('Ctrl Pts',(19.2600675167206,11.1729790050543,18.));
#37156=CARTESIAN_POINT('Ctrl Pts',(19.2998466936739,11.2502363198588,0.));
#37157=CARTESIAN_POINT('Ctrl Pts',(19.2998466936739,11.2502363198588,18.));
#37158=CARTESIAN_POINT('Ctrl Pts',(19.3391499248083,11.3279381634523,0.));
#37159=CARTESIAN_POINT('Ctrl Pts',(19.3391499248083,11.3279381634523,18.));
#37160=CARTESIAN_POINT('Ctrl Pts',(19.3779774742876,11.4060790880015,0.));
#37161=CARTESIAN_POINT('Ctrl Pts',(19.3779774742876,11.4060790880015,18.));
#37162=CARTESIAN_POINT('Ctrl Pts',(19.4163295466324,11.4846537135043,0.));
#37163=CARTESIAN_POINT('Ctrl Pts',(19.4163295466324,11.4846537135043,18.));
#37164=CARTESIAN_POINT('Ctrl Pts',(19.4542063779876,11.5636565297382,0.));
#37165=CARTESIAN_POINT('Ctrl Pts',(19.4542063779876,11.5636565297382,18.));
#37166=CARTESIAN_POINT('Ctrl Pts',(19.4916082541529,11.6430819099846,0.));
#37167=CARTESIAN_POINT('Ctrl Pts',(19.4916082541529,11.6430819099846,18.));
#37168=CARTESIAN_POINT('Ctrl Pts',(19.5285354853626,11.722924244195,0.));
#37169=CARTESIAN_POINT('Ctrl Pts',(19.5285354853626,11.722924244195,18.));
#37170=CARTESIAN_POINT('Ctrl Pts',(19.5649883985826,11.8031780389346,0.));
#37171=CARTESIAN_POINT('Ctrl Pts',(19.5649883985826,11.8031780389346,18.));
#37172=CARTESIAN_POINT('Ctrl Pts',(19.6009673241771,11.8838380136222,0.));
#37173=CARTESIAN_POINT('Ctrl Pts',(19.6009673241771,11.8838380136222,18.));
#37174=CARTESIAN_POINT('Ctrl Pts',(19.6364725931695,11.9648992312094,0.));
#37175=CARTESIAN_POINT('Ctrl Pts',(19.6364725931695,11.9648992312094,18.));
#37176=CARTESIAN_POINT('Ctrl Pts',(19.6715045149944,12.0463570680308,0.));
#37177=CARTESIAN_POINT('Ctrl Pts',(19.6715045149944,12.0463570680308,18.));
#37178=CARTESIAN_POINT('Ctrl Pts',(19.7060633406705,12.1282070378972,0.));
#37179=CARTESIAN_POINT('Ctrl Pts',(19.7060633406705,12.1282070378972,18.));
#37180=CARTESIAN_POINT('Ctrl Pts',(19.7401492304335,12.2104446447874,0.));
#37181=CARTESIAN_POINT('Ctrl Pts',(19.7401492304335,12.2104446447874,18.));
#37182=CARTESIAN_POINT('Ctrl Pts',(19.7737622285562,12.2930652417986,0.));
#37183=CARTESIAN_POINT('Ctrl Pts',(19.7737622285562,12.2930652417986,18.));
#37184=CARTESIAN_POINT('Ctrl Pts',(19.8069022248387,12.3760638341708,0.));
#37185=CARTESIAN_POINT('Ctrl Pts',(19.8069022248387,12.3760638341708,18.));
#37186=CARTESIAN_POINT('Ctrl Pts',(19.839568972011,12.4594350764989,0.));
#37187=CARTESIAN_POINT('Ctrl Pts',(19.839568972011,12.4594350764989,18.));
#37188=CARTESIAN_POINT('Ctrl Pts',(19.8717621942733,12.5431736030595,0.));
#37189=CARTESIAN_POINT('Ctrl Pts',(19.8717621942733,12.5431736030595,18.));
#37190=CARTESIAN_POINT('Ctrl Pts',(19.9034816813503,12.6272742843372,0.));
#37191=CARTESIAN_POINT('Ctrl Pts',(19.9034816813503,12.6272742843372,18.));
#37192=CARTESIAN_POINT('Ctrl Pts',(19.9347273847264,12.7117325003719,0.));
#37193=CARTESIAN_POINT('Ctrl Pts',(19.9347273847264,12.7117325003719,18.));
#37194=CARTESIAN_POINT('Ctrl Pts',(19.9654995335894,12.7965444294443,0.));
#37195=CARTESIAN_POINT('Ctrl Pts',(19.9654995335894,12.7965444294443,18.));
#37196=CARTESIAN_POINT('Ctrl Pts',(19.9957986945787,12.8817072534696,0.));
#37197=CARTESIAN_POINT('Ctrl Pts',(19.9957986945787,12.8817072534696,18.));
#37198=CARTESIAN_POINT('Ctrl Pts',(20.0256255826397,12.9672189949731,0.));
#37199=CARTESIAN_POINT('Ctrl Pts',(20.0256255826397,12.9672189949731,18.));
#37200=CARTESIAN_POINT('Ctrl Pts',(20.0491098457044,13.0359065249991,0.));
#37201=CARTESIAN_POINT('Ctrl Pts',(20.0491098457044,13.0359065249991,18.));
#37202=CARTESIAN_POINT('Ctrl Pts',(20.0665110891946,13.0875783330728,0.));
#37203=CARTESIAN_POINT('Ctrl Pts',(20.0665110891946,13.0875783330728,18.));
#37204=CARTESIAN_POINT('Ctrl Pts',(20.0780177478283,13.1220955868173,0.));
#37205=CARTESIAN_POINT('Ctrl Pts',(20.0780177478283,13.1220955868173,18.));
#37206=CARTESIAN_POINT('Ctrl Pts',(20.0837475345526,13.1393715591102,0.));
#37207=CARTESIAN_POINT('Ctrl Pts',(20.0837475345526,13.1393715591102,18.));
#37208=CARTESIAN_POINT('Ctrl Pts',(16.8707481591095,8.28171148831561,0.));
#37209=CARTESIAN_POINT('Ctrl Pts',(16.8848228151885,8.28862062120315,0.));
#37210=CARTESIAN_POINT('Ctrl Pts',(16.9126979078877,8.30290517019115,0.));
#37211=CARTESIAN_POINT('Ctrl Pts',(16.9536879065132,8.32573081382562,0.));
#37212=CARTESIAN_POINT('Ctrl Pts',(17.0067806259695,8.35882146841243,0.));
#37213=CARTESIAN_POINT('Ctrl Pts',(17.071033847921,8.40379607744266,0.));
#37214=CARTESIAN_POINT('Ctrl Pts',(17.1337886602855,8.45135198307876,0.));
#37215=CARTESIAN_POINT('Ctrl Pts',(17.1956428575086,8.50048099003882,0.));
#37216=CARTESIAN_POINT('Ctrl Pts',(17.2570167183611,8.55046295192433,0.));
#37217=CARTESIAN_POINT('Ctrl Pts',(17.3180459442745,8.60104338529165,0.));
#37218=CARTESIAN_POINT('Ctrl Pts',(17.3786861166843,8.65226368112816,0.));
#37219=CARTESIAN_POINT('Ctrl Pts',(17.438788019753,8.70433925112174,0.));
#37220=CARTESIAN_POINT('Ctrl Pts',(17.4981785296199,8.75752832625954,0.));
#37221=CARTESIAN_POINT('Ctrl Pts',(17.5567525798882,8.8119830723955,0.));
#37222=CARTESIAN_POINT('Ctrl Pts',(17.614513388992,8.86768402115343,0.));
#37223=CARTESIAN_POINT('Ctrl Pts',(17.6715250120654,8.92451585185175,0.));
#37224=CARTESIAN_POINT('Ctrl Pts',(17.7278841963319,8.98231202490685,0.));
#37225=CARTESIAN_POINT('Ctrl Pts',(17.7836872744016,9.04090748239097,0.));
#37226=CARTESIAN_POINT('Ctrl Pts',(17.8389924349283,9.10019864472208,0.));
#37227=CARTESIAN_POINT('Ctrl Pts',(17.8938116696237,9.16015616361609,0.));
#37228=CARTESIAN_POINT('Ctrl Pts',(17.9481305624284,9.22079331175917,0.));
#37229=CARTESIAN_POINT('Ctrl Pts',(18.0019206847747,9.2821461557447,0.));
#37230=CARTESIAN_POINT('Ctrl Pts',(18.0551538338035,9.34425079614396,0.));
#37231=CARTESIAN_POINT('Ctrl Pts',(18.1078184146735,9.40711718355464,0.));
#37232=CARTESIAN_POINT('Ctrl Pts',(18.1599204445014,9.47072748065831,0.));
#37233=CARTESIAN_POINT('Ctrl Pts',(18.2114756946126,9.53504856811685,0.));
#37234=CARTESIAN_POINT('Ctrl Pts',(18.2625044208165,9.60004042085347,0.));
#37235=CARTESIAN_POINT('Ctrl Pts',(18.3130254811852,9.66566546403259,0.));
#37236=CARTESIAN_POINT('Ctrl Pts',(18.3630495772677,9.73189932619939,0.));
#37237=CARTESIAN_POINT('Ctrl Pts',(18.4125796444662,9.79873019947433,0.));
#37238=CARTESIAN_POINT('Ctrl Pts',(18.461614050347,9.86615372541684,0.));
#37239=CARTESIAN_POINT('Ctrl Pts',(18.5101489409161,9.93416923996828,0.));
#37240=CARTESIAN_POINT('Ctrl Pts',(18.5581807679204,10.0027757313807,0.));
#37241=CARTESIAN_POINT('Ctrl Pts',(18.605709190442,10.0719672018851,0.));
#37242=CARTESIAN_POINT('Ctrl Pts',(18.6527367592664,10.1417331637795,0.));
#37243=CARTESIAN_POINT('Ctrl Pts',(18.699267629819,10.2120606864872,0.));
#37244=CARTESIAN_POINT('Ctrl Pts',(18.7453065790062,10.2829359603685,0.));
#37245=CARTESIAN_POINT('Ctrl Pts',(18.7908579693851,10.3543459451258,0.));
#37246=CARTESIAN_POINT('Ctrl Pts',(18.8359245594214,10.4262802670211,0.));
#37247=CARTESIAN_POINT('Ctrl Pts',(18.8805076729356,10.4987309368494,0.));
#37248=CARTESIAN_POINT('Ctrl Pts',(18.9246077453188,10.5716914651544,0.));
#37249=CARTESIAN_POINT('Ctrl Pts',(18.9682247574834,10.6451561585969,0.));
#37250=CARTESIAN_POINT('Ctrl Pts',(19.0113586878152,10.7191193896586,0.));
#37251=CARTESIAN_POINT('Ctrl Pts',(19.0540100416943,10.7935747414879,0.));
#37252=CARTESIAN_POINT('Ctrl Pts',(19.0961797996403,10.868515097783,0.));
#37253=CARTESIAN_POINT('Ctrl Pts',(19.1378691901023,10.9439330179206,0.));
#37254=CARTESIAN_POINT('Ctrl Pts',(19.1790795192393,11.0198210228993,0.));
#37255=CARTESIAN_POINT('Ctrl Pts',(19.2198119937835,11.0961718903994,0.));
#37256=CARTESIAN_POINT('Ctrl Pts',(19.2600675167206,11.1729790050543,0.));
#37257=CARTESIAN_POINT('Ctrl Pts',(19.2998466936739,11.2502363198588,0.));
#37258=CARTESIAN_POINT('Ctrl Pts',(19.3391499248083,11.3279381634523,0.));
#37259=CARTESIAN_POINT('Ctrl Pts',(19.3779774742876,11.4060790880015,0.));
#37260=CARTESIAN_POINT('Ctrl Pts',(19.4163295466324,11.4846537135043,0.));
#37261=CARTESIAN_POINT('Ctrl Pts',(19.4542063779876,11.5636565297382,0.));
#37262=CARTESIAN_POINT('Ctrl Pts',(19.4916082541529,11.6430819099846,0.));
#37263=CARTESIAN_POINT('Ctrl Pts',(19.5285354853626,11.722924244195,0.));
#37264=CARTESIAN_POINT('Ctrl Pts',(19.5649883985826,11.8031780389346,0.));
#37265=CARTESIAN_POINT('Ctrl Pts',(19.6009673241771,11.8838380136222,0.));
#37266=CARTESIAN_POINT('Ctrl Pts',(19.6364725931695,11.9648992312094,0.));
#37267=CARTESIAN_POINT('Ctrl Pts',(19.6715045149944,12.0463570680308,0.));
#37268=CARTESIAN_POINT('Ctrl Pts',(19.7060633406705,12.1282070378972,0.));
#37269=CARTESIAN_POINT('Ctrl Pts',(19.7401492304335,12.2104446447874,0.));
#37270=CARTESIAN_POINT('Ctrl Pts',(19.7737622285562,12.2930652417986,0.));
#37271=CARTESIAN_POINT('Ctrl Pts',(19.8069022248387,12.3760638341708,0.));
#37272=CARTESIAN_POINT('Ctrl Pts',(19.839568972011,12.4594350764989,0.));
#37273=CARTESIAN_POINT('Ctrl Pts',(19.8717621942733,12.5431736030595,0.));
#37274=CARTESIAN_POINT('Ctrl Pts',(19.9034816813503,12.6272742843372,0.));
#37275=CARTESIAN_POINT('Ctrl Pts',(19.9347273847264,12.7117325003719,0.));
#37276=CARTESIAN_POINT('Ctrl Pts',(19.9654995335894,12.7965444294443,0.));
#37277=CARTESIAN_POINT('Ctrl Pts',(20.0018585267766,12.8987398182747,0.));
#37278=CARTESIAN_POINT('Ctrl Pts',(20.0315673466055,12.9843387891477,0.));
#37279=CARTESIAN_POINT('Ctrl Pts',(20.054957345404,13.0530957702829,0.));
#37280=CARTESIAN_POINT('Ctrl Pts',(20.0722879610899,13.1048196144678,0.));
#37281=CARTESIAN_POINT('Ctrl Pts',(20.0837475345526,13.1393715591102,0.));
#37282=CARTESIAN_POINT('Ctrl Pts',(16.8707481591095,8.28171148831561,15.));
#37283=CARTESIAN_POINT('Ctrl Pts',(16.8848228151885,8.28862062120315,15.));
#37284=CARTESIAN_POINT('Ctrl Pts',(16.9126979078877,8.30290517019115,15.));
#37285=CARTESIAN_POINT('Ctrl Pts',(16.9536879065132,8.32573081382562,15.));
#37286=CARTESIAN_POINT('Ctrl Pts',(17.0067806259695,8.35882146841243,15.));
#37287=CARTESIAN_POINT('Ctrl Pts',(17.071033847921,8.40379607744266,15.));
#37288=CARTESIAN_POINT('Ctrl Pts',(17.1337886602855,8.45135198307876,15.));
#37289=CARTESIAN_POINT('Ctrl Pts',(17.1956428575086,8.50048099003882,15.));
#37290=CARTESIAN_POINT('Ctrl Pts',(17.2570167183611,8.55046295192433,15.));
#37291=CARTESIAN_POINT('Ctrl Pts',(17.3180459442745,8.60104338529165,15.));
#37292=CARTESIAN_POINT('Ctrl Pts',(17.3786861166843,8.65226368112816,15.));
#37293=CARTESIAN_POINT('Ctrl Pts',(17.438788019753,8.70433925112174,15.));
#37294=CARTESIAN_POINT('Ctrl Pts',(17.4981785296199,8.75752832625954,15.));
#37295=CARTESIAN_POINT('Ctrl Pts',(17.5567525798882,8.8119830723955,15.));
#37296=CARTESIAN_POINT('Ctrl Pts',(17.614513388992,8.86768402115343,15.));
#37297=CARTESIAN_POINT('Ctrl Pts',(17.6715250120654,8.92451585185175,15.));
#37298=CARTESIAN_POINT('Ctrl Pts',(17.7278841963319,8.98231202490685,15.));
#37299=CARTESIAN_POINT('Ctrl Pts',(17.7836872744016,9.04090748239097,15.));
#37300=CARTESIAN_POINT('Ctrl Pts',(17.8389924349283,9.10019864472208,15.));
#37301=CARTESIAN_POINT('Ctrl Pts',(17.8938116696237,9.16015616361609,15.));
#37302=CARTESIAN_POINT('Ctrl Pts',(17.9481305624284,9.22079331175917,15.));
#37303=CARTESIAN_POINT('Ctrl Pts',(18.0019206847747,9.2821461557447,15.));
#37304=CARTESIAN_POINT('Ctrl Pts',(18.0551538338035,9.34425079614396,15.));
#37305=CARTESIAN_POINT('Ctrl Pts',(18.1078184146735,9.40711718355464,15.));
#37306=CARTESIAN_POINT('Ctrl Pts',(18.1599204445014,9.47072748065831,15.));
#37307=CARTESIAN_POINT('Ctrl Pts',(18.2114756946126,9.53504856811685,15.));
#37308=CARTESIAN_POINT('Ctrl Pts',(18.2625044208165,9.60004042085347,15.));
#37309=CARTESIAN_POINT('Ctrl Pts',(18.3130254811852,9.66566546403259,15.));
#37310=CARTESIAN_POINT('Ctrl Pts',(18.3630495772677,9.73189932619939,15.));
#37311=CARTESIAN_POINT('Ctrl Pts',(18.4125796444662,9.79873019947433,15.));
#37312=CARTESIAN_POINT('Ctrl Pts',(18.461614050347,9.86615372541684,15.));
#37313=CARTESIAN_POINT('Ctrl Pts',(18.5101489409161,9.93416923996828,15.));
#37314=CARTESIAN_POINT('Ctrl Pts',(18.5581807679204,10.0027757313807,15.));
#37315=CARTESIAN_POINT('Ctrl Pts',(18.605709190442,10.0719672018851,15.));
#37316=CARTESIAN_POINT('Ctrl Pts',(18.6527367592664,10.1417331637795,15.));
#37317=CARTESIAN_POINT('Ctrl Pts',(18.699267629819,10.2120606864872,15.));
#37318=CARTESIAN_POINT('Ctrl Pts',(18.7453065790062,10.2829359603685,15.));
#37319=CARTESIAN_POINT('Ctrl Pts',(18.7908579693851,10.3543459451258,15.));
#37320=CARTESIAN_POINT('Ctrl Pts',(18.8359245594214,10.4262802670211,15.));
#37321=CARTESIAN_POINT('Ctrl Pts',(18.8805076729356,10.4987309368494,15.));
#37322=CARTESIAN_POINT('Ctrl Pts',(18.9246077453188,10.5716914651544,15.));
#37323=CARTESIAN_POINT('Ctrl Pts',(18.9682247574834,10.6451561585969,15.));
#37324=CARTESIAN_POINT('Ctrl Pts',(19.0113586878152,10.7191193896586,15.));
#37325=CARTESIAN_POINT('Ctrl Pts',(19.0540100416943,10.7935747414879,15.));
#37326=CARTESIAN_POINT('Ctrl Pts',(19.0961797996403,10.868515097783,15.));
#37327=CARTESIAN_POINT('Ctrl Pts',(19.1378691901023,10.9439330179206,15.));
#37328=CARTESIAN_POINT('Ctrl Pts',(19.1790795192393,11.0198210228993,15.));
#37329=CARTESIAN_POINT('Ctrl Pts',(19.2198119937835,11.0961718903994,15.));
#37330=CARTESIAN_POINT('Ctrl Pts',(19.2600675167206,11.1729790050543,15.));
#37331=CARTESIAN_POINT('Ctrl Pts',(19.2998466936739,11.2502363198588,15.));
#37332=CARTESIAN_POINT('Ctrl Pts',(19.3391499248083,11.3279381634523,15.));
#37333=CARTESIAN_POINT('Ctrl Pts',(19.3779774742876,11.4060790880015,15.));
#37334=CARTESIAN_POINT('Ctrl Pts',(19.4163295466324,11.4846537135043,15.));
#37335=CARTESIAN_POINT('Ctrl Pts',(19.4542063779876,11.5636565297382,15.));
#37336=CARTESIAN_POINT('Ctrl Pts',(19.4916082541529,11.6430819099846,15.));
#37337=CARTESIAN_POINT('Ctrl Pts',(19.5285354853626,11.722924244195,15.));
#37338=CARTESIAN_POINT('Ctrl Pts',(19.5649883985826,11.8031780389346,15.));
#37339=CARTESIAN_POINT('Ctrl Pts',(19.6009673241771,11.8838380136222,15.));
#37340=CARTESIAN_POINT('Ctrl Pts',(19.6364725931695,11.9648992312094,15.));
#37341=CARTESIAN_POINT('Ctrl Pts',(19.6715045149944,12.0463570680308,15.));
#37342=CARTESIAN_POINT('Ctrl Pts',(19.7060633406705,12.1282070378972,15.));
#37343=CARTESIAN_POINT('Ctrl Pts',(19.7401492304335,12.2104446447874,15.));
#37344=CARTESIAN_POINT('Ctrl Pts',(19.7737622285562,12.2930652417986,15.));
#37345=CARTESIAN_POINT('Ctrl Pts',(19.8069022248387,12.3760638341708,15.));
#37346=CARTESIAN_POINT('Ctrl Pts',(19.839568972011,12.4594350764989,15.));
#37347=CARTESIAN_POINT('Ctrl Pts',(19.8717621942733,12.5431736030595,15.));
#37348=CARTESIAN_POINT('Ctrl Pts',(19.9034816813503,12.6272742843372,15.));
#37349=CARTESIAN_POINT('Ctrl Pts',(19.9347273847264,12.7117325003719,15.));
#37350=CARTESIAN_POINT('Ctrl Pts',(19.9654995335894,12.7965444294443,15.));
#37351=CARTESIAN_POINT('Ctrl Pts',(20.0018585267766,12.8987398182747,15.));
#37352=CARTESIAN_POINT('Ctrl Pts',(20.0315673466055,12.9843387891477,15.));
#37353=CARTESIAN_POINT('Ctrl Pts',(20.054957345404,13.0530957702829,15.));
#37354=CARTESIAN_POINT('Ctrl Pts',(20.0722879610899,13.1048196144678,15.));
#37355=CARTESIAN_POINT('Ctrl Pts',(20.0837475345526,13.1393715591102,15.));
#37356=CARTESIAN_POINT('Origin',(0.,0.,0.));
#37357=CARTESIAN_POINT('Origin',(0.,0.,0.));
#37358=CARTESIAN_POINT('Origin',(0.,0.,0.));
#37359=CARTESIAN_POINT('Origin',(0.,0.,0.));
#37360=CARTESIAN_POINT('Origin',(0.,0.,0.));
#37361=CARTESIAN_POINT('Origin',(0.,0.,0.));
#37362=CARTESIAN_POINT('Origin',(0.,0.,0.));
#37363=CARTESIAN_POINT('Origin',(0.,0.,0.));
#37364=CARTESIAN_POINT('',(14.9562571344462,3.5508810918317,0.));
#37365=CARTESIAN_POINT('Origin',(0.,0.,0.));
#37366=CARTESIAN_POINT('',(16.1003491021971,2.79663061332403,0.));
#37367=CARTESIAN_POINT('Origin',(15.9292116709051,3.78187778008512,0.));
#37368=CARTESIAN_POINT('',(18.5165898451125,3.2163316265074,0.));
#37369=CARTESIAN_POINT('',(15.135366975784,2.62901321950806,0.));
#37370=CARTESIAN_POINT('',(23.9712218930251,1.17495572484827,0.));
#37371=CARTESIAN_POINT('Ctrl Pts',(18.5165898451125,3.2163316265074,0.));
#37372=CARTESIAN_POINT('Ctrl Pts',(18.5320375674878,3.2190148958593,0.));
#37373=CARTESIAN_POINT('Ctrl Pts',(18.5629852384321,3.22384302136592,0.));
#37374=CARTESIAN_POINT('Ctrl Pts',(18.6095634206219,3.2294700044416,0.));
#37375=CARTESIAN_POINT('Ctrl Pts',(18.6719665316945,3.23390622002644,0.));
#37376=CARTESIAN_POINT('Ctrl Pts',(18.7503838921122,3.23528809328097,0.));
#37377=CARTESIAN_POINT('Ctrl Pts',(18.8291062617862,3.23370091065669,0.));
#37378=CARTESIAN_POINT('Ctrl Pts',(18.908024664264,3.23031169402939,0.));
#37379=CARTESIAN_POINT('Ctrl Pts',(18.987055820781,3.22595008773715,0.));
#37380=CARTESIAN_POINT('Ctrl Pts',(19.0661599344864,3.22090173651085,0.));
#37381=CARTESIAN_POINT('Ctrl Pts',(19.1453253990185,3.21510704576117,0.));
#37382=CARTESIAN_POINT('Ctrl Pts',(19.2245581120423,3.2083040369031,0.));
#37383=CARTESIAN_POINT('Ctrl Pts',(19.3038697977783,3.2001820370274,0.));
#37384=CARTESIAN_POINT('Ctrl Pts',(19.3832648965708,3.19055618489382,0.));
#37385=CARTESIAN_POINT('Ctrl Pts',(19.4627345689632,3.17944412249754,0.));
#37386=CARTESIAN_POINT('Ctrl Pts',(19.5422628528517,3.16697679689294,0.));
#37387=CARTESIAN_POINT('Ctrl Pts',(19.6218301288731,3.15334580802458,0.));
#37388=CARTESIAN_POINT('Ctrl Pts',(19.7014173131304,3.13874131344865,0.));
#37389=CARTESIAN_POINT('Ctrl Pts',(19.7810105986827,3.1232813132398,0.));
#37390=CARTESIAN_POINT('Ctrl Pts',(19.8606024365399,3.10699659920993,0.));
#37391=CARTESIAN_POINT('Ctrl Pts',(19.9401889653541,3.08986795998319,0.));
#37392=CARTESIAN_POINT('Ctrl Pts',(20.0197683853426,3.07184950717982,0.));
#37393=CARTESIAN_POINT('Ctrl Pts',(20.0993390992966,3.05289545759951,0.));
#37394=CARTESIAN_POINT('Ctrl Pts',(20.178897575607,3.03299094576288,0.));
#37395=CARTESIAN_POINT('Ctrl Pts',(20.2584381977107,3.01215393913612,0.));
#37396=CARTESIAN_POINT('Ctrl Pts',(20.3379542578194,2.99042050197904,0.));
#37397=CARTESIAN_POINT('Ctrl Pts',(20.4174386170774,2.96783492132513,0.));
#37398=CARTESIAN_POINT('Ctrl Pts',(20.4968844460513,2.94443868035154,0.));
#37399=CARTESIAN_POINT('Ctrl Pts',(20.5762860772943,2.92025778619206,0.));
#37400=CARTESIAN_POINT('Ctrl Pts',(20.6556389450993,2.89530351700805,0.));
#37401=CARTESIAN_POINT('Ctrl Pts',(20.7349391669725,2.86957843933153,0.));
#37402=CARTESIAN_POINT('Ctrl Pts',(20.8141832346435,2.84308082507644,0.));
#37403=CARTESIAN_POINT('Ctrl Pts',(20.8933676828246,2.81580940715318,0.));
#37404=CARTESIAN_POINT('Ctrl Pts',(20.9724887103073,2.78776883747222,0.));
#37405=CARTESIAN_POINT('Ctrl Pts',(21.0515422162039,2.7589691000769,0.));
#37406=CARTESIAN_POINT('Ctrl Pts',(21.1305239619219,2.72942309852119,0.));
#37407=CARTESIAN_POINT('Ctrl Pts',(21.2094296949571,2.69914481283353,0.));
#37408=CARTESIAN_POINT('Ctrl Pts',(21.2882552797978,2.668147357083,0.));
#37409=CARTESIAN_POINT('Ctrl Pts',(21.3669968505594,2.6364407451853,0.));
#37410=CARTESIAN_POINT('Ctrl Pts',(21.4456507822983,2.60403221866523,0.));
#37411=CARTESIAN_POINT('Ctrl Pts',(21.5242136128466,2.5709272835198,0.));
#37412=CARTESIAN_POINT('Ctrl Pts',(21.6026819803014,2.53713053453766,0.));
#37413=CARTESIAN_POINT('Ctrl Pts',(21.6810525594039,2.50264651177235,0.));
#37414=CARTESIAN_POINT('Ctrl Pts',(21.7593219872847,2.46748070362075,0.));
#37415=CARTESIAN_POINT('Ctrl Pts',(21.8374868743435,2.43163944362692,0.));
#37416=CARTESIAN_POINT('Ctrl Pts',(21.9155438409279,2.39512947344577,0.));
#37417=CARTESIAN_POINT('Ctrl Pts',(21.9934895476958,2.35795761145761,0.));
#37418=CARTESIAN_POINT('Ctrl Pts',(22.0713207257413,2.32013040994125,0.));
#37419=CARTESIAN_POINT('Ctrl Pts',(22.1490342171802,2.28165375160231,0.));
#37420=CARTESIAN_POINT('Ctrl Pts',(22.2266269576315,2.24253288454712,0.));
#37421=CARTESIAN_POINT('Ctrl Pts',(22.3040959372933,2.20277263221399,0.));
#37422=CARTESIAN_POINT('Ctrl Pts',(22.3814381677224,2.16237755726404,0.));
#37423=CARTESIAN_POINT('Ctrl Pts',(22.4586506520939,2.1213521324248,0.));
#37424=CARTESIAN_POINT('Ctrl Pts',(22.5357303426251,2.07970095436224,0.));
#37425=CARTESIAN_POINT('Ctrl Pts',(22.6126741632309,2.03742874317627,0.));
#37426=CARTESIAN_POINT('Ctrl Pts',(22.6894790673923,1.99454021984253,0.));
#37427=CARTESIAN_POINT('Ctrl Pts',(22.7661420906702,1.95104002082891,0.));
#37428=CARTESIAN_POINT('Ctrl Pts',(22.8426603964871,1.90693261239855,0.));
#37429=CARTESIAN_POINT('Ctrl Pts',(22.9190313507225,1.86222218327819,0.));
#37430=CARTESIAN_POINT('Ctrl Pts',(22.9952524859917,1.81691265597281,0.));
#37431=CARTESIAN_POINT('Ctrl Pts',(23.0713213684573,1.77100780743078,0.));
#37432=CARTESIAN_POINT('Ctrl Pts',(23.1472354850579,1.72451136919382,0.));
#37433=CARTESIAN_POINT('Ctrl Pts',(23.2229921402299,1.67742712670823,0.));
#37434=CARTESIAN_POINT('Ctrl Pts',(23.2985883089733,1.62975905604583,0.));
#37435=CARTESIAN_POINT('Ctrl Pts',(23.3740206492924,1.58151133638847,0.));
#37436=CARTESIAN_POINT('Ctrl Pts',(23.4492857841673,1.53268814658653,0.));
#37437=CARTESIAN_POINT('Ctrl Pts',(23.5243805284282,1.48329351290851,0.));
#37438=CARTESIAN_POINT('Ctrl Pts',(23.5993021272808,1.4333311444639,0.));
#37439=CARTESIAN_POINT('Ctrl Pts',(23.6740485197917,1.38280426780156,0.));
#37440=CARTESIAN_POINT('Ctrl Pts',(23.7635325055853,1.32149774147467,0.));
#37441=CARTESIAN_POINT('Ctrl Pts',(23.8378812584003,1.2697091254959,0.));
#37442=CARTESIAN_POINT('Ctrl Pts',(23.89721850443,1.22783185562043,0.));
#37443=CARTESIAN_POINT('Ctrl Pts',(23.9416417798466,1.19617306697386,0.));
#37444=CARTESIAN_POINT('Ctrl Pts',(23.9712218930251,1.17495572484832,0.));
#37445=CARTESIAN_POINT('',(23.9712218930251,-1.17495572484832,0.));
#37446=CARTESIAN_POINT('Origin',(1.15463194561016E-13,-6.93889390390723E-17,
0.));
#37447=CARTESIAN_POINT('',(18.5165898451125,-3.2163316265074,0.));
#37448=CARTESIAN_POINT('Ctrl Pts',(18.5165898451125,-3.2163316265074,0.));
#37449=CARTESIAN_POINT('Ctrl Pts',(18.5320375674878,-3.2190148958593,0.));
#37450=CARTESIAN_POINT('Ctrl Pts',(18.5629852384321,-3.22384302136592,0.));
#37451=CARTESIAN_POINT('Ctrl Pts',(18.6095634206219,-3.2294700044416,0.));
#37452=CARTESIAN_POINT('Ctrl Pts',(18.6719665316945,-3.23390622002644,0.));
#37453=CARTESIAN_POINT('Ctrl Pts',(18.7503838921122,-3.23528809328097,0.));
#37454=CARTESIAN_POINT('Ctrl Pts',(18.8291062617862,-3.23370091065669,0.));
#37455=CARTESIAN_POINT('Ctrl Pts',(18.908024664264,-3.23031169402939,0.));
#37456=CARTESIAN_POINT('Ctrl Pts',(18.987055820781,-3.22595008773715,0.));
#37457=CARTESIAN_POINT('Ctrl Pts',(19.0661599344864,-3.22090173651085,0.));
#37458=CARTESIAN_POINT('Ctrl Pts',(19.1453253990185,-3.21510704576117,0.));
#37459=CARTESIAN_POINT('Ctrl Pts',(19.2245581120423,-3.2083040369031,0.));
#37460=CARTESIAN_POINT('Ctrl Pts',(19.3038697977783,-3.2001820370274,0.));
#37461=CARTESIAN_POINT('Ctrl Pts',(19.3832648965708,-3.19055618489382,0.));
#37462=CARTESIAN_POINT('Ctrl Pts',(19.4627345689632,-3.17944412249754,0.));
#37463=CARTESIAN_POINT('Ctrl Pts',(19.5422628528517,-3.16697679689294,0.));
#37464=CARTESIAN_POINT('Ctrl Pts',(19.6218301288731,-3.15334580802458,0.));
#37465=CARTESIAN_POINT('Ctrl Pts',(19.7014173131304,-3.13874131344865,0.));
#37466=CARTESIAN_POINT('Ctrl Pts',(19.7810105986827,-3.1232813132398,0.));
#37467=CARTESIAN_POINT('Ctrl Pts',(19.8606024365399,-3.10699659920993,0.));
#37468=CARTESIAN_POINT('Ctrl Pts',(19.9401889653541,-3.08986795998319,0.));
#37469=CARTESIAN_POINT('Ctrl Pts',(20.0197683853426,-3.07184950717982,0.));
#37470=CARTESIAN_POINT('Ctrl Pts',(20.0993390992966,-3.05289545759951,0.));
#37471=CARTESIAN_POINT('Ctrl Pts',(20.178897575607,-3.03299094576288,0.));
#37472=CARTESIAN_POINT('Ctrl Pts',(20.2584381977107,-3.01215393913612,0.));
#37473=CARTESIAN_POINT('Ctrl Pts',(20.3379542578194,-2.99042050197904,0.));
#37474=CARTESIAN_POINT('Ctrl Pts',(20.4174386170774,-2.96783492132513,0.));
#37475=CARTESIAN_POINT('Ctrl Pts',(20.4968844460513,-2.94443868035154,0.));
#37476=CARTESIAN_POINT('Ctrl Pts',(20.5762860772943,-2.92025778619206,0.));
#37477=CARTESIAN_POINT('Ctrl Pts',(20.6556389450993,-2.89530351700805,0.));
#37478=CARTESIAN_POINT('Ctrl Pts',(20.7349391669725,-2.86957843933153,0.));
#37479=CARTESIAN_POINT('Ctrl Pts',(20.8141832346435,-2.84308082507644,0.));
#37480=CARTESIAN_POINT('Ctrl Pts',(20.8933676828246,-2.81580940715318,0.));
#37481=CARTESIAN_POINT('Ctrl Pts',(20.9724887103073,-2.78776883747222,0.));
#37482=CARTESIAN_POINT('Ctrl Pts',(21.0515422162039,-2.7589691000769,0.));
#37483=CARTESIAN_POINT('Ctrl Pts',(21.1305239619219,-2.72942309852119,0.));
#37484=CARTESIAN_POINT('Ctrl Pts',(21.2094296949571,-2.69914481283353,0.));
#37485=CARTESIAN_POINT('Ctrl Pts',(21.2882552797978,-2.668147357083,0.));
#37486=CARTESIAN_POINT('Ctrl Pts',(21.3669968505594,-2.6364407451853,0.));
#37487=CARTESIAN_POINT('Ctrl Pts',(21.4456507822983,-2.60403221866523,0.));
#37488=CARTESIAN_POINT('Ctrl Pts',(21.5242136128466,-2.5709272835198,0.));
#37489=CARTESIAN_POINT('Ctrl Pts',(21.6026819803014,-2.53713053453766,0.));
#37490=CARTESIAN_POINT('Ctrl Pts',(21.6810525594039,-2.50264651177235,0.));
#37491=CARTESIAN_POINT('Ctrl Pts',(21.7593219872847,-2.46748070362075,0.));
#37492=CARTESIAN_POINT('Ctrl Pts',(21.8374868743435,-2.43163944362692,0.));
#37493=CARTESIAN_POINT('Ctrl Pts',(21.9155438409279,-2.39512947344577,0.));
#37494=CARTESIAN_POINT('Ctrl Pts',(21.9934895476958,-2.35795761145761,0.));
#37495=CARTESIAN_POINT('Ctrl Pts',(22.0713207257413,-2.32013040994125,0.));
#37496=CARTESIAN_POINT('Ctrl Pts',(22.1490342171802,-2.28165375160231,0.));
#37497=CARTESIAN_POINT('Ctrl Pts',(22.2266269576315,-2.24253288454712,0.));
#37498=CARTESIAN_POINT('Ctrl Pts',(22.3040959372933,-2.20277263221399,0.));
#37499=CARTESIAN_POINT('Ctrl Pts',(22.3814381677224,-2.16237755726404,0.));
#37500=CARTESIAN_POINT('Ctrl Pts',(22.4586506520939,-2.1213521324248,0.));
#37501=CARTESIAN_POINT('Ctrl Pts',(22.5357303426251,-2.07970095436224,0.));
#37502=CARTESIAN_POINT('Ctrl Pts',(22.6126741632309,-2.03742874317627,0.));
#37503=CARTESIAN_POINT('Ctrl Pts',(22.6894790673923,-1.99454021984253,0.));
#37504=CARTESIAN_POINT('Ctrl Pts',(22.7661420906702,-1.95104002082891,0.));
#37505=CARTESIAN_POINT('Ctrl Pts',(22.8426603964871,-1.90693261239855,0.));
#37506=CARTESIAN_POINT('Ctrl Pts',(22.9190313507225,-1.86222218327819,0.));
#37507=CARTESIAN_POINT('Ctrl Pts',(22.9952524859917,-1.81691265597281,0.));
#37508=CARTESIAN_POINT('Ctrl Pts',(23.0713213684573,-1.77100780743078,0.));
#37509=CARTESIAN_POINT('Ctrl Pts',(23.1472354850579,-1.72451136919382,0.));
#37510=CARTESIAN_POINT('Ctrl Pts',(23.2229921402299,-1.67742712670823,0.));
#37511=CARTESIAN_POINT('Ctrl Pts',(23.2985883089733,-1.62975905604583,0.));
#37512=CARTESIAN_POINT('Ctrl Pts',(23.3740206492924,-1.58151133638847,0.));
#37513=CARTESIAN_POINT('Ctrl Pts',(23.4492857841673,-1.53268814658653,0.));
#37514=CARTESIAN_POINT('Ctrl Pts',(23.5243805284282,-1.48329351290851,0.));
#37515=CARTESIAN_POINT('Ctrl Pts',(23.5993021272808,-1.4333311444639,0.));
#37516=CARTESIAN_POINT('Ctrl Pts',(23.6740485197917,-1.38280426780156,0.));
#37517=CARTESIAN_POINT('Ctrl Pts',(23.7635325055853,-1.32149774147467,0.));
#37518=CARTESIAN_POINT('Ctrl Pts',(23.8378812584003,-1.2697091254959,0.));
#37519=CARTESIAN_POINT('Ctrl Pts',(23.89721850443,-1.22783185562043,0.));
#37520=CARTESIAN_POINT('Ctrl Pts',(23.9416417798466,-1.19617306697386,0.));
#37521=CARTESIAN_POINT('Ctrl Pts',(23.9712218930251,-1.17495572484832,0.));
#37522=CARTESIAN_POINT('',(16.1003491021971,-2.79663061332403,0.));
#37523=CARTESIAN_POINT('',(15.135366975784,-2.62901321950806,0.));
#37524=CARTESIAN_POINT('',(14.9562571344462,-3.5508810918317,0.));
#37525=CARTESIAN_POINT('Origin',(15.9292116709051,-3.78187778008512,0.));
#37526=CARTESIAN_POINT('Origin',(0.,0.,0.));
#37527=CARTESIAN_POINT('Origin',(0.,0.,0.));
#37528=CARTESIAN_POINT('Origin',(0.,0.,15.));
#37529=CARTESIAN_POINT('',(14.9562571344462,-3.5508810918317,15.));
#37530=CARTESIAN_POINT('Origin',(0.,0.,15.));
#37531=CARTESIAN_POINT('',(16.1003491021971,-2.79663061332403,15.));
#37532=CARTESIAN_POINT('Origin',(15.9292116709051,-3.78187778008512,15.));
#37533=CARTESIAN_POINT('',(18.5165898451125,-3.2163316265074,15.));
#37534=CARTESIAN_POINT('',(15.135366975784,-2.62901321950806,15.));
#37535=CARTESIAN_POINT('',(23.9712218930251,-1.17495572484832,15.));
#37536=CARTESIAN_POINT('Ctrl Pts',(18.5165898451125,-3.2163316265074,15.));
#37537=CARTESIAN_POINT('Ctrl Pts',(18.5320375674878,-3.2190148958593,15.));
#37538=CARTESIAN_POINT('Ctrl Pts',(18.5629852384321,-3.22384302136592,15.));
#37539=CARTESIAN_POINT('Ctrl Pts',(18.6095634206219,-3.2294700044416,15.));
#37540=CARTESIAN_POINT('Ctrl Pts',(18.6719665316945,-3.23390622002644,15.));
#37541=CARTESIAN_POINT('Ctrl Pts',(18.7503838921122,-3.23528809328097,15.));
#37542=CARTESIAN_POINT('Ctrl Pts',(18.8291062617862,-3.23370091065669,15.));
#37543=CARTESIAN_POINT('Ctrl Pts',(18.908024664264,-3.23031169402939,15.));
#37544=CARTESIAN_POINT('Ctrl Pts',(18.987055820781,-3.22595008773715,15.));
#37545=CARTESIAN_POINT('Ctrl Pts',(19.0661599344864,-3.22090173651085,15.));
#37546=CARTESIAN_POINT('Ctrl Pts',(19.1453253990185,-3.21510704576117,15.));
#37547=CARTESIAN_POINT('Ctrl Pts',(19.2245581120423,-3.2083040369031,15.));
#37548=CARTESIAN_POINT('Ctrl Pts',(19.3038697977783,-3.2001820370274,15.));
#37549=CARTESIAN_POINT('Ctrl Pts',(19.3832648965708,-3.19055618489382,15.));
#37550=CARTESIAN_POINT('Ctrl Pts',(19.4627345689632,-3.17944412249754,15.));
#37551=CARTESIAN_POINT('Ctrl Pts',(19.5422628528517,-3.16697679689294,15.));
#37552=CARTESIAN_POINT('Ctrl Pts',(19.6218301288731,-3.15334580802458,15.));
#37553=CARTESIAN_POINT('Ctrl Pts',(19.7014173131304,-3.13874131344865,15.));
#37554=CARTESIAN_POINT('Ctrl Pts',(19.7810105986827,-3.1232813132398,15.));
#37555=CARTESIAN_POINT('Ctrl Pts',(19.8606024365399,-3.10699659920993,15.));
#37556=CARTESIAN_POINT('Ctrl Pts',(19.9401889653541,-3.08986795998319,15.));
#37557=CARTESIAN_POINT('Ctrl Pts',(20.0197683853426,-3.07184950717982,15.));
#37558=CARTESIAN_POINT('Ctrl Pts',(20.0993390992966,-3.05289545759951,15.));
#37559=CARTESIAN_POINT('Ctrl Pts',(20.178897575607,-3.03299094576288,15.));
#37560=CARTESIAN_POINT('Ctrl Pts',(20.2584381977107,-3.01215393913612,15.));
#37561=CARTESIAN_POINT('Ctrl Pts',(20.3379542578194,-2.99042050197904,15.));
#37562=CARTESIAN_POINT('Ctrl Pts',(20.4174386170774,-2.96783492132513,15.));
#37563=CARTESIAN_POINT('Ctrl Pts',(20.4968844460513,-2.94443868035154,15.));
#37564=CARTESIAN_POINT('Ctrl Pts',(20.5762860772943,-2.92025778619206,15.));
#37565=CARTESIAN_POINT('Ctrl Pts',(20.6556389450993,-2.89530351700805,15.));
#37566=CARTESIAN_POINT('Ctrl Pts',(20.7349391669725,-2.86957843933153,15.));
#37567=CARTESIAN_POINT('Ctrl Pts',(20.8141832346435,-2.84308082507644,15.));
#37568=CARTESIAN_POINT('Ctrl Pts',(20.8933676828246,-2.81580940715318,15.));
#37569=CARTESIAN_POINT('Ctrl Pts',(20.9724887103073,-2.78776883747222,15.));
#37570=CARTESIAN_POINT('Ctrl Pts',(21.0515422162039,-2.7589691000769,15.));
#37571=CARTESIAN_POINT('Ctrl Pts',(21.1305239619219,-2.72942309852119,15.));
#37572=CARTESIAN_POINT('Ctrl Pts',(21.2094296949571,-2.69914481283353,15.));
#37573=CARTESIAN_POINT('Ctrl Pts',(21.2882552797978,-2.668147357083,15.));
#37574=CARTESIAN_POINT('Ctrl Pts',(21.3669968505594,-2.6364407451853,15.));
#37575=CARTESIAN_POINT('Ctrl Pts',(21.4456507822983,-2.60403221866523,15.));
#37576=CARTESIAN_POINT('Ctrl Pts',(21.5242136128466,-2.5709272835198,15.));
#37577=CARTESIAN_POINT('Ctrl Pts',(21.6026819803014,-2.53713053453766,15.));
#37578=CARTESIAN_POINT('Ctrl Pts',(21.6810525594039,-2.50264651177235,15.));
#37579=CARTESIAN_POINT('Ctrl Pts',(21.7593219872847,-2.46748070362075,15.));
#37580=CARTESIAN_POINT('Ctrl Pts',(21.8374868743435,-2.43163944362692,15.));
#37581=CARTESIAN_POINT('Ctrl Pts',(21.9155438409279,-2.39512947344577,15.));
#37582=CARTESIAN_POINT('Ctrl Pts',(21.9934895476958,-2.35795761145761,15.));
#37583=CARTESIAN_POINT('Ctrl Pts',(22.0713207257413,-2.32013040994125,15.));
#37584=CARTESIAN_POINT('Ctrl Pts',(22.1490342171802,-2.28165375160231,15.));
#37585=CARTESIAN_POINT('Ctrl Pts',(22.2266269576315,-2.24253288454712,15.));
#37586=CARTESIAN_POINT('Ctrl Pts',(22.3040959372933,-2.20277263221399,15.));
#37587=CARTESIAN_POINT('Ctrl Pts',(22.3814381677224,-2.16237755726404,15.));
#37588=CARTESIAN_POINT('Ctrl Pts',(22.4586506520939,-2.1213521324248,15.));
#37589=CARTESIAN_POINT('Ctrl Pts',(22.5357303426251,-2.07970095436224,15.));
#37590=CARTESIAN_POINT('Ctrl Pts',(22.6126741632309,-2.03742874317627,15.));
#37591=CARTESIAN_POINT('Ctrl Pts',(22.6894790673923,-1.99454021984253,15.));
#37592=CARTESIAN_POINT('Ctrl Pts',(22.7661420906702,-1.95104002082891,15.));
#37593=CARTESIAN_POINT('Ctrl Pts',(22.8426603964871,-1.90693261239855,15.));
#37594=CARTESIAN_POINT('Ctrl Pts',(22.9190313507225,-1.86222218327819,15.));
#37595=CARTESIAN_POINT('Ctrl Pts',(22.9952524859917,-1.81691265597281,15.));
#37596=CARTESIAN_POINT('Ctrl Pts',(23.0713213684573,-1.77100780743078,15.));
#37597=CARTESIAN_POINT('Ctrl Pts',(23.1472354850579,-1.72451136919382,15.));
#37598=CARTESIAN_POINT('Ctrl Pts',(23.2229921402299,-1.67742712670823,15.));
#37599=CARTESIAN_POINT('Ctrl Pts',(23.2985883089733,-1.62975905604583,15.));
#37600=CARTESIAN_POINT('Ctrl Pts',(23.3740206492924,-1.58151133638847,15.));
#37601=CARTESIAN_POINT('Ctrl Pts',(23.4492857841673,-1.53268814658653,15.));
#37602=CARTESIAN_POINT('Ctrl Pts',(23.5243805284282,-1.48329351290851,15.));
#37603=CARTESIAN_POINT('Ctrl Pts',(23.5993021272808,-1.4333311444639,15.));
#37604=CARTESIAN_POINT('Ctrl Pts',(23.6740485197917,-1.38280426780156,15.));
#37605=CARTESIAN_POINT('Ctrl Pts',(23.7635325055853,-1.32149774147467,15.));
#37606=CARTESIAN_POINT('Ctrl Pts',(23.8378812584003,-1.2697091254959,15.));
#37607=CARTESIAN_POINT('Ctrl Pts',(23.89721850443,-1.22783185562043,15.));
#37608=CARTESIAN_POINT('Ctrl Pts',(23.9416417798466,-1.19617306697386,15.));
#37609=CARTESIAN_POINT('Ctrl Pts',(23.9712218930251,-1.17495572484832,15.));
#37610=CARTESIAN_POINT('',(23.9712218930251,1.17495572484827,15.));
#37611=CARTESIAN_POINT('Origin',(1.15463194561016E-13,-6.93889390390723E-17,
15.));
#37612=CARTESIAN_POINT('',(18.5165898451125,3.2163316265074,15.));
#37613=CARTESIAN_POINT('Ctrl Pts',(23.9712218930251,1.17495572484832,15.));
#37614=CARTESIAN_POINT('Ctrl Pts',(23.9564318364582,1.18556439589232,15.));
#37615=CARTESIAN_POINT('Ctrl Pts',(23.9268340213744,1.20672599652272,15.));
#37616=CARTESIAN_POINT('Ctrl Pts',(23.8823841929226,1.2383011730893,15.));
#37617=CARTESIAN_POINT('Ctrl Pts',(23.8230115078373,1.28006684869166,15.));
#37618=CARTESIAN_POINT('Ctrl Pts',(23.748618507953,1.33171549586249,15.));
#37619=CARTESIAN_POINT('Ctrl Pts',(23.6740485197917,1.38280426780156,15.));
#37620=CARTESIAN_POINT('Ctrl Pts',(23.5993021272808,1.4333311444639,15.));
#37621=CARTESIAN_POINT('Ctrl Pts',(23.5243805284282,1.48329351290851,15.));
#37622=CARTESIAN_POINT('Ctrl Pts',(23.4492857841673,1.53268814658653,15.));
#37623=CARTESIAN_POINT('Ctrl Pts',(23.3740206492924,1.58151133638847,15.));
#37624=CARTESIAN_POINT('Ctrl Pts',(23.2985883089733,1.62975905604583,15.));
#37625=CARTESIAN_POINT('Ctrl Pts',(23.2229921402299,1.67742712670823,15.));
#37626=CARTESIAN_POINT('Ctrl Pts',(23.1472354850579,1.72451136919382,15.));
#37627=CARTESIAN_POINT('Ctrl Pts',(23.0713213684573,1.77100780743078,15.));
#37628=CARTESIAN_POINT('Ctrl Pts',(22.9952524859917,1.81691265597281,15.));
#37629=CARTESIAN_POINT('Ctrl Pts',(22.9190313507225,1.86222218327819,15.));
#37630=CARTESIAN_POINT('Ctrl Pts',(22.8426603964871,1.90693261239855,15.));
#37631=CARTESIAN_POINT('Ctrl Pts',(22.7661420906702,1.95104002082891,15.));
#37632=CARTESIAN_POINT('Ctrl Pts',(22.6894790673923,1.99454021984253,15.));
#37633=CARTESIAN_POINT('Ctrl Pts',(22.6126741632309,2.03742874317627,15.));
#37634=CARTESIAN_POINT('Ctrl Pts',(22.5357303426251,2.07970095436224,15.));
#37635=CARTESIAN_POINT('Ctrl Pts',(22.4586506520939,2.1213521324248,15.));
#37636=CARTESIAN_POINT('Ctrl Pts',(22.3814381677224,2.16237755726404,15.));
#37637=CARTESIAN_POINT('Ctrl Pts',(22.3040959372933,2.20277263221399,15.));
#37638=CARTESIAN_POINT('Ctrl Pts',(22.2266269576315,2.24253288454712,15.));
#37639=CARTESIAN_POINT('Ctrl Pts',(22.1490342171802,2.28165375160231,15.));
#37640=CARTESIAN_POINT('Ctrl Pts',(22.0713207257413,2.32013040994125,15.));
#37641=CARTESIAN_POINT('Ctrl Pts',(21.9934895476958,2.35795761145761,15.));
#37642=CARTESIAN_POINT('Ctrl Pts',(21.9155438409279,2.39512947344577,15.));
#37643=CARTESIAN_POINT('Ctrl Pts',(21.8374868743435,2.43163944362692,15.));
#37644=CARTESIAN_POINT('Ctrl Pts',(21.7593219872847,2.46748070362075,15.));
#37645=CARTESIAN_POINT('Ctrl Pts',(21.6810525594039,2.50264651177235,15.));
#37646=CARTESIAN_POINT('Ctrl Pts',(21.6026819803014,2.53713053453766,15.));
#37647=CARTESIAN_POINT('Ctrl Pts',(21.5242136128466,2.5709272835198,15.));
#37648=CARTESIAN_POINT('Ctrl Pts',(21.4456507822983,2.60403221866523,15.));
#37649=CARTESIAN_POINT('Ctrl Pts',(21.3669968505594,2.6364407451853,15.));
#37650=CARTESIAN_POINT('Ctrl Pts',(21.2882552797978,2.668147357083,15.));
#37651=CARTESIAN_POINT('Ctrl Pts',(21.2094296949571,2.69914481283353,15.));
#37652=CARTESIAN_POINT('Ctrl Pts',(21.1305239619219,2.72942309852119,15.));
#37653=CARTESIAN_POINT('Ctrl Pts',(21.0515422162039,2.7589691000769,15.));
#37654=CARTESIAN_POINT('Ctrl Pts',(20.9724887103073,2.78776883747222,15.));
#37655=CARTESIAN_POINT('Ctrl Pts',(20.8933676828246,2.81580940715318,15.));
#37656=CARTESIAN_POINT('Ctrl Pts',(20.8141832346435,2.84308082507644,15.));
#37657=CARTESIAN_POINT('Ctrl Pts',(20.7349391669725,2.86957843933153,15.));
#37658=CARTESIAN_POINT('Ctrl Pts',(20.6556389450993,2.89530351700805,15.));
#37659=CARTESIAN_POINT('Ctrl Pts',(20.5762860772943,2.92025778619206,15.));
#37660=CARTESIAN_POINT('Ctrl Pts',(20.4968844460513,2.94443868035154,15.));
#37661=CARTESIAN_POINT('Ctrl Pts',(20.4174386170774,2.96783492132513,15.));
#37662=CARTESIAN_POINT('Ctrl Pts',(20.3379542578194,2.99042050197904,15.));
#37663=CARTESIAN_POINT('Ctrl Pts',(20.2584381977107,3.01215393913612,15.));
#37664=CARTESIAN_POINT('Ctrl Pts',(20.178897575607,3.03299094576288,15.));
#37665=CARTESIAN_POINT('Ctrl Pts',(20.0993390992966,3.05289545759951,15.));
#37666=CARTESIAN_POINT('Ctrl Pts',(20.0197683853426,3.07184950717982,15.));
#37667=CARTESIAN_POINT('Ctrl Pts',(19.9401889653541,3.08986795998319,15.));
#37668=CARTESIAN_POINT('Ctrl Pts',(19.8606024365399,3.10699659920993,15.));
#37669=CARTESIAN_POINT('Ctrl Pts',(19.7810105986827,3.1232813132398,15.));
#37670=CARTESIAN_POINT('Ctrl Pts',(19.7014173131304,3.13874131344865,15.));
#37671=CARTESIAN_POINT('Ctrl Pts',(19.6218301288731,3.15334580802458,15.));
#37672=CARTESIAN_POINT('Ctrl Pts',(19.5422628528517,3.16697679689294,15.));
#37673=CARTESIAN_POINT('Ctrl Pts',(19.4627345689632,3.17944412249754,15.));
#37674=CARTESIAN_POINT('Ctrl Pts',(19.3832648965708,3.19055618489382,15.));
#37675=CARTESIAN_POINT('Ctrl Pts',(19.3038697977783,3.2001820370274,15.));
#37676=CARTESIAN_POINT('Ctrl Pts',(19.2245581120423,3.2083040369031,15.));
#37677=CARTESIAN_POINT('Ctrl Pts',(19.1453253990185,3.21510704576117,15.));
#37678=CARTESIAN_POINT('Ctrl Pts',(19.0661599344864,3.22090173651085,15.));
#37679=CARTESIAN_POINT('Ctrl Pts',(18.987055820781,3.22595008773715,15.));
#37680=CARTESIAN_POINT('Ctrl Pts',(18.908024664264,3.23031169402939,15.));
#37681=CARTESIAN_POINT('Ctrl Pts',(18.8291062617862,3.23370091065669,15.));
#37682=CARTESIAN_POINT('Ctrl Pts',(18.7503838921122,3.23528809328097,15.));
#37683=CARTESIAN_POINT('Ctrl Pts',(18.6719665316945,3.23390622002644,15.));
#37684=CARTESIAN_POINT('Ctrl Pts',(18.6095634206219,3.2294700044416,15.));
#37685=CARTESIAN_POINT('Ctrl Pts',(18.5629852384321,3.22384302136592,15.));
#37686=CARTESIAN_POINT('Ctrl Pts',(18.5320375674878,3.2190148958593,15.));
#37687=CARTESIAN_POINT('Ctrl Pts',(18.5165898451125,3.2163316265074,15.));
#37688=CARTESIAN_POINT('',(16.1003491021971,2.79663061332403,15.));
#37689=CARTESIAN_POINT('',(15.135366975784,2.62901321950806,15.));
#37690=CARTESIAN_POINT('',(14.9562571344462,3.5508810918317,15.));
#37691=CARTESIAN_POINT('Origin',(15.9292116709051,3.78187778008512,15.));
#37692=CARTESIAN_POINT('Origin',(0.,0.,15.));
#37693=CARTESIAN_POINT('Origin',(0.,0.,15.));
#37694=CARTESIAN_POINT('Origin',(0.,0.,15.));
#37695=CARTESIAN_POINT('Origin',(0.,0.,15.));
#37696=CARTESIAN_POINT('Origin',(0.,0.,15.));
#37697=CARTESIAN_POINT('Origin',(0.,0.,15.));
#37698=CARTESIAN_POINT('Origin',(0.,0.,15.));
#37699=CARTESIAN_POINT('Origin',(0.,0.,15.));
#37700=CARTESIAN_POINT('Origin',(0.,0.,15.));
#37701=CARTESIAN_POINT('Origin',(0.,0.,0.));
#37702=CARTESIAN_POINT('',(14.9562571344462,3.5508810918317,0.));
#37703=CARTESIAN_POINT('Origin',(0.,0.,0.));
#37704=CARTESIAN_POINT('Origin',(0.,0.,0.));
#37705=CARTESIAN_POINT('Origin',(0.,0.,0.));
#37706=CARTESIAN_POINT('Origin',(0.,0.,0.));
#37707=CARTESIAN_POINT('Origin',(0.,0.,0.));
#37708=CARTESIAN_POINT('Origin',(0.,0.,0.));
#37709=CARTESIAN_POINT('Origin',(0.,0.,0.));
#37710=CARTESIAN_POINT('Origin',(0.,0.,0.));
#37711=CARTESIAN_POINT('Origin',(15.9292116709051,3.78187778008512,0.));
#37712=CARTESIAN_POINT('',(16.1003491021971,2.79663061332403,0.));
#37713=CARTESIAN_POINT('Origin',(18.5165898451125,3.2163316265074,0.));
#37714=CARTESIAN_POINT('',(18.5165898451125,3.2163316265074,0.));
#37715=CARTESIAN_POINT('Origin',(15.9292116709051,-3.78187778008512,0.));
#37716=CARTESIAN_POINT('',(16.1003491021971,-2.79663061332403,0.));
#37717=CARTESIAN_POINT('',(14.9562571344462,-3.5508810918317,0.));
#37718=CARTESIAN_POINT('Origin',(15.135366975784,-2.62901321950806,0.));
#37719=CARTESIAN_POINT('',(18.5165898451125,-3.2163316265074,0.));
#37720=CARTESIAN_POINT('Ctrl Pts',(23.9712218930251,1.17495572484832,0.));
#37721=CARTESIAN_POINT('Ctrl Pts',(23.9712218930251,1.17495572484832,18.));
#37722=CARTESIAN_POINT('Ctrl Pts',(23.9564318364582,1.18556439589232,0.));
#37723=CARTESIAN_POINT('Ctrl Pts',(23.9564318364582,1.18556439589232,18.));
#37724=CARTESIAN_POINT('Ctrl Pts',(23.9268340213744,1.20672599652272,0.));
#37725=CARTESIAN_POINT('Ctrl Pts',(23.9268340213744,1.20672599652272,18.));
#37726=CARTESIAN_POINT('Ctrl Pts',(23.8823841929226,1.2383011730893,0.));
#37727=CARTESIAN_POINT('Ctrl Pts',(23.8823841929226,1.2383011730893,18.));
#37728=CARTESIAN_POINT('Ctrl Pts',(23.8230115078373,1.28006684869166,0.));
#37729=CARTESIAN_POINT('Ctrl Pts',(23.8230115078373,1.28006684869166,18.));
#37730=CARTESIAN_POINT('Ctrl Pts',(23.748618507953,1.33171549586249,0.));
#37731=CARTESIAN_POINT('Ctrl Pts',(23.748618507953,1.33171549586249,18.));
#37732=CARTESIAN_POINT('Ctrl Pts',(23.6740485197917,1.38280426780156,0.));
#37733=CARTESIAN_POINT('Ctrl Pts',(23.6740485197917,1.38280426780156,18.));
#37734=CARTESIAN_POINT('Ctrl Pts',(23.5993021272808,1.4333311444639,0.));
#37735=CARTESIAN_POINT('Ctrl Pts',(23.5993021272808,1.4333311444639,18.));
#37736=CARTESIAN_POINT('Ctrl Pts',(23.5243805284282,1.48329351290851,0.));
#37737=CARTESIAN_POINT('Ctrl Pts',(23.5243805284282,1.48329351290851,18.));
#37738=CARTESIAN_POINT('Ctrl Pts',(23.4492857841673,1.53268814658653,0.));
#37739=CARTESIAN_POINT('Ctrl Pts',(23.4492857841673,1.53268814658653,18.));
#37740=CARTESIAN_POINT('Ctrl Pts',(23.3740206492924,1.58151133638847,0.));
#37741=CARTESIAN_POINT('Ctrl Pts',(23.3740206492924,1.58151133638847,18.));
#37742=CARTESIAN_POINT('Ctrl Pts',(23.2985883089733,1.62975905604583,0.));
#37743=CARTESIAN_POINT('Ctrl Pts',(23.2985883089733,1.62975905604583,18.));
#37744=CARTESIAN_POINT('Ctrl Pts',(23.2229921402299,1.67742712670823,0.));
#37745=CARTESIAN_POINT('Ctrl Pts',(23.2229921402299,1.67742712670823,18.));
#37746=CARTESIAN_POINT('Ctrl Pts',(23.1472354850579,1.72451136919382,0.));
#37747=CARTESIAN_POINT('Ctrl Pts',(23.1472354850579,1.72451136919382,18.));
#37748=CARTESIAN_POINT('Ctrl Pts',(23.0713213684573,1.77100780743078,0.));
#37749=CARTESIAN_POINT('Ctrl Pts',(23.0713213684573,1.77100780743078,18.));
#37750=CARTESIAN_POINT('Ctrl Pts',(22.9952524859917,1.81691265597281,0.));
#37751=CARTESIAN_POINT('Ctrl Pts',(22.9952524859917,1.81691265597281,18.));
#37752=CARTESIAN_POINT('Ctrl Pts',(22.9190313507225,1.86222218327819,0.));
#37753=CARTESIAN_POINT('Ctrl Pts',(22.9190313507225,1.86222218327819,18.));
#37754=CARTESIAN_POINT('Ctrl Pts',(22.8426603964871,1.90693261239855,0.));
#37755=CARTESIAN_POINT('Ctrl Pts',(22.8426603964871,1.90693261239855,18.));
#37756=CARTESIAN_POINT('Ctrl Pts',(22.7661420906702,1.95104002082891,0.));
#37757=CARTESIAN_POINT('Ctrl Pts',(22.7661420906702,1.95104002082891,18.));
#37758=CARTESIAN_POINT('Ctrl Pts',(22.6894790673923,1.99454021984253,0.));
#37759=CARTESIAN_POINT('Ctrl Pts',(22.6894790673923,1.99454021984253,18.));
#37760=CARTESIAN_POINT('Ctrl Pts',(22.6126741632309,2.03742874317627,0.));
#37761=CARTESIAN_POINT('Ctrl Pts',(22.6126741632309,2.03742874317627,18.));
#37762=CARTESIAN_POINT('Ctrl Pts',(22.5357303426251,2.07970095436224,0.));
#37763=CARTESIAN_POINT('Ctrl Pts',(22.5357303426251,2.07970095436224,18.));
#37764=CARTESIAN_POINT('Ctrl Pts',(22.4586506520939,2.1213521324248,0.));
#37765=CARTESIAN_POINT('Ctrl Pts',(22.4586506520939,2.1213521324248,18.));
#37766=CARTESIAN_POINT('Ctrl Pts',(22.3814381677224,2.16237755726404,0.));
#37767=CARTESIAN_POINT('Ctrl Pts',(22.3814381677224,2.16237755726404,18.));
#37768=CARTESIAN_POINT('Ctrl Pts',(22.3040959372933,2.20277263221399,0.));
#37769=CARTESIAN_POINT('Ctrl Pts',(22.3040959372933,2.20277263221399,18.));
#37770=CARTESIAN_POINT('Ctrl Pts',(22.2266269576315,2.24253288454712,0.));
#37771=CARTESIAN_POINT('Ctrl Pts',(22.2266269576315,2.24253288454712,18.));
#37772=CARTESIAN_POINT('Ctrl Pts',(22.1490342171802,2.28165375160231,0.));
#37773=CARTESIAN_POINT('Ctrl Pts',(22.1490342171802,2.28165375160231,18.));
#37774=CARTESIAN_POINT('Ctrl Pts',(22.0713207257413,2.32013040994125,0.));
#37775=CARTESIAN_POINT('Ctrl Pts',(22.0713207257413,2.32013040994125,18.));
#37776=CARTESIAN_POINT('Ctrl Pts',(21.9934895476958,2.35795761145761,0.));
#37777=CARTESIAN_POINT('Ctrl Pts',(21.9934895476958,2.35795761145761,18.));
#37778=CARTESIAN_POINT('Ctrl Pts',(21.9155438409279,2.39512947344577,0.));
#37779=CARTESIAN_POINT('Ctrl Pts',(21.9155438409279,2.39512947344577,18.));
#37780=CARTESIAN_POINT('Ctrl Pts',(21.8374868743435,2.43163944362692,0.));
#37781=CARTESIAN_POINT('Ctrl Pts',(21.8374868743435,2.43163944362692,18.));
#37782=CARTESIAN_POINT('Ctrl Pts',(21.7593219872847,2.46748070362075,0.));
#37783=CARTESIAN_POINT('Ctrl Pts',(21.7593219872847,2.46748070362075,18.));
#37784=CARTESIAN_POINT('Ctrl Pts',(21.6810525594039,2.50264651177235,0.));
#37785=CARTESIAN_POINT('Ctrl Pts',(21.6810525594039,2.50264651177235,18.));
#37786=CARTESIAN_POINT('Ctrl Pts',(21.6026819803014,2.53713053453766,0.));
#37787=CARTESIAN_POINT('Ctrl Pts',(21.6026819803014,2.53713053453766,18.));
#37788=CARTESIAN_POINT('Ctrl Pts',(21.5242136128466,2.5709272835198,0.));
#37789=CARTESIAN_POINT('Ctrl Pts',(21.5242136128466,2.5709272835198,18.));
#37790=CARTESIAN_POINT('Ctrl Pts',(21.4456507822983,2.60403221866523,0.));
#37791=CARTESIAN_POINT('Ctrl Pts',(21.4456507822983,2.60403221866523,18.));
#37792=CARTESIAN_POINT('Ctrl Pts',(21.3669968505594,2.6364407451853,0.));
#37793=CARTESIAN_POINT('Ctrl Pts',(21.3669968505594,2.6364407451853,18.));
#37794=CARTESIAN_POINT('Ctrl Pts',(21.2882552797978,2.668147357083,0.));
#37795=CARTESIAN_POINT('Ctrl Pts',(21.2882552797978,2.668147357083,18.));
#37796=CARTESIAN_POINT('Ctrl Pts',(21.2094296949571,2.69914481283353,0.));
#37797=CARTESIAN_POINT('Ctrl Pts',(21.2094296949571,2.69914481283353,18.));
#37798=CARTESIAN_POINT('Ctrl Pts',(21.1305239619219,2.72942309852119,0.));
#37799=CARTESIAN_POINT('Ctrl Pts',(21.1305239619219,2.72942309852119,18.));
#37800=CARTESIAN_POINT('Ctrl Pts',(21.0515422162039,2.7589691000769,0.));
#37801=CARTESIAN_POINT('Ctrl Pts',(21.0515422162039,2.7589691000769,18.));
#37802=CARTESIAN_POINT('Ctrl Pts',(20.9724887103073,2.78776883747222,0.));
#37803=CARTESIAN_POINT('Ctrl Pts',(20.9724887103073,2.78776883747222,18.));
#37804=CARTESIAN_POINT('Ctrl Pts',(20.8933676828246,2.81580940715318,0.));
#37805=CARTESIAN_POINT('Ctrl Pts',(20.8933676828246,2.81580940715318,18.));
#37806=CARTESIAN_POINT('Ctrl Pts',(20.8141832346435,2.84308082507644,0.));
#37807=CARTESIAN_POINT('Ctrl Pts',(20.8141832346435,2.84308082507644,18.));
#37808=CARTESIAN_POINT('Ctrl Pts',(20.7349391669725,2.86957843933153,0.));
#37809=CARTESIAN_POINT('Ctrl Pts',(20.7349391669725,2.86957843933153,18.));
#37810=CARTESIAN_POINT('Ctrl Pts',(20.6556389450993,2.89530351700805,0.));
#37811=CARTESIAN_POINT('Ctrl Pts',(20.6556389450993,2.89530351700805,18.));
#37812=CARTESIAN_POINT('Ctrl Pts',(20.5762860772943,2.92025778619206,0.));
#37813=CARTESIAN_POINT('Ctrl Pts',(20.5762860772943,2.92025778619206,18.));
#37814=CARTESIAN_POINT('Ctrl Pts',(20.4968844460513,2.94443868035154,0.));
#37815=CARTESIAN_POINT('Ctrl Pts',(20.4968844460513,2.94443868035154,18.));
#37816=CARTESIAN_POINT('Ctrl Pts',(20.4174386170774,2.96783492132513,0.));
#37817=CARTESIAN_POINT('Ctrl Pts',(20.4174386170774,2.96783492132513,18.));
#37818=CARTESIAN_POINT('Ctrl Pts',(20.3379542578194,2.99042050197904,0.));
#37819=CARTESIAN_POINT('Ctrl Pts',(20.3379542578194,2.99042050197904,18.));
#37820=CARTESIAN_POINT('Ctrl Pts',(20.2584381977107,3.01215393913612,0.));
#37821=CARTESIAN_POINT('Ctrl Pts',(20.2584381977107,3.01215393913612,18.));
#37822=CARTESIAN_POINT('Ctrl Pts',(20.178897575607,3.03299094576288,0.));
#37823=CARTESIAN_POINT('Ctrl Pts',(20.178897575607,3.03299094576288,18.));
#37824=CARTESIAN_POINT('Ctrl Pts',(20.0993390992966,3.05289545759951,0.));
#37825=CARTESIAN_POINT('Ctrl Pts',(20.0993390992966,3.05289545759951,18.));
#37826=CARTESIAN_POINT('Ctrl Pts',(20.0197683853426,3.07184950717982,0.));
#37827=CARTESIAN_POINT('Ctrl Pts',(20.0197683853426,3.07184950717982,18.));
#37828=CARTESIAN_POINT('Ctrl Pts',(19.9401889653541,3.08986795998319,0.));
#37829=CARTESIAN_POINT('Ctrl Pts',(19.9401889653541,3.08986795998319,18.));
#37830=CARTESIAN_POINT('Ctrl Pts',(19.8606024365399,3.10699659920993,0.));
#37831=CARTESIAN_POINT('Ctrl Pts',(19.8606024365399,3.10699659920993,18.));
#37832=CARTESIAN_POINT('Ctrl Pts',(19.7810105986827,3.1232813132398,0.));
#37833=CARTESIAN_POINT('Ctrl Pts',(19.7810105986827,3.1232813132398,18.));
#37834=CARTESIAN_POINT('Ctrl Pts',(19.7014173131304,3.13874131344865,0.));
#37835=CARTESIAN_POINT('Ctrl Pts',(19.7014173131304,3.13874131344865,18.));
#37836=CARTESIAN_POINT('Ctrl Pts',(19.6218301288731,3.15334580802458,0.));
#37837=CARTESIAN_POINT('Ctrl Pts',(19.6218301288731,3.15334580802458,18.));
#37838=CARTESIAN_POINT('Ctrl Pts',(19.5422628528517,3.16697679689294,0.));
#37839=CARTESIAN_POINT('Ctrl Pts',(19.5422628528517,3.16697679689294,18.));
#37840=CARTESIAN_POINT('Ctrl Pts',(19.4627345689632,3.17944412249754,0.));
#37841=CARTESIAN_POINT('Ctrl Pts',(19.4627345689632,3.17944412249754,18.));
#37842=CARTESIAN_POINT('Ctrl Pts',(19.3832648965708,3.19055618489382,0.));
#37843=CARTESIAN_POINT('Ctrl Pts',(19.3832648965708,3.19055618489382,18.));
#37844=CARTESIAN_POINT('Ctrl Pts',(19.3038697977783,3.2001820370274,0.));
#37845=CARTESIAN_POINT('Ctrl Pts',(19.3038697977783,3.2001820370274,18.));
#37846=CARTESIAN_POINT('Ctrl Pts',(19.2245581120423,3.2083040369031,0.));
#37847=CARTESIAN_POINT('Ctrl Pts',(19.2245581120423,3.2083040369031,18.));
#37848=CARTESIAN_POINT('Ctrl Pts',(19.1453253990185,3.21510704576117,0.));
#37849=CARTESIAN_POINT('Ctrl Pts',(19.1453253990185,3.21510704576117,18.));
#37850=CARTESIAN_POINT('Ctrl Pts',(19.0661599344864,3.22090173651085,0.));
#37851=CARTESIAN_POINT('Ctrl Pts',(19.0661599344864,3.22090173651085,18.));
#37852=CARTESIAN_POINT('Ctrl Pts',(18.987055820781,3.22595008773715,0.));
#37853=CARTESIAN_POINT('Ctrl Pts',(18.987055820781,3.22595008773715,18.));
#37854=CARTESIAN_POINT('Ctrl Pts',(18.908024664264,3.23031169402939,0.));
#37855=CARTESIAN_POINT('Ctrl Pts',(18.908024664264,3.23031169402939,18.));
#37856=CARTESIAN_POINT('Ctrl Pts',(18.8291062617862,3.23370091065669,0.));
#37857=CARTESIAN_POINT('Ctrl Pts',(18.8291062617862,3.23370091065669,18.));
#37858=CARTESIAN_POINT('Ctrl Pts',(18.7503838921122,3.23528809328097,0.));
#37859=CARTESIAN_POINT('Ctrl Pts',(18.7503838921122,3.23528809328097,18.));
#37860=CARTESIAN_POINT('Ctrl Pts',(18.6719665316945,3.23390622002644,0.));
#37861=CARTESIAN_POINT('Ctrl Pts',(18.6719665316945,3.23390622002644,18.));
#37862=CARTESIAN_POINT('Ctrl Pts',(18.6095634206219,3.2294700044416,0.));
#37863=CARTESIAN_POINT('Ctrl Pts',(18.6095634206219,3.2294700044416,18.));
#37864=CARTESIAN_POINT('Ctrl Pts',(18.5629852384321,3.22384302136592,0.));
#37865=CARTESIAN_POINT('Ctrl Pts',(18.5629852384321,3.22384302136592,18.));
#37866=CARTESIAN_POINT('Ctrl Pts',(18.5320375674878,3.2190148958593,0.));
#37867=CARTESIAN_POINT('Ctrl Pts',(18.5320375674878,3.2190148958593,18.));
#37868=CARTESIAN_POINT('Ctrl Pts',(18.5165898451125,3.2163316265074,0.));
#37869=CARTESIAN_POINT('Ctrl Pts',(18.5165898451125,3.2163316265074,18.));
#37870=CARTESIAN_POINT('',(23.9712218930251,1.17495572484827,0.));
#37871=CARTESIAN_POINT('Origin',(1.15463194561016E-13,-6.93889390390723E-17,
0.));
#37872=CARTESIAN_POINT('',(23.9712218930251,-1.17495572484832,0.));
#37873=CARTESIAN_POINT('Ctrl Pts',(18.5165898451125,-3.2163316265074,0.));
#37874=CARTESIAN_POINT('Ctrl Pts',(18.5165898451125,-3.2163316265074,18.));
#37875=CARTESIAN_POINT('Ctrl Pts',(18.5320375674878,-3.2190148958593,0.));
#37876=CARTESIAN_POINT('Ctrl Pts',(18.5320375674878,-3.2190148958593,18.));
#37877=CARTESIAN_POINT('Ctrl Pts',(18.5629852384321,-3.22384302136592,0.));
#37878=CARTESIAN_POINT('Ctrl Pts',(18.5629852384321,-3.22384302136592,18.));
#37879=CARTESIAN_POINT('Ctrl Pts',(18.6095634206219,-3.2294700044416,0.));
#37880=CARTESIAN_POINT('Ctrl Pts',(18.6095634206219,-3.2294700044416,18.));
#37881=CARTESIAN_POINT('Ctrl Pts',(18.6719665316945,-3.23390622002644,0.));
#37882=CARTESIAN_POINT('Ctrl Pts',(18.6719665316945,-3.23390622002644,18.));
#37883=CARTESIAN_POINT('Ctrl Pts',(18.7503838921122,-3.23528809328097,0.));
#37884=CARTESIAN_POINT('Ctrl Pts',(18.7503838921122,-3.23528809328097,18.));
#37885=CARTESIAN_POINT('Ctrl Pts',(18.8291062617862,-3.23370091065669,0.));
#37886=CARTESIAN_POINT('Ctrl Pts',(18.8291062617862,-3.23370091065669,18.));
#37887=CARTESIAN_POINT('Ctrl Pts',(18.908024664264,-3.23031169402939,0.));
#37888=CARTESIAN_POINT('Ctrl Pts',(18.908024664264,-3.23031169402939,18.));
#37889=CARTESIAN_POINT('Ctrl Pts',(18.987055820781,-3.22595008773715,0.));
#37890=CARTESIAN_POINT('Ctrl Pts',(18.987055820781,-3.22595008773715,18.));
#37891=CARTESIAN_POINT('Ctrl Pts',(19.0661599344864,-3.22090173651085,0.));
#37892=CARTESIAN_POINT('Ctrl Pts',(19.0661599344864,-3.22090173651085,18.));
#37893=CARTESIAN_POINT('Ctrl Pts',(19.1453253990185,-3.21510704576117,0.));
#37894=CARTESIAN_POINT('Ctrl Pts',(19.1453253990185,-3.21510704576117,18.));
#37895=CARTESIAN_POINT('Ctrl Pts',(19.2245581120423,-3.2083040369031,0.));
#37896=CARTESIAN_POINT('Ctrl Pts',(19.2245581120423,-3.2083040369031,18.));
#37897=CARTESIAN_POINT('Ctrl Pts',(19.3038697977783,-3.2001820370274,0.));
#37898=CARTESIAN_POINT('Ctrl Pts',(19.3038697977783,-3.2001820370274,18.));
#37899=CARTESIAN_POINT('Ctrl Pts',(19.3832648965708,-3.19055618489382,0.));
#37900=CARTESIAN_POINT('Ctrl Pts',(19.3832648965708,-3.19055618489382,18.));
#37901=CARTESIAN_POINT('Ctrl Pts',(19.4627345689632,-3.17944412249754,0.));
#37902=CARTESIAN_POINT('Ctrl Pts',(19.4627345689632,-3.17944412249754,18.));
#37903=CARTESIAN_POINT('Ctrl Pts',(19.5422628528517,-3.16697679689294,0.));
#37904=CARTESIAN_POINT('Ctrl Pts',(19.5422628528517,-3.16697679689294,18.));
#37905=CARTESIAN_POINT('Ctrl Pts',(19.6218301288731,-3.15334580802458,0.));
#37906=CARTESIAN_POINT('Ctrl Pts',(19.6218301288731,-3.15334580802458,18.));
#37907=CARTESIAN_POINT('Ctrl Pts',(19.7014173131304,-3.13874131344865,0.));
#37908=CARTESIAN_POINT('Ctrl Pts',(19.7014173131304,-3.13874131344865,18.));
#37909=CARTESIAN_POINT('Ctrl Pts',(19.7810105986827,-3.1232813132398,0.));
#37910=CARTESIAN_POINT('Ctrl Pts',(19.7810105986827,-3.1232813132398,18.));
#37911=CARTESIAN_POINT('Ctrl Pts',(19.8606024365399,-3.10699659920993,0.));
#37912=CARTESIAN_POINT('Ctrl Pts',(19.8606024365399,-3.10699659920993,18.));
#37913=CARTESIAN_POINT('Ctrl Pts',(19.9401889653541,-3.08986795998319,0.));
#37914=CARTESIAN_POINT('Ctrl Pts',(19.9401889653541,-3.08986795998319,18.));
#37915=CARTESIAN_POINT('Ctrl Pts',(20.0197683853426,-3.07184950717982,0.));
#37916=CARTESIAN_POINT('Ctrl Pts',(20.0197683853426,-3.07184950717982,18.));
#37917=CARTESIAN_POINT('Ctrl Pts',(20.0993390992966,-3.05289545759951,0.));
#37918=CARTESIAN_POINT('Ctrl Pts',(20.0993390992966,-3.05289545759951,18.));
#37919=CARTESIAN_POINT('Ctrl Pts',(20.178897575607,-3.03299094576288,0.));
#37920=CARTESIAN_POINT('Ctrl Pts',(20.178897575607,-3.03299094576288,18.));
#37921=CARTESIAN_POINT('Ctrl Pts',(20.2584381977107,-3.01215393913612,0.));
#37922=CARTESIAN_POINT('Ctrl Pts',(20.2584381977107,-3.01215393913612,18.));
#37923=CARTESIAN_POINT('Ctrl Pts',(20.3379542578194,-2.99042050197904,0.));
#37924=CARTESIAN_POINT('Ctrl Pts',(20.3379542578194,-2.99042050197904,18.));
#37925=CARTESIAN_POINT('Ctrl Pts',(20.4174386170774,-2.96783492132513,0.));
#37926=CARTESIAN_POINT('Ctrl Pts',(20.4174386170774,-2.96783492132513,18.));
#37927=CARTESIAN_POINT('Ctrl Pts',(20.4968844460513,-2.94443868035154,0.));
#37928=CARTESIAN_POINT('Ctrl Pts',(20.4968844460513,-2.94443868035154,18.));
#37929=CARTESIAN_POINT('Ctrl Pts',(20.5762860772943,-2.92025778619206,0.));
#37930=CARTESIAN_POINT('Ctrl Pts',(20.5762860772943,-2.92025778619206,18.));
#37931=CARTESIAN_POINT('Ctrl Pts',(20.6556389450993,-2.89530351700805,0.));
#37932=CARTESIAN_POINT('Ctrl Pts',(20.6556389450993,-2.89530351700805,18.));
#37933=CARTESIAN_POINT('Ctrl Pts',(20.7349391669725,-2.86957843933153,0.));
#37934=CARTESIAN_POINT('Ctrl Pts',(20.7349391669725,-2.86957843933153,18.));
#37935=CARTESIAN_POINT('Ctrl Pts',(20.8141832346435,-2.84308082507644,0.));
#37936=CARTESIAN_POINT('Ctrl Pts',(20.8141832346435,-2.84308082507644,18.));
#37937=CARTESIAN_POINT('Ctrl Pts',(20.8933676828246,-2.81580940715318,0.));
#37938=CARTESIAN_POINT('Ctrl Pts',(20.8933676828246,-2.81580940715318,18.));
#37939=CARTESIAN_POINT('Ctrl Pts',(20.9724887103073,-2.78776883747222,0.));
#37940=CARTESIAN_POINT('Ctrl Pts',(20.9724887103073,-2.78776883747222,18.));
#37941=CARTESIAN_POINT('Ctrl Pts',(21.0515422162039,-2.7589691000769,0.));
#37942=CARTESIAN_POINT('Ctrl Pts',(21.0515422162039,-2.7589691000769,18.));
#37943=CARTESIAN_POINT('Ctrl Pts',(21.1305239619219,-2.72942309852119,0.));
#37944=CARTESIAN_POINT('Ctrl Pts',(21.1305239619219,-2.72942309852119,18.));
#37945=CARTESIAN_POINT('Ctrl Pts',(21.2094296949571,-2.69914481283353,0.));
#37946=CARTESIAN_POINT('Ctrl Pts',(21.2094296949571,-2.69914481283353,18.));
#37947=CARTESIAN_POINT('Ctrl Pts',(21.2882552797978,-2.668147357083,0.));
#37948=CARTESIAN_POINT('Ctrl Pts',(21.2882552797978,-2.668147357083,18.));
#37949=CARTESIAN_POINT('Ctrl Pts',(21.3669968505594,-2.6364407451853,0.));
#37950=CARTESIAN_POINT('Ctrl Pts',(21.3669968505594,-2.6364407451853,18.));
#37951=CARTESIAN_POINT('Ctrl Pts',(21.4456507822983,-2.60403221866523,0.));
#37952=CARTESIAN_POINT('Ctrl Pts',(21.4456507822983,-2.60403221866523,18.));
#37953=CARTESIAN_POINT('Ctrl Pts',(21.5242136128466,-2.5709272835198,0.));
#37954=CARTESIAN_POINT('Ctrl Pts',(21.5242136128466,-2.5709272835198,18.));
#37955=CARTESIAN_POINT('Ctrl Pts',(21.6026819803014,-2.53713053453766,0.));
#37956=CARTESIAN_POINT('Ctrl Pts',(21.6026819803014,-2.53713053453766,18.));
#37957=CARTESIAN_POINT('Ctrl Pts',(21.6810525594039,-2.50264651177235,0.));
#37958=CARTESIAN_POINT('Ctrl Pts',(21.6810525594039,-2.50264651177235,18.));
#37959=CARTESIAN_POINT('Ctrl Pts',(21.7593219872847,-2.46748070362075,0.));
#37960=CARTESIAN_POINT('Ctrl Pts',(21.7593219872847,-2.46748070362075,18.));
#37961=CARTESIAN_POINT('Ctrl Pts',(21.8374868743435,-2.43163944362692,0.));
#37962=CARTESIAN_POINT('Ctrl Pts',(21.8374868743435,-2.43163944362692,18.));
#37963=CARTESIAN_POINT('Ctrl Pts',(21.9155438409279,-2.39512947344577,0.));
#37964=CARTESIAN_POINT('Ctrl Pts',(21.9155438409279,-2.39512947344577,18.));
#37965=CARTESIAN_POINT('Ctrl Pts',(21.9934895476958,-2.35795761145761,0.));
#37966=CARTESIAN_POINT('Ctrl Pts',(21.9934895476958,-2.35795761145761,18.));
#37967=CARTESIAN_POINT('Ctrl Pts',(22.0713207257413,-2.32013040994125,0.));
#37968=CARTESIAN_POINT('Ctrl Pts',(22.0713207257413,-2.32013040994125,18.));
#37969=CARTESIAN_POINT('Ctrl Pts',(22.1490342171802,-2.28165375160231,0.));
#37970=CARTESIAN_POINT('Ctrl Pts',(22.1490342171802,-2.28165375160231,18.));
#37971=CARTESIAN_POINT('Ctrl Pts',(22.2266269576315,-2.24253288454712,0.));
#37972=CARTESIAN_POINT('Ctrl Pts',(22.2266269576315,-2.24253288454712,18.));
#37973=CARTESIAN_POINT('Ctrl Pts',(22.3040959372933,-2.20277263221399,0.));
#37974=CARTESIAN_POINT('Ctrl Pts',(22.3040959372933,-2.20277263221399,18.));
#37975=CARTESIAN_POINT('Ctrl Pts',(22.3814381677224,-2.16237755726404,0.));
#37976=CARTESIAN_POINT('Ctrl Pts',(22.3814381677224,-2.16237755726404,18.));
#37977=CARTESIAN_POINT('Ctrl Pts',(22.4586506520939,-2.1213521324248,0.));
#37978=CARTESIAN_POINT('Ctrl Pts',(22.4586506520939,-2.1213521324248,18.));
#37979=CARTESIAN_POINT('Ctrl Pts',(22.5357303426251,-2.07970095436224,0.));
#37980=CARTESIAN_POINT('Ctrl Pts',(22.5357303426251,-2.07970095436224,18.));
#37981=CARTESIAN_POINT('Ctrl Pts',(22.6126741632309,-2.03742874317627,0.));
#37982=CARTESIAN_POINT('Ctrl Pts',(22.6126741632309,-2.03742874317627,18.));
#37983=CARTESIAN_POINT('Ctrl Pts',(22.6894790673923,-1.99454021984253,0.));
#37984=CARTESIAN_POINT('Ctrl Pts',(22.6894790673923,-1.99454021984253,18.));
#37985=CARTESIAN_POINT('Ctrl Pts',(22.7661420906702,-1.95104002082891,0.));
#37986=CARTESIAN_POINT('Ctrl Pts',(22.7661420906702,-1.95104002082891,18.));
#37987=CARTESIAN_POINT('Ctrl Pts',(22.8426603964871,-1.90693261239855,0.));
#37988=CARTESIAN_POINT('Ctrl Pts',(22.8426603964871,-1.90693261239855,18.));
#37989=CARTESIAN_POINT('Ctrl Pts',(22.9190313507225,-1.86222218327819,0.));
#37990=CARTESIAN_POINT('Ctrl Pts',(22.9190313507225,-1.86222218327819,18.));
#37991=CARTESIAN_POINT('Ctrl Pts',(22.9952524859917,-1.81691265597281,0.));
#37992=CARTESIAN_POINT('Ctrl Pts',(22.9952524859917,-1.81691265597281,18.));
#37993=CARTESIAN_POINT('Ctrl Pts',(23.0713213684573,-1.77100780743078,0.));
#37994=CARTESIAN_POINT('Ctrl Pts',(23.0713213684573,-1.77100780743078,18.));
#37995=CARTESIAN_POINT('Ctrl Pts',(23.1472354850579,-1.72451136919382,0.));
#37996=CARTESIAN_POINT('Ctrl Pts',(23.1472354850579,-1.72451136919382,18.));
#37997=CARTESIAN_POINT('Ctrl Pts',(23.2229921402299,-1.67742712670823,0.));
#37998=CARTESIAN_POINT('Ctrl Pts',(23.2229921402299,-1.67742712670823,18.));
#37999=CARTESIAN_POINT('Ctrl Pts',(23.2985883089733,-1.62975905604583,0.));
#38000=CARTESIAN_POINT('Ctrl Pts',(23.2985883089733,-1.62975905604583,18.));
#38001=CARTESIAN_POINT('Ctrl Pts',(23.3740206492924,-1.58151133638847,0.));
#38002=CARTESIAN_POINT('Ctrl Pts',(23.3740206492924,-1.58151133638847,18.));
#38003=CARTESIAN_POINT('Ctrl Pts',(23.4492857841673,-1.53268814658653,0.));
#38004=CARTESIAN_POINT('Ctrl Pts',(23.4492857841673,-1.53268814658653,18.));
#38005=CARTESIAN_POINT('Ctrl Pts',(23.5243805284282,-1.48329351290851,0.));
#38006=CARTESIAN_POINT('Ctrl Pts',(23.5243805284282,-1.48329351290851,18.));
#38007=CARTESIAN_POINT('Ctrl Pts',(23.5993021272808,-1.4333311444639,0.));
#38008=CARTESIAN_POINT('Ctrl Pts',(23.5993021272808,-1.4333311444639,18.));
#38009=CARTESIAN_POINT('Ctrl Pts',(23.6740485197917,-1.38280426780156,0.));
#38010=CARTESIAN_POINT('Ctrl Pts',(23.6740485197917,-1.38280426780156,18.));
#38011=CARTESIAN_POINT('Ctrl Pts',(23.748618507953,-1.33171549586249,0.));
#38012=CARTESIAN_POINT('Ctrl Pts',(23.748618507953,-1.33171549586249,18.));
#38013=CARTESIAN_POINT('Ctrl Pts',(23.8230115078373,-1.28006684869166,0.));
#38014=CARTESIAN_POINT('Ctrl Pts',(23.8230115078373,-1.28006684869166,18.));
#38015=CARTESIAN_POINT('Ctrl Pts',(23.8823841929226,-1.2383011730893,0.));
#38016=CARTESIAN_POINT('Ctrl Pts',(23.8823841929226,-1.2383011730893,18.));
#38017=CARTESIAN_POINT('Ctrl Pts',(23.9268340213744,-1.20672599652272,0.));
#38018=CARTESIAN_POINT('Ctrl Pts',(23.9268340213744,-1.20672599652272,18.));
#38019=CARTESIAN_POINT('Ctrl Pts',(23.9564318364582,-1.18556439589232,0.));
#38020=CARTESIAN_POINT('Ctrl Pts',(23.9564318364582,-1.18556439589232,18.));
#38021=CARTESIAN_POINT('Ctrl Pts',(23.9712218930251,-1.17495572484832,0.));
#38022=CARTESIAN_POINT('Ctrl Pts',(23.9712218930251,-1.17495572484832,18.));
#38023=CARTESIAN_POINT('Origin',(0.,0.,0.));
#43764=UNCERTAINTY_MEASURE_WITH_UNIT(LENGTH_MEASURE(0.01),#43782,
'DISTANCE_ACCURACY_VALUE',
'Maximum model space distance between geometric entities at asserted c
onnectivities');
#43771=UNCERTAINTY_MEASURE_WITH_UNIT(LENGTH_MEASURE(0.01),#43782,
'DISTANCE_ACCURACY_VALUE',
'Maximum model space distance between geometric entities at asserted c
onnectivities');
#43774=(
GEOMETRIC_REPRESENTATION_CONTEXT(3)
GLOBAL_UNCERTAINTY_ASSIGNED_CONTEXT((#43764))
GLOBAL_UNIT_ASSIGNED_CONTEXT((#43782,#43784,#43785))
REPRESENTATION_CONTEXT('','3D')
);
#43781=(
GEOMETRIC_REPRESENTATION_CONTEXT(3)
GLOBAL_UNCERTAINTY_ASSIGNED_CONTEXT((#43771))
GLOBAL_UNIT_ASSIGNED_CONTEXT((#43782,#43784,#43785))
REPRESENTATION_CONTEXT('','3D')
);
#43782=(
LENGTH_UNIT()
NAMED_UNIT(*)
SI_UNIT(.MILLI.,.METRE.)
);
#43784=(
NAMED_UNIT(*)
PLANE_ANGLE_UNIT()
SI_UNIT($,.RADIAN.)
);
#43785=(
NAMED_UNIT(*)
SI_UNIT($,.STERADIAN.)
SOLID_ANGLE_UNIT()
);
#43788=SHAPE_DEFINITION_REPRESENTATION(#43797,#43814);
#43797=PRODUCT_DEFINITION_SHAPE('',$,#43824);
#43814=SHAPE_REPRESENTATION('',(#13476),#43774);
#43821=PRODUCT_DEFINITION_CONTEXT('part definition',#43850,'design');
#43824=PRODUCT_DEFINITION('Spur Gear 10 teeth','Spur Gear 10 teeth',#43833,
#43821);
#43833=PRODUCT_DEFINITION_FORMATION('',$,#43854);
#43850=APPLICATION_CONTEXT(
'Core Data for Automotive Mechanical Design Process');
#43851=PRODUCT_CONTEXT('part definition',#43850,'mechanical');
#43854=PRODUCT('Spur Gear 10 teeth','Spur Gear 10 teeth',
'Spur Gear; Module: 4.0; Num Teeth: 10; Pressure Angle: 20.0; Backlash
: 0.00 mm',(#43851));
#43862=PRESENTATION_STYLE_ASSIGNMENT((#43865));
#43865=SURFACE_STYLE_USAGE(.BOTH.,#43868);
#43868=SURFACE_SIDE_STYLE('',(#43871));
#43871=SURFACE_STYLE_FILL_AREA(#43874);
#43874=FILL_AREA_STYLE('Opaque(203,203,203)',(#43877));
#43877=FILL_AREA_STYLE_COLOUR('Opaque(203,203,203)',#43880);
#43880=COLOUR_RGB('Opaque(203,203,203)', 0.09019608, 0.27058824, 0.51372549);
ENDSEC;
END-ISO-10303-21;
